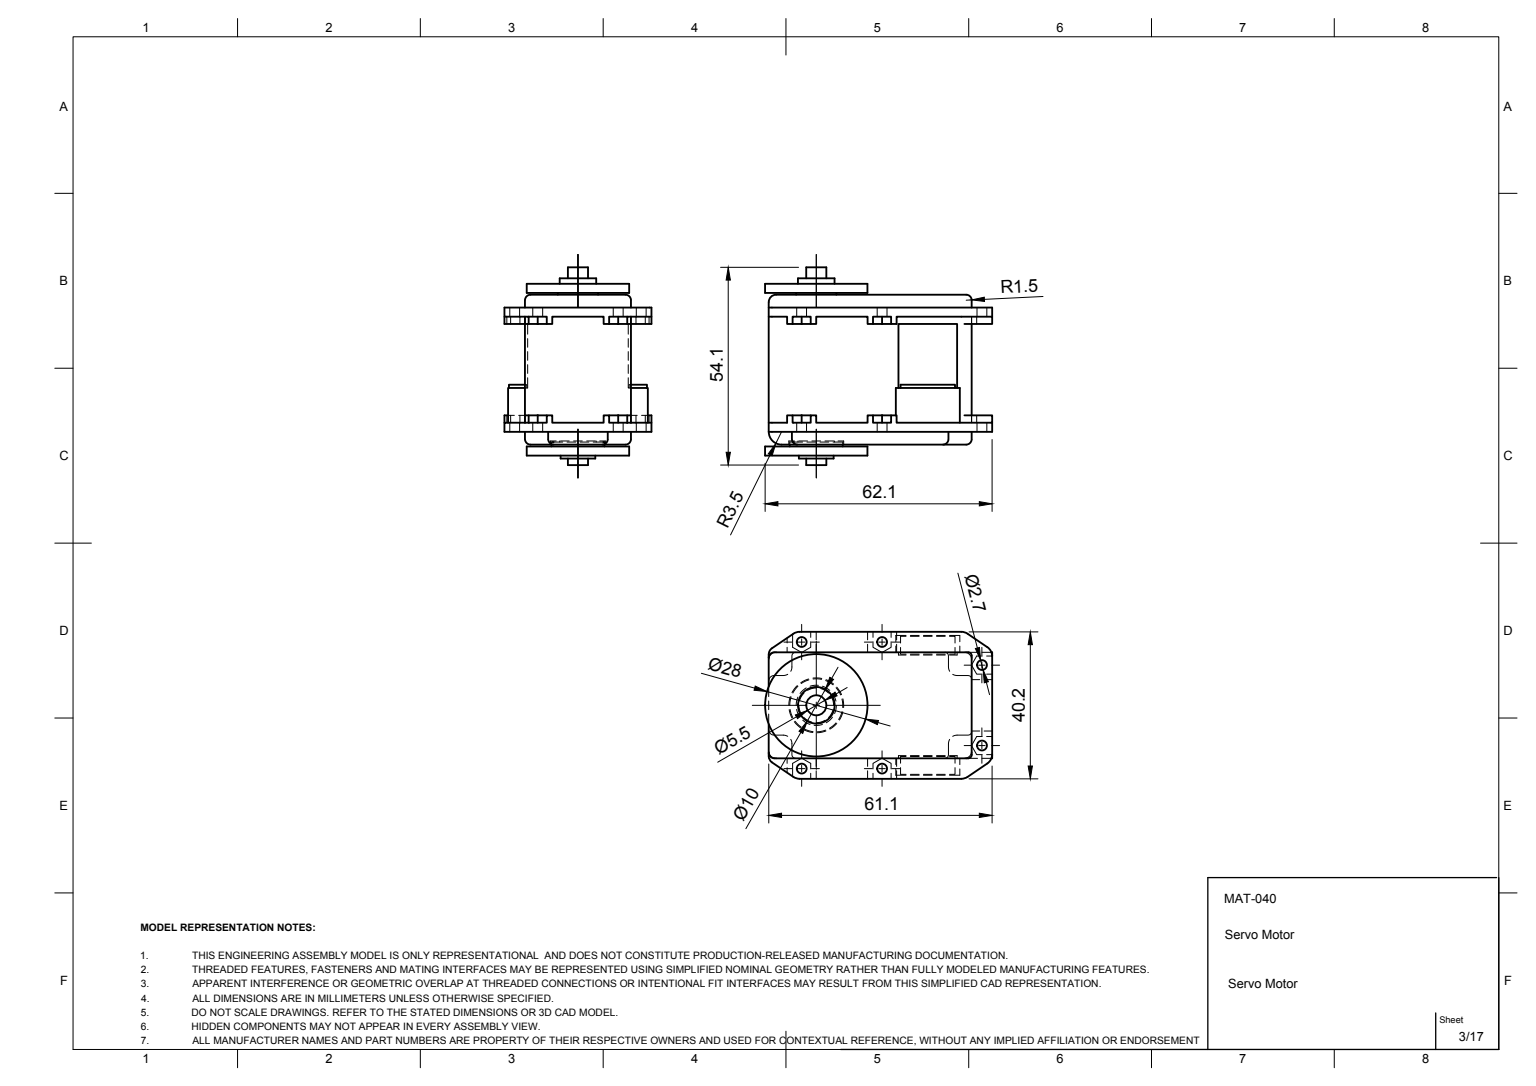
ISO-10303-21;
HEADER;
/* Generated by software containing ST-Developer
 * from STEP Tools, Inc. (www.steptools.com) 
 */

FILE_DESCRIPTION(
/* description */ ('STEP AP214'),
/* implementation_level */ '2;1');

FILE_NAME(
/* name */ 'Servo Motor.step',
/* time_stamp */ '2026-11-14T21:53:28-08:00',
/* author */ (''),
/* organization */ (''),
/* preprocessor_version */ 'ST-DEVELOPER v20.2',
/* originating_system */ 'Autodesk Translation Framework v15.17.0.0',
/* authorisation */ '');

FILE_SCHEMA (('AUTOMOTIVE_DESIGN { 1 0 10303 214 3 1 1 }'));
ENDSEC;

DATA;
#10=MECHANICAL_DESIGN_GEOMETRIC_PRESENTATION_REPRESENTATION('',(#319),#20176);
#223=TOROIDAL_SURFACE('',#11390,2.00000000000006,1.49999999999999);
#224=TOROIDAL_SURFACE('',#11425,1.99999999999991,1.5);
#225=TOROIDAL_SURFACE('',#11523,3.85000000000003,1.50000000000001);
#226=TOROIDAL_SURFACE('',#11533,3.85000000000009,1.50000000000001);
#227=TOROIDAL_SURFACE('',#11543,3.85,1.5);
#228=TOROIDAL_SURFACE('',#11553,3.84999999999996,1.49999999999999);
#232=B_SPLINE_SURFACE_WITH_KNOTS('',3,3,((#16443,#16444,#16445,#16446),
(#16447,#16448,#16449,#16450),(#16451,#16452,#16453,#16454),(#16455,#16456,
#16457,#16458),(#16459,#16460,#16461,#16462),(#16463,#16464,#16465,#16466),
(#16467,#16468,#16469,#16470),(#16471,#16472,#16473,#16474),(#16475,#16476,
#16477,#16478),(#16479,#16480,#16481,#16482),(#16483,#16484,#16485,#16486)),
 .UNSPECIFIED.,.F.,.F.,.F.,(4,1,1,1,1,1,1,1,4),(4,4),(-1.345105E-12,0.125,
0.25,0.375,0.5,0.625,0.75,0.875,0.999999999999432),(-0.007830111379204,
1.00000000177778),.UNSPECIFIED.);
#233=B_SPLINE_SURFACE_WITH_KNOTS('',3,3,((#16489,#16490,#16491,#16492),
(#16493,#16494,#16495,#16496),(#16497,#16498,#16499,#16500),(#16501,#16502,
#16503,#16504),(#16505,#16506,#16507,#16508),(#16509,#16510,#16511,#16512),
(#16513,#16514,#16515,#16516),(#16517,#16518,#16519,#16520),(#16521,#16522,
#16523,#16524),(#16525,#16526,#16527,#16528),(#16529,#16530,#16531,#16532)),
 .UNSPECIFIED.,.F.,.F.,.F.,(4,1,1,1,1,1,1,1,4),(4,4),(-0.000181680414011076,
0.125,0.25,0.375,0.5,0.625,0.75,0.875,1.00018168041298),(-0.007830111378265,
1.00000000177562),.UNSPECIFIED.);
#234=B_SPLINE_SURFACE_WITH_KNOTS('',3,3,((#18463,#18464,#18465,#18466),
(#18467,#18468,#18469,#18470),(#18471,#18472,#18473,#18474),(#18475,#18476,
#18477,#18478),(#18479,#18480,#18481,#18482),(#18483,#18484,#18485,#18486),
(#18487,#18488,#18489,#18490),(#18491,#18492,#18493,#18494),(#18495,#18496,
#18497,#18498),(#18499,#18500,#18501,#18502),(#18503,#18504,#18505,#18506)),
 .UNSPECIFIED.,.F.,.F.,.F.,(4,1,1,1,1,1,1,1,4),(4,4),(-0.000181679232336337,
0.125,0.25,0.375,0.5,0.625,0.75,0.875,1.00018167923146),(-0.007830111378221,
1.00000000177564),.UNSPECIFIED.);
#235=B_SPLINE_SURFACE_WITH_KNOTS('',3,3,((#18507,#18508,#18509,#18510),
(#18511,#18512,#18513,#18514),(#18515,#18516,#18517,#18518),(#18519,#18520,
#18521,#18522),(#18523,#18524,#18525,#18526),(#18527,#18528,#18529,#18530),
(#18531,#18532,#18533,#18534),(#18535,#18536,#18537,#18538),(#18539,#18540,
#18541,#18542),(#18543,#18544,#18545,#18546),(#18547,#18548,#18549,#18550)),
 .UNSPECIFIED.,.F.,.F.,.F.,(4,1,1,1,1,1,1,1,4),(4,4),(-1.346238E-12,0.125,
0.25,0.375,0.5,0.625,0.75,0.875,0.999999999999431),(-0.007830111379204,
1.00000000177778),.UNSPECIFIED.);
#236=B_SPLINE_SURFACE_WITH_KNOTS('',3,3,((#18551,#18552,#18553,#18554),
(#18555,#18556,#18557,#18558),(#18559,#18560,#18561,#18562),(#18563,#18564,
#18565,#18566),(#18567,#18568,#18569,#18570),(#18571,#18572,#18573,#18574),
(#18575,#18576,#18577,#18578),(#18579,#18580,#18581,#18582),(#18583,#18584,
#18585,#18586),(#18587,#18588,#18589,#18590),(#18591,#18592,#18593,#18594)),
 .UNSPECIFIED.,.F.,.F.,.F.,(4,1,1,1,1,1,1,1,4),(4,4),(-1.340881E-12,0.125,
0.25,0.375,0.5,0.625,0.75,0.875,0.999999999999857),(-0.007830111378128,
1.00000000177777),.UNSPECIFIED.);
#237=B_SPLINE_SURFACE_WITH_KNOTS('',3,3,((#18595,#18596,#18597,#18598),
(#18599,#18600,#18601,#18602),(#18603,#18604,#18605,#18606),(#18607,#18608,
#18609,#18610),(#18611,#18612,#18613,#18614),(#18615,#18616,#18617,#18618),
(#18619,#18620,#18621,#18622),(#18623,#18624,#18625,#18626),(#18627,#18628,
#18629,#18630),(#18631,#18632,#18633,#18634),(#18635,#18636,#18637,#18638)),
 .UNSPECIFIED.,.F.,.F.,.F.,(4,1,1,1,1,1,1,1,4),(4,4),(-0.000181679230988105,
0.125,0.25,0.375,0.5,0.625,0.75,0.875,1.00018167923038),(-0.007830111380071,
1.00000000177566),.UNSPECIFIED.);
#238=B_SPLINE_SURFACE_WITH_KNOTS('',3,3,((#18639,#18640,#18641,#18642),
(#18643,#18644,#18645,#18646),(#18647,#18648,#18649,#18650),(#18651,#18652,
#18653,#18654),(#18655,#18656,#18657,#18658),(#18659,#18660,#18661,#18662),
(#18663,#18664,#18665,#18666),(#18667,#18668,#18669,#18670),(#18671,#18672,
#18673,#18674),(#18675,#18676,#18677,#18678),(#18679,#18680,#18681,#18682)),
 .UNSPECIFIED.,.F.,.F.,.F.,(4,1,1,1,1,1,1,1,4),(4,4),(-0.000181679231834029,
0.125,0.25,0.375,0.5,0.625,0.75,0.875,1.0001816792308),(-0.00783011137814,
1.00000000177563),.UNSPECIFIED.);
#239=B_SPLINE_SURFACE_WITH_KNOTS('',3,3,((#18683,#18684,#18685,#18686),
(#18687,#18688,#18689,#18690),(#18691,#18692,#18693,#18694),(#18695,#18696,
#18697,#18698),(#18699,#18700,#18701,#18702),(#18703,#18704,#18705,#18706),
(#18707,#18708,#18709,#18710),(#18711,#18712,#18713,#18714),(#18715,#18716,
#18717,#18718),(#18719,#18720,#18721,#18722),(#18723,#18724,#18725,#18726)),
 .UNSPECIFIED.,.F.,.F.,.F.,(4,1,1,1,1,1,1,1,4),(4,4),(-4.869438E-14,0.125,
0.25,0.375,0.5,0.625,0.75,0.875,0.999999999999432),(-0.007830111379894,
1.00000000177778),.UNSPECIFIED.);
#244=SPHERICAL_SURFACE('',#11302,1.5);
#245=SPHERICAL_SURFACE('',#11304,1.5);
#246=SPHERICAL_SURFACE('',#11635,1.5);
#247=SPHERICAL_SURFACE('',#11636,1.5);
#248=SPHERICAL_SURFACE('',#11637,1.5);
#249=SPHERICAL_SURFACE('',#11638,1.49999999999999);
#250=SPHERICAL_SURFACE('',#11639,1.49999999999999);
#251=SPHERICAL_SURFACE('',#11640,1.50000000000001);
#264=B_SPLINE_CURVE_WITH_KNOTS('',3,(#15932,#15933,#15934,#15935),
 .UNSPECIFIED.,.F.,.F.,(4,4),(0.,1.),.UNSPECIFIED.);
#265=B_SPLINE_CURVE_WITH_KNOTS('',3,(#15937,#15938,#15939,#15940,#15941,
#15942,#15943,#15944,#15945,#15946,#15947,#15948,#15949,#15950,#15951,#15952,
#15953,#15954,#15955,#15956,#15957,#15958,#15959,#15960,#15961,#15962,#15963,
#15964,#15965,#15966,#15967,#15968,#15969,#15970,#15971,#15972,#15973,#15974,
#15975,#15976,#15977,#15978,#15979,#15980,#15981,#15982,#15983,#15984,#15985,
#15986,#15987,#15988,#15989,#15990,#15991,#15992,#15993,#15994,#15995,#15996,
#15997,#15998,#15999,#16000,#16001,#16002,#16003,#16004,#16005,#16006,#16007,
#16008,#16009,#16010,#16011,#16012,#16013,#16014,#16015,#16016,#16017,#16018,
#16019,#16020,#16021,#16022,#16023,#16024,#16025,#16026,#16027,#16028,#16029,
#16030,#16031,#16032,#16033,#16034,#16035,#16036,#16037,#16038,#16039,#16040,
#16041,#16042,#16043,#16044,#16045,#16046,#16047,#16048,#16049,#16050,#16051,
#16052,#16053,#16054,#16055,#16056,#16057,#16058,#16059,#16060,#16061,#16062,
#16063,#16064,#16065,#16066,#16067,#16068,#16069,#16070,#16071,#16072,#16073,
#16074,#16075,#16076,#16077,#16078,#16079,#16080,#16081,#16082,#16083,#16084,
#16085,#16086,#16087,#16088,#16089,#16090,#16091,#16092,#16093,#16094,#16095,
#16096,#16097,#16098,#16099,#16100,#16101,#16102,#16103,#16104,#16105,#16106,
#16107,#16108,#16109,#16110,#16111,#16112,#16113,#16114,#16115,#16116,#16117),
 .UNSPECIFIED.,.F.,.F.,(4,3,3,3,3,3,3,3,3,3,3,3,3,3,3,3,3,3,3,3,3,3,3,3,
3,3,3,3,3,3,3,3,3,3,3,3,3,3,3,3,3,3,3,3,3,3,3,3,3,3,3,3,3,3,3,3,3,3,3,3,
4),(0.,0.0533325059244852,0.0625000000000259,0.0841085084394197,0.105548099870102,
0.125000000000052,0.17630092547594,0.187500000000078,0.218750000000089,
0.234375000000094,0.242187500000095,0.24754815261247,0.250000000000095,
0.287437188888397,0.323763744374451,0.36001030828085,0.393976204362633,
0.427224027426155,0.459537106534552,0.468750000000046,0.484375000000039,
0.492187500000034,0.496093750000031,0.499047272546838,0.500000000000028,
0.531406909119804,0.562578454559912,0.59375000000002,0.605659576286838,
0.617496842340772,0.625000000000018,0.661169076078725,0.687500000000014,
0.71875000000001,0.73437500000001,0.742187500000009,0.750000000000009,0.781516758419965,
0.812499999999997,0.832471681794437,0.852007987221176,0.870840274034354,
0.874999999999985,0.897518269248034,0.906249999999981,0.921874999999979,
0.92968749999998,0.934543491568822,0.93749999999998,0.950765500153561,0.963898282500585,
0.968749999999992,0.97863369201704,0.984374999999997,0.991614704653795,
0.992187500000001,0.994140625,0.995507742631974,0.99609375,0.998075415265071,
1.),.UNSPECIFIED.);
#266=B_SPLINE_CURVE_WITH_KNOTS('',3,(#16122,#16123,#16124,#16125,#16126,
#16127,#16128,#16129,#16130,#16131,#16132,#16133,#16134,#16135,#16136,#16137,
#16138,#16139,#16140,#16141,#16142,#16143,#16144,#16145,#16146,#16147,#16148,
#16149,#16150,#16151,#16152,#16153,#16154,#16155,#16156,#16157,#16158,#16159,
#16160,#16161,#16162,#16163,#16164,#16165,#16166,#16167,#16168,#16169,#16170,
#16171,#16172,#16173),.UNSPECIFIED.,.F.,.F.,(4,3,3,3,3,3,3,3,3,3,3,3,3,
3,3,3,3,4),(0.,0.0745637565188147,0.124999999999995,0.166238958053025,0.208865678848304,
0.249999999999991,0.346113958897021,0.44432471974493,0.499999999999994,
0.562499999999995,0.623864871544663,0.68693243577233,0.744023847861239,
0.749999999999997,0.824321378787994,0.897946690630251,0.96837154638694,
1.),.UNSPECIFIED.);
#267=B_SPLINE_CURVE_WITH_KNOTS('',3,(#16175,#16176,#16177,#16178),
 .UNSPECIFIED.,.F.,.F.,(4,4),(0.,1.),.UNSPECIFIED.);
#268=B_SPLINE_CURVE_WITH_KNOTS('',3,(#16183,#16184,#16185,#16186,#16187,
#16188,#16189,#16190,#16191,#16192,#16193,#16194,#16195,#16196,#16197,#16198,
#16199,#16200,#16201,#16202,#16203,#16204,#16205,#16206,#16207,#16208,#16209,
#16210,#16211,#16212,#16213,#16214,#16215,#16216,#16217,#16218,#16219,#16220,
#16221,#16222,#16223,#16224,#16225,#16226,#16227,#16228,#16229,#16230,#16231,
#16232,#16233,#16234,#16235,#16236),.UNSPECIFIED.,.F.,.F.,(4,2,2,2,1,1,
2,2,2,2,2,2,2,2,2,2,1,1,2,2,2,2,2,2,2,2,2,2,4),(0.,0.0625000000000705,0.0937500000001039,
0.109375000000121,0.117187500000129,0.121093750000133,0.123046875000136,
0.125000000000139,0.187500000000148,0.218750000000152,0.250000000000156,
0.312500000000164,0.343750000000167,0.37500000000017,0.437500000000176,
0.468750000000182,0.484375000000184,0.492187500000182,0.496093750000183,
0.500000000000184,0.625000000000146,0.687500000000124,0.718750000000111,
0.734375000000106,0.7500000000001,0.812500000000071,0.84375000000006,0.875000000000048,
1.),.UNSPECIFIED.);
#269=B_SPLINE_CURVE_WITH_KNOTS('',3,(#16244,#16245,#16246,#16247,#16248,
#16249,#16250,#16251,#16252,#16253,#16254,#16255,#16256,#16257,#16258,#16259,
#16260,#16261,#16262,#16263,#16264,#16265,#16266,#16267,#16268,#16269,#16270,
#16271,#16272,#16273,#16274,#16275,#16276,#16277,#16278,#16279,#16280,#16281,
#16282,#16283,#16284,#16285,#16286,#16287,#16288,#16289,#16290,#16291,#16292,
#16293,#16294,#16295),.UNSPECIFIED.,.F.,.F.,(4,3,3,3,3,3,3,3,3,3,3,3,3,
3,3,3,3,4),(0.,0.0745637565509513,0.125,0.166238958062739,0.208865678867621,
0.25,0.346113958735942,0.444324719419348,0.5,0.5625,0.623864871537258,0.686932435768629,
0.74402384785074,0.75,0.824321356610985,0.897946645963302,0.968371480101265,
0.999999995426981),.UNSPECIFIED.);
#270=B_SPLINE_CURVE_WITH_KNOTS('',3,(#16770,#16771,#16772,#16773),
 .UNSPECIFIED.,.F.,.F.,(4,4),(0.,1.),.UNSPECIFIED.);
#271=B_SPLINE_CURVE_WITH_KNOTS('',3,(#16782,#16783,#16784,#16785),
 .UNSPECIFIED.,.F.,.F.,(4,4),(0.,1.),.UNSPECIFIED.);
#272=B_SPLINE_CURVE_WITH_KNOTS('',3,(#16789,#16790,#16791,#16792),
 .UNSPECIFIED.,.F.,.F.,(4,4),(0.,1.),.UNSPECIFIED.);
#273=B_SPLINE_CURVE_WITH_KNOTS('',3,(#16802,#16803,#16804,#16805),
 .UNSPECIFIED.,.F.,.F.,(4,4),(0.,1.),.UNSPECIFIED.);
#274=B_SPLINE_CURVE_WITH_KNOTS('',3,(#16814,#16815,#16816,#16817),
 .UNSPECIFIED.,.F.,.F.,(4,4),(0.,1.),.UNSPECIFIED.);
#275=B_SPLINE_CURVE_WITH_KNOTS('',3,(#16826,#16827,#16828,#16829),
 .UNSPECIFIED.,.F.,.F.,(4,4),(0.,1.),.UNSPECIFIED.);
#276=B_SPLINE_CURVE_WITH_KNOTS('',3,(#16833,#16834,#16835,#16836),
 .UNSPECIFIED.,.F.,.F.,(4,4),(0.,1.),.UNSPECIFIED.);
#277=B_SPLINE_CURVE_WITH_KNOTS('',3,(#16846,#16847,#16848,#16849),
 .UNSPECIFIED.,.F.,.F.,(4,4),(0.,1.),.UNSPECIFIED.);
#278=B_SPLINE_CURVE_WITH_KNOTS('',3,(#16858,#16859,#16860,#16861),
 .UNSPECIFIED.,.F.,.F.,(4,4),(0.,1.),.UNSPECIFIED.);
#279=B_SPLINE_CURVE_WITH_KNOTS('',3,(#16870,#16871,#16872,#16873),
 .UNSPECIFIED.,.F.,.F.,(4,4),(0.,1.),.UNSPECIFIED.);
#280=B_SPLINE_CURVE_WITH_KNOTS('',3,(#16877,#16878,#16879,#16880),
 .UNSPECIFIED.,.F.,.F.,(4,4),(0.,1.),.UNSPECIFIED.);
#281=B_SPLINE_CURVE_WITH_KNOTS('',3,(#16890,#16891,#16892,#16893),
 .UNSPECIFIED.,.F.,.F.,(4,4),(0.,1.),.UNSPECIFIED.);
#282=B_SPLINE_CURVE_WITH_KNOTS('',3,(#17701,#17702,#17703,#17704,#17705,
#17706,#17707,#17708,#17709,#17710,#17711,#17712,#17713,#17714,#17715,#17716,
#17717,#17718,#17719,#17720,#17721,#17722,#17723,#17724,#17725,#17726,#17727,
#17728,#17729,#17730,#17731,#17732,#17733,#17734,#17735,#17736,#17737,#17738,
#17739,#17740,#17741,#17742,#17743,#17744,#17745,#17746,#17747,#17748,#17749,
#17750,#17751,#17752,#17753,#17754),.UNSPECIFIED.,.F.,.F.,(4,2,2,2,1,1,
2,2,2,2,2,2,2,2,2,2,1,1,2,2,2,2,2,2,2,2,2,2,4),(0.,0.0624999999999807,0.093749999999971,
0.109374999999966,0.117187499999965,0.121093749999965,0.123046874999964,
0.124999999999963,0.187499999999964,0.218749999999966,0.249999999999968,
0.312499999999973,0.343749999999976,0.37499999999998,0.437499999999987,
0.468749999999992,0.484374999999994,0.492187499999996,0.496093749999996,
0.499999999999996,0.625000000000009,0.687500000000016,0.718750000000018,
0.734375000000018,0.750000000000018,0.812500000000013,0.843750000000011,
0.875000000000008,1.),.UNSPECIFIED.);
#283=B_SPLINE_CURVE_WITH_KNOTS('',3,(#17756,#17757,#17758,#17759,#17760,
#17761,#17762,#17763,#17764,#17765,#17766,#17767,#17768,#17769,#17770,#17771,
#17772,#17773,#17774,#17775,#17776,#17777,#17778,#17779,#17780,#17781,#17782,
#17783,#17784,#17785,#17786,#17787,#17788,#17789,#17790,#17791,#17792,#17793,
#17794,#17795,#17796,#17797,#17798,#17799,#17800,#17801,#17802,#17803,#17804,
#17805,#17806,#17807,#17808,#17809,#17810,#17811,#17812,#17813,#17814,#17815,
#17816,#17817,#17818,#17819,#17820,#17821,#17822,#17823,#17824,#17825,#17826,
#17827,#17828,#17829,#17830,#17831,#17832,#17833,#17834,#17835,#17836,#17837,
#17838,#17839,#17840,#17841,#17842,#17843,#17844,#17845,#17846,#17847,#17848,
#17849,#17850,#17851,#17852,#17853,#17854,#17855,#17856,#17857,#17858,#17859,
#17860,#17861,#17862,#17863,#17864,#17865,#17866,#17867,#17868,#17869,#17870,
#17871,#17872,#17873,#17874,#17875,#17876,#17877,#17878,#17879,#17880,#17881,
#17882,#17883,#17884,#17885,#17886,#17887,#17888,#17889,#17890,#17891,#17892,
#17893,#17894,#17895,#17896,#17897,#17898,#17899,#17900,#17901,#17902,#17903,
#17904,#17905,#17906,#17907,#17908,#17909,#17910,#17911,#17912,#17913,#17914,
#17915,#17916,#17917,#17918,#17919,#17920,#17921,#17922,#17923,#17924,#17925,
#17926,#17927,#17928,#17929,#17930,#17931,#17932,#17933,#17934,#17935,#17936),
 .UNSPECIFIED.,.F.,.F.,(4,3,3,3,3,3,3,3,3,3,3,3,3,3,3,3,3,3,3,3,3,3,3,3,
3,3,3,3,3,3,3,3,3,3,3,3,3,3,3,3,3,3,3,3,3,3,3,3,3,3,3,3,3,3,3,3,3,3,3,3,
4),(0.,0.0533325059154056,0.062500000000017,0.0841085084223245,0.105548099835893,
0.125000000000034,0.17630092547998,0.187500000000051,0.21875000000006,0.234375000000064,
0.242187500000064,0.2475481526123,0.250000000000065,0.287437188884715,0.323763744367256,
0.360010308275466,0.393976204354617,0.427224027414522,0.45953710653336,
0.468750000000096,0.484375000000098,0.492187500000099,0.496093750000102,
0.499047272544739,0.500000000000104,0.531406909072734,0.56257845453641,
0.593750000000087,0.605659576246251,0.617496842260655,0.625000000000081,
0.661169076083868,0.687500000000069,0.718750000000065,0.734375000000062,
0.742187500000061,0.750000000000059,0.781516758434333,0.812500000000044,
0.832471682711535,0.852007989016106,0.870840276699918,0.875000000000029,
0.897518269572018,0.906250000000022,0.921875000000018,0.929687500000018,
0.934543491257381,0.937500000000019,0.950765546817596,0.963898373867096,
0.968750000000011,0.978633754201887,0.984375000000007,0.991614644761784,
0.992187500000004,0.994140625000003,0.995507742863477,0.996093750000002,
0.998075415535184,1.),.UNSPECIFIED.);
#284=B_SPLINE_CURVE_WITH_KNOTS('',3,(#17938,#17939,#17940,#17941,#17942,
#17943,#17944,#17945,#17946,#17947,#17948,#17949,#17950,#17951,#17952,#17953,
#17954,#17955,#17956,#17957,#17958,#17959,#17960,#17961,#17962,#17963,#17964,
#17965,#17966,#17967,#17968,#17969,#17970,#17971,#17972,#17973,#17974,#17975,
#17976,#17977,#17978,#17979,#17980,#17981,#17982,#17983,#17984,#17985,#17986,
#17987,#17988,#17989,#17990,#17991,#17992,#17993,#17994,#17995,#17996,#17997,
#17998,#17999,#18000,#18001,#18002,#18003,#18004,#18005,#18006,#18007,#18008,
#18009,#18010,#18011,#18012,#18013,#18014,#18015,#18016,#18017,#18018,#18019,
#18020,#18021,#18022,#18023,#18024,#18025,#18026,#18027,#18028,#18029,#18030,
#18031,#18032,#18033,#18034,#18035,#18036,#18037,#18038,#18039,#18040,#18041,
#18042,#18043,#18044,#18045,#18046,#18047,#18048,#18049,#18050,#18051,#18052,
#18053,#18054,#18055,#18056,#18057,#18058,#18059,#18060,#18061,#18062,#18063,
#18064,#18065,#18066,#18067,#18068,#18069,#18070,#18071,#18072,#18073,#18074,
#18075,#18076,#18077,#18078,#18079,#18080,#18081,#18082,#18083,#18084,#18085,
#18086,#18087,#18088,#18089,#18090,#18091,#18092,#18093,#18094,#18095,#18096,
#18097,#18098,#18099,#18100,#18101,#18102,#18103,#18104,#18105,#18106,#18107,
#18108,#18109,#18110,#18111,#18112,#18113,#18114,#18115,#18116,#18117,#18118),
 .UNSPECIFIED.,.F.,.F.,(4,3,3,3,3,3,3,3,3,3,3,3,3,3,3,3,3,3,3,3,3,3,3,3,
3,3,3,3,3,3,3,3,3,3,3,3,3,3,3,3,3,3,3,3,3,3,3,3,3,3,3,3,3,3,3,3,3,3,3,3,
4),(0.,0.053332505916002,0.0625000000000664,0.0841085085020462,0.105548099995911,
0.125000000000133,0.176300925460898,0.187500000000199,0.218750000000231,
0.234375000000248,0.242187500000256,0.247548152608829,0.250000000000264,
0.287437188887554,0.323763744372456,0.360010308279463,0.393976204361919,
0.427224027424111,0.459537106542875,0.468750000000484,0.484375000000498,
0.492187500000504,0.496093750000504,0.499047272547063,0.500000000000505,
0.531250000000472,0.562500000000438,0.593750000000407,0.605659576239387,
0.617496842248128,0.625000000000376,0.661011309028678,0.697853969089471,
0.718750000000282,0.734375000000266,0.742187500000258,0.750000000000251,
0.781516758445273,0.812500000000191,0.832471681935561,0.85200798749801,
0.870840274446439,0.875000000000132,0.897518269314931,0.906250000000102,
0.921875000000087,0.92968750000008,0.934543491553856,0.937500000000074,
0.950765490114461,0.963898262934216,0.96875000000004,0.978633529008707,
0.984375000000022,0.991614027021566,0.992187500000011,0.994140625000009,
0.995507744224286,0.996093750000006,0.998075415565434,1.),.UNSPECIFIED.);
#285=B_SPLINE_CURVE_WITH_KNOTS('',3,(#18120,#18121,#18122,#18123,#18124,
#18125,#18126,#18127,#18128,#18129,#18130,#18131,#18132,#18133,#18134,#18135,
#18136,#18137,#18138,#18139,#18140,#18141,#18142,#18143,#18144,#18145,#18146,
#18147,#18148,#18149,#18150,#18151,#18152,#18153,#18154,#18155,#18156,#18157,
#18158,#18159,#18160,#18161,#18162,#18163,#18164,#18165,#18166,#18167,#18168,
#18169,#18170,#18171,#18172,#18173),.UNSPECIFIED.,.F.,.F.,(4,2,2,2,1,1,
2,2,2,2,2,2,2,2,2,2,1,1,2,2,2,2,2,2,2,2,2,2,4),(0.,0.0625000000000238,0.0937500000000341,
0.109375000000038,0.11718750000004,0.12109375000004,0.123046875000041,0.125000000000041,
0.187500000000023,0.218750000000015,0.250000000000006,0.312499999999989,
0.343749999999983,0.374999999999977,0.437499999999965,0.468749999999959,
0.484374999999956,0.492187499999955,0.496093749999954,0.499999999999953,
0.624999999999966,0.687499999999976,0.71874999999998,0.734374999999982,
0.749999999999985,0.812499999999992,0.843749999999994,0.874999999999997,
1.),.UNSPECIFIED.);
#286=B_SPLINE_CURVE_WITH_KNOTS('',3,(#18175,#18176,#18177,#18178,#18179,
#18180,#18181,#18182,#18183,#18184,#18185,#18186,#18187,#18188,#18189,#18190,
#18191,#18192,#18193,#18194,#18195,#18196,#18197,#18198,#18199,#18200,#18201,
#18202,#18203,#18204,#18205,#18206,#18207,#18208,#18209,#18210,#18211,#18212,
#18213,#18214,#18215,#18216,#18217,#18218,#18219,#18220,#18221,#18222,#18223,
#18224,#18225,#18226,#18227,#18228),.UNSPECIFIED.,.F.,.F.,(4,2,2,2,1,1,
2,2,2,2,2,2,2,2,2,2,1,1,2,2,2,2,2,2,2,2,2,2,4),(0.,0.0625000000000846,0.093750000000127,
0.109375000000148,0.117187500000158,0.121093750000162,0.123046875000163,
0.125000000000164,0.187500000000187,0.2187500000002,0.250000000000213,0.312500000000245,
0.343750000000259,0.375000000000273,0.437500000000297,0.468750000000308,
0.484375000000314,0.492187500000316,0.496093750000316,0.500000000000315,
0.625000000000258,0.687500000000227,0.718750000000211,0.734375000000202,
0.750000000000193,0.812500000000147,0.843750000000123,0.875000000000099,
1.),.UNSPECIFIED.);
#287=B_SPLINE_CURVE_WITH_KNOTS('',3,(#18230,#18231,#18232,#18233,#18234,
#18235,#18236,#18237,#18238,#18239,#18240,#18241,#18242,#18243,#18244,#18245,
#18246,#18247,#18248,#18249,#18250,#18251,#18252,#18253,#18254,#18255,#18256,
#18257,#18258,#18259,#18260,#18261,#18262,#18263,#18264,#18265,#18266,#18267,
#18268,#18269,#18270,#18271,#18272,#18273,#18274,#18275,#18276,#18277,#18278,
#18279,#18280,#18281,#18282,#18283,#18284,#18285,#18286,#18287,#18288,#18289,
#18290,#18291,#18292,#18293,#18294,#18295,#18296,#18297,#18298,#18299,#18300,
#18301,#18302,#18303,#18304,#18305,#18306,#18307,#18308,#18309,#18310,#18311,
#18312,#18313,#18314,#18315,#18316,#18317,#18318,#18319,#18320,#18321,#18322,
#18323,#18324,#18325,#18326,#18327,#18328,#18329,#18330,#18331,#18332,#18333,
#18334,#18335,#18336,#18337,#18338,#18339,#18340,#18341,#18342,#18343,#18344,
#18345,#18346,#18347,#18348,#18349,#18350,#18351,#18352,#18353,#18354,#18355,
#18356,#18357,#18358,#18359,#18360,#18361,#18362,#18363,#18364,#18365,#18366,
#18367,#18368,#18369,#18370,#18371,#18372,#18373,#18374,#18375,#18376,#18377,
#18378,#18379,#18380,#18381,#18382,#18383,#18384,#18385,#18386,#18387,#18388,
#18389,#18390,#18391,#18392,#18393,#18394,#18395,#18396,#18397,#18398,#18399,
#18400,#18401,#18402,#18403,#18404,#18405,#18406,#18407,#18408,#18409,#18410),
 .UNSPECIFIED.,.F.,.F.,(4,3,3,3,3,3,3,3,3,3,3,3,3,3,3,3,3,3,3,3,3,3,3,3,
3,3,3,3,3,3,3,3,3,3,3,3,3,3,3,3,3,3,3,3,3,3,3,3,3,3,3,3,3,3,3,3,3,3,3,3,
4),(0.,0.05335209394236,0.062500000000007,0.0841472767069337,0.105624836390271,
0.125000000000014,0.176300925463353,0.187500000000021,0.218750000000026,
0.234375000000029,0.24218750000003,0.247548152609244,0.250000000000031,
0.287437188886521,0.323763744370703,0.360010308278026,0.393976204358943,
0.427224027420569,0.459537106532236,0.468749999999997,0.484374999999994,
0.492187499999994,0.496093749999994,0.499047272546512,0.499999999999994,
0.531406909114999,0.562578454557502,0.593750000000005,0.605659576241387,
0.617496842252372,0.625000000000008,0.661011309019872,0.69785396907197,
0.718750000000017,0.734375000000017,0.742187500000017,0.750000000000017,
0.781516758358948,0.812500000000015,0.83247168165504,0.852007986946234,
0.870840273623334,0.875000000000014,0.897518269153575,0.906250000000012,
0.921875000000012,0.929687500000011,0.934543491364392,0.937500000000009,
0.950765509160406,0.963898300247594,0.968750000000007,0.978633643598403,
0.984375000000004,0.991614445716802,0.992187500000004,0.994140625000004,
0.995507743246036,0.996093750000003,0.998075415497727,1.),.UNSPECIFIED.);
#292=(
BOUNDED_SURFACE()
B_SPLINE_SURFACE(2,2,((#15889,#15890,#15891),(#15892,#15893,#15894),(#15895,
#15896,#15897),(#15898,#15899,#15900),(#15901,#15902,#15903)),
 .UNSPECIFIED.,.F.,.F.,.F.)
B_SPLINE_SURFACE_WITH_KNOTS((3,2,3),(3,3),(-1.57079650760589,-0.785398253794349,
1.7193274521714E-11),(-6.45261621924302E-12,1.57079632720499),
 .UNSPECIFIED.)
GEOMETRIC_REPRESENTATION_ITEM()
RATIONAL_B_SPLINE_SURFACE(((1.,0.707106781039276,1.),(0.923879515211315,
0.6532814700692,0.923879515211315),(1.,0.707106781039276,1.),(0.923879515211332,
0.653281470069212,0.923879515211332),(1.,0.707106781039276,1.)))
REPRESENTATION_ITEM('')
SURFACE()
);
#293=(
BOUNDED_SURFACE()
B_SPLINE_SURFACE(2,2,((#15907,#15908,#15909),(#15910,#15911,#15912),(#15913,
#15914,#15915),(#15916,#15917,#15918),(#15919,#15920,#15921)),
 .UNSPECIFIED.,.F.,.F.,.F.)
B_SPLINE_SURFACE_WITH_KNOTS((3,2,3),(3,3),(-1.21879451958182E-11,0.785398208598734,
1.57079641720966),(-1.18060512023842E-11,1.57079632732992),
 .UNSPECIFIED.)
GEOMETRIC_REPRESENTATION_ITEM()
RATIONAL_B_SPLINE_SURFACE(((1.,0.707106780993216,1.),(0.923879523860082,
0.653281476142247,0.923879523860082),(1.,0.707106780993216,1.),(0.923879523860064,
0.653281476142235,0.923879523860064),(1.,0.707106780993216,1.)))
REPRESENTATION_ITEM('')
SURFACE()
);
#295=SHAPE_REPRESENTATION_RELATIONSHIP('SRR','None',#20257,#307);
#307=ADVANCED_BREP_SHAPE_REPRESENTATION('',(#354),#20163);
#319=STYLED_ITEM('',(#20336),#354);
#354=MANIFOLD_SOLID_BREP('Body1',#10945);
#414=FACE_BOUND('',#1600,.T.);
#415=FACE_BOUND('',#1606,.T.);
#416=FACE_BOUND('',#1619,.T.);
#417=FACE_BOUND('',#1620,.T.);
#418=FACE_BOUND('',#1621,.T.);
#419=FACE_BOUND('',#1622,.T.);
#420=FACE_BOUND('',#1623,.T.);
#421=FACE_BOUND('',#1624,.T.);
#422=FACE_BOUND('',#1632,.T.);
#423=FACE_BOUND('',#1633,.T.);
#424=FACE_BOUND('',#1634,.T.);
#425=FACE_BOUND('',#1635,.T.);
#426=FACE_BOUND('',#1636,.T.);
#427=FACE_BOUND('',#1637,.T.);
#428=FACE_BOUND('',#1643,.T.);
#429=FACE_BOUND('',#1685,.T.);
#430=FACE_BOUND('',#1739,.T.);
#431=FACE_BOUND('',#1741,.T.);
#432=FACE_BOUND('',#1743,.T.);
#433=FACE_BOUND('',#1745,.T.);
#434=FACE_BOUND('',#1747,.T.);
#435=FACE_BOUND('',#1749,.T.);
#436=FACE_BOUND('',#1816,.T.);
#437=FACE_BOUND('',#1818,.T.);
#438=FACE_BOUND('',#1820,.T.);
#439=FACE_BOUND('',#1822,.T.);
#440=FACE_BOUND('',#1824,.T.);
#441=FACE_BOUND('',#1826,.T.);
#442=FACE_BOUND('',#1839,.T.);
#443=FACE_BOUND('',#1848,.T.);
#444=FACE_BOUND('',#1875,.T.);
#445=FACE_BOUND('',#1881,.T.);
#446=FACE_BOUND('',#1910,.T.);
#447=FACE_BOUND('',#1913,.T.);
#448=FACE_BOUND('',#1915,.T.);
#449=FACE_BOUND('',#1917,.T.);
#598=PLANE('',#11282);
#599=PLANE('',#11295);
#600=PLANE('',#11296);
#601=PLANE('',#11301);
#602=PLANE('',#11303);
#603=PLANE('',#11305);
#604=PLANE('',#11315);
#605=PLANE('',#11350);
#606=PLANE('',#11363);
#607=PLANE('',#11364);
#608=PLANE('',#11365);
#609=PLANE('',#11366);
#610=PLANE('',#11367);
#611=PLANE('',#11368);
#612=PLANE('',#11371);
#613=PLANE('',#11374);
#614=PLANE('',#11379);
#615=PLANE('',#11384);
#616=PLANE('',#11387);
#617=PLANE('',#11393);
#618=PLANE('',#11396);
#619=PLANE('',#11399);
#620=PLANE('',#11402);
#621=PLANE('',#11405);
#622=PLANE('',#11408);
#623=PLANE('',#11411);
#624=PLANE('',#11414);
#625=PLANE('',#11417);
#626=PLANE('',#11420);
#627=PLANE('',#11423);
#628=PLANE('',#11427);
#629=PLANE('',#11428);
#630=PLANE('',#11433);
#631=PLANE('',#11434);
#632=PLANE('',#11435);
#633=PLANE('',#11436);
#634=PLANE('',#11437);
#635=PLANE('',#11440);
#636=PLANE('',#11445);
#637=PLANE('',#11450);
#638=PLANE('',#11453);
#639=PLANE('',#11458);
#640=PLANE('',#11459);
#641=PLANE('',#11460);
#642=PLANE('',#11461);
#643=PLANE('',#11462);
#644=PLANE('',#11466);
#645=PLANE('',#11467);
#646=PLANE('',#11468);
#647=PLANE('',#11469);
#648=PLANE('',#11470);
#649=PLANE('',#11471);
#650=PLANE('',#11472);
#651=PLANE('',#11473);
#652=PLANE('',#11474);
#653=PLANE('',#11475);
#654=PLANE('',#11476);
#655=PLANE('',#11477);
#656=PLANE('',#11478);
#657=PLANE('',#11479);
#658=PLANE('',#11480);
#659=PLANE('',#11481);
#660=PLANE('',#11482);
#661=PLANE('',#11483);
#662=PLANE('',#11484);
#663=PLANE('',#11485);
#664=PLANE('',#11486);
#665=PLANE('',#11487);
#666=PLANE('',#11488);
#667=PLANE('',#11489);
#668=PLANE('',#11490);
#669=PLANE('',#11491);
#670=PLANE('',#11492);
#671=PLANE('',#11493);
#672=PLANE('',#11494);
#673=PLANE('',#11495);
#674=PLANE('',#11496);
#675=PLANE('',#11497);
#676=PLANE('',#11498);
#677=PLANE('',#11499);
#678=PLANE('',#11500);
#679=PLANE('',#11501);
#680=PLANE('',#11502);
#681=PLANE('',#11503);
#682=PLANE('',#11504);
#683=PLANE('',#11505);
#684=PLANE('',#11506);
#685=PLANE('',#11507);
#686=PLANE('',#11508);
#687=PLANE('',#11509);
#688=PLANE('',#11510);
#689=PLANE('',#11511);
#690=PLANE('',#11512);
#691=PLANE('',#11513);
#692=PLANE('',#11514);
#693=PLANE('',#11515);
#694=PLANE('',#11516);
#695=PLANE('',#11517);
#696=PLANE('',#11518);
#697=PLANE('',#11519);
#698=PLANE('',#11520);
#699=PLANE('',#11556);
#700=PLANE('',#11557);
#701=PLANE('',#11558);
#702=PLANE('',#11559);
#703=PLANE('',#11560);
#704=PLANE('',#11561);
#705=PLANE('',#11562);
#706=PLANE('',#11563);
#707=PLANE('',#11564);
#708=PLANE('',#11565);
#709=PLANE('',#11566);
#710=PLANE('',#11567);
#711=PLANE('',#11568);
#712=PLANE('',#11569);
#713=PLANE('',#11570);
#714=PLANE('',#11571);
#715=PLANE('',#11572);
#716=PLANE('',#11573);
#717=PLANE('',#11574);
#718=PLANE('',#11575);
#719=PLANE('',#11576);
#720=PLANE('',#11577);
#721=PLANE('',#11578);
#722=PLANE('',#11579);
#723=PLANE('',#11580);
#724=PLANE('',#11581);
#725=PLANE('',#11582);
#726=PLANE('',#11586);
#727=PLANE('',#11587);
#728=PLANE('',#11588);
#729=PLANE('',#11589);
#730=PLANE('',#11590);
#731=PLANE('',#11591);
#732=PLANE('',#11592);
#733=PLANE('',#11593);
#734=PLANE('',#11594);
#735=PLANE('',#11595);
#736=PLANE('',#11596);
#737=PLANE('',#11597);
#738=PLANE('',#11598);
#739=PLANE('',#11599);
#740=PLANE('',#11600);
#741=PLANE('',#11601);
#742=PLANE('',#11602);
#743=PLANE('',#11603);
#744=PLANE('',#11604);
#745=PLANE('',#11605);
#746=PLANE('',#11606);
#747=PLANE('',#11607);
#748=PLANE('',#11608);
#749=PLANE('',#11609);
#750=PLANE('',#11610);
#751=PLANE('',#11611);
#752=PLANE('',#11612);
#753=PLANE('',#11613);
#754=PLANE('',#11614);
#755=PLANE('',#11615);
#756=PLANE('',#11616);
#757=PLANE('',#11617);
#758=PLANE('',#11618);
#759=PLANE('',#11619);
#760=PLANE('',#11620);
#761=PLANE('',#11621);
#762=PLANE('',#11622);
#763=PLANE('',#11623);
#764=PLANE('',#11624);
#765=PLANE('',#11625);
#766=PLANE('',#11626);
#767=PLANE('',#11627);
#768=PLANE('',#11628);
#769=PLANE('',#11629);
#770=PLANE('',#11630);
#771=PLANE('',#11631);
#772=PLANE('',#11632);
#773=PLANE('',#11633);
#774=PLANE('',#11634);
#775=PLANE('',#11641);
#776=PLANE('',#11642);
#777=PLANE('',#11643);
#778=PLANE('',#11644);
#779=PLANE('',#11645);
#780=PLANE('',#11646);
#781=PLANE('',#11647);
#782=PLANE('',#11648);
#783=PLANE('',#11649);
#784=PLANE('',#11650);
#785=PLANE('',#11651);
#786=PLANE('',#11652);
#787=PLANE('',#11653);
#788=PLANE('',#11654);
#789=PLANE('',#11655);
#790=PLANE('',#11656);
#791=PLANE('',#11657);
#792=PLANE('',#11658);
#793=PLANE('',#11659);
#794=PLANE('',#11660);
#795=PLANE('',#11661);
#796=PLANE('',#11662);
#797=PLANE('',#11663);
#798=PLANE('',#11664);
#799=PLANE('',#11665);
#800=PLANE('',#11666);
#801=PLANE('',#11667);
#802=PLANE('',#11668);
#803=PLANE('',#11669);
#804=PLANE('',#11670);
#805=PLANE('',#11671);
#806=PLANE('',#11672);
#807=PLANE('',#11673);
#951=FACE_OUTER_BOUND('',#1577,.T.);
#952=FACE_OUTER_BOUND('',#1578,.T.);
#953=FACE_OUTER_BOUND('',#1579,.T.);
#954=FACE_OUTER_BOUND('',#1580,.T.);
#955=FACE_OUTER_BOUND('',#1581,.T.);
#956=FACE_OUTER_BOUND('',#1582,.T.);
#957=FACE_OUTER_BOUND('',#1583,.T.);
#958=FACE_OUTER_BOUND('',#1584,.T.);
#959=FACE_OUTER_BOUND('',#1585,.T.);
#960=FACE_OUTER_BOUND('',#1586,.T.);
#961=FACE_OUTER_BOUND('',#1587,.T.);
#962=FACE_OUTER_BOUND('',#1588,.T.);
#963=FACE_OUTER_BOUND('',#1589,.T.);
#964=FACE_OUTER_BOUND('',#1590,.T.);
#965=FACE_OUTER_BOUND('',#1591,.T.);
#966=FACE_OUTER_BOUND('',#1592,.T.);
#967=FACE_OUTER_BOUND('',#1593,.T.);
#968=FACE_OUTER_BOUND('',#1594,.T.);
#969=FACE_OUTER_BOUND('',#1595,.T.);
#970=FACE_OUTER_BOUND('',#1596,.T.);
#971=FACE_OUTER_BOUND('',#1597,.T.);
#972=FACE_OUTER_BOUND('',#1598,.T.);
#973=FACE_OUTER_BOUND('',#1599,.T.);
#974=FACE_OUTER_BOUND('',#1601,.T.);
#975=FACE_OUTER_BOUND('',#1602,.T.);
#976=FACE_OUTER_BOUND('',#1603,.T.);
#977=FACE_OUTER_BOUND('',#1604,.T.);
#978=FACE_OUTER_BOUND('',#1605,.T.);
#979=FACE_OUTER_BOUND('',#1607,.T.);
#980=FACE_OUTER_BOUND('',#1608,.T.);
#981=FACE_OUTER_BOUND('',#1609,.T.);
#982=FACE_OUTER_BOUND('',#1610,.T.);
#983=FACE_OUTER_BOUND('',#1611,.T.);
#984=FACE_OUTER_BOUND('',#1612,.T.);
#985=FACE_OUTER_BOUND('',#1613,.T.);
#986=FACE_OUTER_BOUND('',#1614,.T.);
#987=FACE_OUTER_BOUND('',#1615,.T.);
#988=FACE_OUTER_BOUND('',#1616,.T.);
#989=FACE_OUTER_BOUND('',#1617,.T.);
#990=FACE_OUTER_BOUND('',#1618,.T.);
#991=FACE_OUTER_BOUND('',#1625,.T.);
#992=FACE_OUTER_BOUND('',#1626,.T.);
#993=FACE_OUTER_BOUND('',#1627,.T.);
#994=FACE_OUTER_BOUND('',#1628,.T.);
#995=FACE_OUTER_BOUND('',#1629,.T.);
#996=FACE_OUTER_BOUND('',#1630,.T.);
#997=FACE_OUTER_BOUND('',#1631,.T.);
#998=FACE_OUTER_BOUND('',#1638,.T.);
#999=FACE_OUTER_BOUND('',#1639,.T.);
#1000=FACE_OUTER_BOUND('',#1640,.T.);
#1001=FACE_OUTER_BOUND('',#1641,.T.);
#1002=FACE_OUTER_BOUND('',#1642,.T.);
#1003=FACE_OUTER_BOUND('',#1644,.T.);
#1004=FACE_OUTER_BOUND('',#1645,.T.);
#1005=FACE_OUTER_BOUND('',#1646,.T.);
#1006=FACE_OUTER_BOUND('',#1647,.T.);
#1007=FACE_OUTER_BOUND('',#1648,.T.);
#1008=FACE_OUTER_BOUND('',#1649,.T.);
#1009=FACE_OUTER_BOUND('',#1650,.T.);
#1010=FACE_OUTER_BOUND('',#1651,.T.);
#1011=FACE_OUTER_BOUND('',#1652,.T.);
#1012=FACE_OUTER_BOUND('',#1653,.T.);
#1013=FACE_OUTER_BOUND('',#1654,.T.);
#1014=FACE_OUTER_BOUND('',#1655,.T.);
#1015=FACE_OUTER_BOUND('',#1656,.T.);
#1016=FACE_OUTER_BOUND('',#1657,.T.);
#1017=FACE_OUTER_BOUND('',#1658,.T.);
#1018=FACE_OUTER_BOUND('',#1659,.T.);
#1019=FACE_OUTER_BOUND('',#1660,.T.);
#1020=FACE_OUTER_BOUND('',#1661,.T.);
#1021=FACE_OUTER_BOUND('',#1662,.T.);
#1022=FACE_OUTER_BOUND('',#1663,.T.);
#1023=FACE_OUTER_BOUND('',#1664,.T.);
#1024=FACE_OUTER_BOUND('',#1665,.T.);
#1025=FACE_OUTER_BOUND('',#1666,.T.);
#1026=FACE_OUTER_BOUND('',#1667,.T.);
#1027=FACE_OUTER_BOUND('',#1668,.T.);
#1028=FACE_OUTER_BOUND('',#1669,.T.);
#1029=FACE_OUTER_BOUND('',#1670,.T.);
#1030=FACE_OUTER_BOUND('',#1671,.T.);
#1031=FACE_OUTER_BOUND('',#1672,.T.);
#1032=FACE_OUTER_BOUND('',#1673,.T.);
#1033=FACE_OUTER_BOUND('',#1674,.T.);
#1034=FACE_OUTER_BOUND('',#1675,.T.);
#1035=FACE_OUTER_BOUND('',#1676,.T.);
#1036=FACE_OUTER_BOUND('',#1677,.T.);
#1037=FACE_OUTER_BOUND('',#1678,.T.);
#1038=FACE_OUTER_BOUND('',#1679,.T.);
#1039=FACE_OUTER_BOUND('',#1680,.T.);
#1040=FACE_OUTER_BOUND('',#1681,.T.);
#1041=FACE_OUTER_BOUND('',#1682,.T.);
#1042=FACE_OUTER_BOUND('',#1683,.T.);
#1043=FACE_OUTER_BOUND('',#1684,.T.);
#1044=FACE_OUTER_BOUND('',#1686,.T.);
#1045=FACE_OUTER_BOUND('',#1687,.T.);
#1046=FACE_OUTER_BOUND('',#1688,.T.);
#1047=FACE_OUTER_BOUND('',#1689,.T.);
#1048=FACE_OUTER_BOUND('',#1690,.T.);
#1049=FACE_OUTER_BOUND('',#1691,.T.);
#1050=FACE_OUTER_BOUND('',#1692,.T.);
#1051=FACE_OUTER_BOUND('',#1693,.T.);
#1052=FACE_OUTER_BOUND('',#1694,.T.);
#1053=FACE_OUTER_BOUND('',#1695,.T.);
#1054=FACE_OUTER_BOUND('',#1696,.T.);
#1055=FACE_OUTER_BOUND('',#1697,.T.);
#1056=FACE_OUTER_BOUND('',#1698,.T.);
#1057=FACE_OUTER_BOUND('',#1699,.T.);
#1058=FACE_OUTER_BOUND('',#1700,.T.);
#1059=FACE_OUTER_BOUND('',#1701,.T.);
#1060=FACE_OUTER_BOUND('',#1702,.T.);
#1061=FACE_OUTER_BOUND('',#1703,.T.);
#1062=FACE_OUTER_BOUND('',#1704,.T.);
#1063=FACE_OUTER_BOUND('',#1705,.T.);
#1064=FACE_OUTER_BOUND('',#1706,.T.);
#1065=FACE_OUTER_BOUND('',#1707,.T.);
#1066=FACE_OUTER_BOUND('',#1708,.T.);
#1067=FACE_OUTER_BOUND('',#1709,.T.);
#1068=FACE_OUTER_BOUND('',#1710,.T.);
#1069=FACE_OUTER_BOUND('',#1711,.T.);
#1070=FACE_OUTER_BOUND('',#1712,.T.);
#1071=FACE_OUTER_BOUND('',#1713,.T.);
#1072=FACE_OUTER_BOUND('',#1714,.T.);
#1073=FACE_OUTER_BOUND('',#1715,.T.);
#1074=FACE_OUTER_BOUND('',#1716,.T.);
#1075=FACE_OUTER_BOUND('',#1717,.T.);
#1076=FACE_OUTER_BOUND('',#1718,.T.);
#1077=FACE_OUTER_BOUND('',#1719,.T.);
#1078=FACE_OUTER_BOUND('',#1720,.T.);
#1079=FACE_OUTER_BOUND('',#1721,.T.);
#1080=FACE_OUTER_BOUND('',#1722,.T.);
#1081=FACE_OUTER_BOUND('',#1723,.T.);
#1082=FACE_OUTER_BOUND('',#1724,.T.);
#1083=FACE_OUTER_BOUND('',#1725,.T.);
#1084=FACE_OUTER_BOUND('',#1726,.T.);
#1085=FACE_OUTER_BOUND('',#1727,.T.);
#1086=FACE_OUTER_BOUND('',#1728,.T.);
#1087=FACE_OUTER_BOUND('',#1729,.T.);
#1088=FACE_OUTER_BOUND('',#1730,.T.);
#1089=FACE_OUTER_BOUND('',#1731,.T.);
#1090=FACE_OUTER_BOUND('',#1732,.T.);
#1091=FACE_OUTER_BOUND('',#1733,.T.);
#1092=FACE_OUTER_BOUND('',#1734,.T.);
#1093=FACE_OUTER_BOUND('',#1735,.T.);
#1094=FACE_OUTER_BOUND('',#1736,.T.);
#1095=FACE_OUTER_BOUND('',#1737,.T.);
#1096=FACE_OUTER_BOUND('',#1738,.T.);
#1097=FACE_OUTER_BOUND('',#1740,.T.);
#1098=FACE_OUTER_BOUND('',#1742,.T.);
#1099=FACE_OUTER_BOUND('',#1744,.T.);
#1100=FACE_OUTER_BOUND('',#1746,.T.);
#1101=FACE_OUTER_BOUND('',#1748,.T.);
#1102=FACE_OUTER_BOUND('',#1750,.T.);
#1103=FACE_OUTER_BOUND('',#1751,.T.);
#1104=FACE_OUTER_BOUND('',#1752,.T.);
#1105=FACE_OUTER_BOUND('',#1753,.T.);
#1106=FACE_OUTER_BOUND('',#1754,.T.);
#1107=FACE_OUTER_BOUND('',#1755,.T.);
#1108=FACE_OUTER_BOUND('',#1756,.T.);
#1109=FACE_OUTER_BOUND('',#1757,.T.);
#1110=FACE_OUTER_BOUND('',#1758,.T.);
#1111=FACE_OUTER_BOUND('',#1759,.T.);
#1112=FACE_OUTER_BOUND('',#1760,.T.);
#1113=FACE_OUTER_BOUND('',#1761,.T.);
#1114=FACE_OUTER_BOUND('',#1762,.T.);
#1115=FACE_OUTER_BOUND('',#1763,.T.);
#1116=FACE_OUTER_BOUND('',#1764,.T.);
#1117=FACE_OUTER_BOUND('',#1765,.T.);
#1118=FACE_OUTER_BOUND('',#1766,.T.);
#1119=FACE_OUTER_BOUND('',#1767,.T.);
#1120=FACE_OUTER_BOUND('',#1768,.T.);
#1121=FACE_OUTER_BOUND('',#1769,.T.);
#1122=FACE_OUTER_BOUND('',#1770,.T.);
#1123=FACE_OUTER_BOUND('',#1771,.T.);
#1124=FACE_OUTER_BOUND('',#1772,.T.);
#1125=FACE_OUTER_BOUND('',#1773,.T.);
#1126=FACE_OUTER_BOUND('',#1774,.T.);
#1127=FACE_OUTER_BOUND('',#1775,.T.);
#1128=FACE_OUTER_BOUND('',#1776,.T.);
#1129=FACE_OUTER_BOUND('',#1777,.T.);
#1130=FACE_OUTER_BOUND('',#1778,.T.);
#1131=FACE_OUTER_BOUND('',#1779,.T.);
#1132=FACE_OUTER_BOUND('',#1780,.T.);
#1133=FACE_OUTER_BOUND('',#1781,.T.);
#1134=FACE_OUTER_BOUND('',#1782,.T.);
#1135=FACE_OUTER_BOUND('',#1783,.T.);
#1136=FACE_OUTER_BOUND('',#1784,.T.);
#1137=FACE_OUTER_BOUND('',#1785,.T.);
#1138=FACE_OUTER_BOUND('',#1786,.T.);
#1139=FACE_OUTER_BOUND('',#1787,.T.);
#1140=FACE_OUTER_BOUND('',#1788,.T.);
#1141=FACE_OUTER_BOUND('',#1789,.T.);
#1142=FACE_OUTER_BOUND('',#1790,.T.);
#1143=FACE_OUTER_BOUND('',#1791,.T.);
#1144=FACE_OUTER_BOUND('',#1792,.T.);
#1145=FACE_OUTER_BOUND('',#1793,.T.);
#1146=FACE_OUTER_BOUND('',#1794,.T.);
#1147=FACE_OUTER_BOUND('',#1795,.T.);
#1148=FACE_OUTER_BOUND('',#1796,.T.);
#1149=FACE_OUTER_BOUND('',#1797,.T.);
#1150=FACE_OUTER_BOUND('',#1798,.T.);
#1151=FACE_OUTER_BOUND('',#1799,.T.);
#1152=FACE_OUTER_BOUND('',#1800,.T.);
#1153=FACE_OUTER_BOUND('',#1801,.T.);
#1154=FACE_OUTER_BOUND('',#1802,.T.);
#1155=FACE_OUTER_BOUND('',#1803,.T.);
#1156=FACE_OUTER_BOUND('',#1804,.T.);
#1157=FACE_OUTER_BOUND('',#1805,.T.);
#1158=FACE_OUTER_BOUND('',#1806,.T.);
#1159=FACE_OUTER_BOUND('',#1807,.T.);
#1160=FACE_OUTER_BOUND('',#1808,.T.);
#1161=FACE_OUTER_BOUND('',#1809,.T.);
#1162=FACE_OUTER_BOUND('',#1810,.T.);
#1163=FACE_OUTER_BOUND('',#1811,.T.);
#1164=FACE_OUTER_BOUND('',#1812,.T.);
#1165=FACE_OUTER_BOUND('',#1813,.T.);
#1166=FACE_OUTER_BOUND('',#1814,.T.);
#1167=FACE_OUTER_BOUND('',#1815,.T.);
#1168=FACE_OUTER_BOUND('',#1817,.T.);
#1169=FACE_OUTER_BOUND('',#1819,.T.);
#1170=FACE_OUTER_BOUND('',#1821,.T.);
#1171=FACE_OUTER_BOUND('',#1823,.T.);
#1172=FACE_OUTER_BOUND('',#1825,.T.);
#1173=FACE_OUTER_BOUND('',#1827,.T.);
#1174=FACE_OUTER_BOUND('',#1828,.T.);
#1175=FACE_OUTER_BOUND('',#1829,.T.);
#1176=FACE_OUTER_BOUND('',#1830,.T.);
#1177=FACE_OUTER_BOUND('',#1831,.T.);
#1178=FACE_OUTER_BOUND('',#1832,.T.);
#1179=FACE_OUTER_BOUND('',#1833,.T.);
#1180=FACE_OUTER_BOUND('',#1834,.T.);
#1181=FACE_OUTER_BOUND('',#1835,.T.);
#1182=FACE_OUTER_BOUND('',#1836,.T.);
#1183=FACE_OUTER_BOUND('',#1837,.T.);
#1184=FACE_OUTER_BOUND('',#1838,.T.);
#1185=FACE_OUTER_BOUND('',#1840,.T.);
#1186=FACE_OUTER_BOUND('',#1841,.T.);
#1187=FACE_OUTER_BOUND('',#1842,.T.);
#1188=FACE_OUTER_BOUND('',#1843,.T.);
#1189=FACE_OUTER_BOUND('',#1844,.T.);
#1190=FACE_OUTER_BOUND('',#1845,.T.);
#1191=FACE_OUTER_BOUND('',#1846,.T.);
#1192=FACE_OUTER_BOUND('',#1847,.T.);
#1193=FACE_OUTER_BOUND('',#1849,.T.);
#1194=FACE_OUTER_BOUND('',#1850,.T.);
#1195=FACE_OUTER_BOUND('',#1851,.T.);
#1196=FACE_OUTER_BOUND('',#1852,.T.);
#1197=FACE_OUTER_BOUND('',#1853,.T.);
#1198=FACE_OUTER_BOUND('',#1854,.T.);
#1199=FACE_OUTER_BOUND('',#1855,.T.);
#1200=FACE_OUTER_BOUND('',#1856,.T.);
#1201=FACE_OUTER_BOUND('',#1857,.T.);
#1202=FACE_OUTER_BOUND('',#1858,.T.);
#1203=FACE_OUTER_BOUND('',#1859,.T.);
#1204=FACE_OUTER_BOUND('',#1860,.T.);
#1205=FACE_OUTER_BOUND('',#1861,.T.);
#1206=FACE_OUTER_BOUND('',#1862,.T.);
#1207=FACE_OUTER_BOUND('',#1863,.T.);
#1208=FACE_OUTER_BOUND('',#1864,.T.);
#1209=FACE_OUTER_BOUND('',#1865,.T.);
#1210=FACE_OUTER_BOUND('',#1866,.T.);
#1211=FACE_OUTER_BOUND('',#1867,.T.);
#1212=FACE_OUTER_BOUND('',#1868,.T.);
#1213=FACE_OUTER_BOUND('',#1869,.T.);
#1214=FACE_OUTER_BOUND('',#1870,.T.);
#1215=FACE_OUTER_BOUND('',#1871,.T.);
#1216=FACE_OUTER_BOUND('',#1872,.T.);
#1217=FACE_OUTER_BOUND('',#1873,.T.);
#1218=FACE_OUTER_BOUND('',#1874,.T.);
#1219=FACE_OUTER_BOUND('',#1876,.T.);
#1220=FACE_OUTER_BOUND('',#1877,.T.);
#1221=FACE_OUTER_BOUND('',#1878,.T.);
#1222=FACE_OUTER_BOUND('',#1879,.T.);
#1223=FACE_OUTER_BOUND('',#1880,.T.);
#1224=FACE_OUTER_BOUND('',#1882,.T.);
#1225=FACE_OUTER_BOUND('',#1883,.T.);
#1226=FACE_OUTER_BOUND('',#1884,.T.);
#1227=FACE_OUTER_BOUND('',#1885,.T.);
#1228=FACE_OUTER_BOUND('',#1886,.T.);
#1229=FACE_OUTER_BOUND('',#1887,.T.);
#1230=FACE_OUTER_BOUND('',#1888,.T.);
#1231=FACE_OUTER_BOUND('',#1889,.T.);
#1232=FACE_OUTER_BOUND('',#1890,.T.);
#1233=FACE_OUTER_BOUND('',#1891,.T.);
#1234=FACE_OUTER_BOUND('',#1892,.T.);
#1235=FACE_OUTER_BOUND('',#1893,.T.);
#1236=FACE_OUTER_BOUND('',#1894,.T.);
#1237=FACE_OUTER_BOUND('',#1895,.T.);
#1238=FACE_OUTER_BOUND('',#1896,.T.);
#1239=FACE_OUTER_BOUND('',#1897,.T.);
#1240=FACE_OUTER_BOUND('',#1898,.T.);
#1241=FACE_OUTER_BOUND('',#1899,.T.);
#1242=FACE_OUTER_BOUND('',#1900,.T.);
#1243=FACE_OUTER_BOUND('',#1901,.T.);
#1244=FACE_OUTER_BOUND('',#1902,.T.);
#1245=FACE_OUTER_BOUND('',#1903,.T.);
#1246=FACE_OUTER_BOUND('',#1904,.T.);
#1247=FACE_OUTER_BOUND('',#1905,.T.);
#1248=FACE_OUTER_BOUND('',#1906,.T.);
#1249=FACE_OUTER_BOUND('',#1907,.T.);
#1250=FACE_OUTER_BOUND('',#1908,.T.);
#1251=FACE_OUTER_BOUND('',#1909,.T.);
#1252=FACE_OUTER_BOUND('',#1911,.T.);
#1253=FACE_OUTER_BOUND('',#1912,.T.);
#1254=FACE_OUTER_BOUND('',#1914,.T.);
#1255=FACE_OUTER_BOUND('',#1916,.T.);
#1256=FACE_OUTER_BOUND('',#1918,.T.);
#1577=EDGE_LOOP('',(#7445,#7446,#7447,#7448));
#1578=EDGE_LOOP('',(#7449,#7450,#7451,#7452));
#1579=EDGE_LOOP('',(#7453,#7454,#7455,#7456));
#1580=EDGE_LOOP('',(#7457,#7458,#7459,#7460));
#1581=EDGE_LOOP('',(#7461,#7462,#7463,#7464));
#1582=EDGE_LOOP('',(#7465,#7466,#7467,#7468));
#1583=EDGE_LOOP('',(#7469,#7470,#7471,#7472));
#1584=EDGE_LOOP('',(#7473,#7474,#7475,#7476));
#1585=EDGE_LOOP('',(#7477,#7478,#7479,#7480));
#1586=EDGE_LOOP('',(#7481,#7482,#7483,#7484));
#1587=EDGE_LOOP('',(#7485,#7486,#7487,#7488));
#1588=EDGE_LOOP('',(#7489,#7490,#7491,#7492));
#1589=EDGE_LOOP('',(#7493,#7494,#7495,#7496));
#1590=EDGE_LOOP('',(#7497,#7498,#7499,#7500));
#1591=EDGE_LOOP('',(#7501,#7502,#7503,#7504));
#1592=EDGE_LOOP('',(#7505,#7506,#7507,#7508));
#1593=EDGE_LOOP('',(#7509,#7510,#7511,#7512));
#1594=EDGE_LOOP('',(#7513,#7514,#7515,#7516));
#1595=EDGE_LOOP('',(#7517,#7518,#7519,#7520));
#1596=EDGE_LOOP('',(#7521,#7522,#7523,#7524));
#1597=EDGE_LOOP('',(#7525,#7526,#7527,#7528));
#1598=EDGE_LOOP('',(#7529,#7530,#7531,#7532));
#1599=EDGE_LOOP('',(#7533,#7534,#7535,#7536));
#1600=EDGE_LOOP('',(#7537));
#1601=EDGE_LOOP('',(#7538,#7539,#7540,#7541));
#1602=EDGE_LOOP('',(#7542,#7543,#7544,#7545));
#1603=EDGE_LOOP('',(#7546,#7547,#7548,#7549));
#1604=EDGE_LOOP('',(#7550,#7551,#7552,#7553));
#1605=EDGE_LOOP('',(#7554));
#1606=EDGE_LOOP('',(#7555));
#1607=EDGE_LOOP('',(#7556,#7557,#7558,#7559,#7560,#7561,#7562,#7563,#7564,
#7565,#7566,#7567,#7568,#7569,#7570,#7571,#7572,#7573));
#1608=EDGE_LOOP('',(#7574,#7575,#7576,#7577));
#1609=EDGE_LOOP('',(#7578,#7579,#7580,#7581));
#1610=EDGE_LOOP('',(#7582,#7583,#7584,#7585,#7586,#7587));
#1611=EDGE_LOOP('',(#7588,#7589,#7590));
#1612=EDGE_LOOP('',(#7591,#7592,#7593,#7594,#7595,#7596));
#1613=EDGE_LOOP('',(#7597,#7598,#7599));
#1614=EDGE_LOOP('',(#7600,#7601,#7602,#7603,#7604,#7605));
#1615=EDGE_LOOP('',(#7606,#7607,#7608,#7609));
#1616=EDGE_LOOP('',(#7610,#7611,#7612,#7613));
#1617=EDGE_LOOP('',(#7614,#7615,#7616,#7617));
#1618=EDGE_LOOP('',(#7618,#7619,#7620,#7621,#7622,#7623,#7624,#7625,#7626,
#7627,#7628,#7629,#7630,#7631,#7632,#7633,#7634,#7635,#7636,#7637,#7638,
#7639,#7640,#7641,#7642,#7643,#7644,#7645,#7646,#7647,#7648,#7649,#7650,
#7651,#7652,#7653,#7654,#7655,#7656,#7657));
#1619=EDGE_LOOP('',(#7658));
#1620=EDGE_LOOP('',(#7659));
#1621=EDGE_LOOP('',(#7660));
#1622=EDGE_LOOP('',(#7661));
#1623=EDGE_LOOP('',(#7662));
#1624=EDGE_LOOP('',(#7663));
#1625=EDGE_LOOP('',(#7664,#7665,#7666,#7667));
#1626=EDGE_LOOP('',(#7668,#7669,#7670,#7671));
#1627=EDGE_LOOP('',(#7672,#7673,#7674,#7675));
#1628=EDGE_LOOP('',(#7676,#7677,#7678,#7679));
#1629=EDGE_LOOP('',(#7680,#7681,#7682,#7683));
#1630=EDGE_LOOP('',(#7684,#7685,#7686,#7687));
#1631=EDGE_LOOP('',(#7688,#7689,#7690,#7691,#7692,#7693,#7694,#7695,#7696,
#7697,#7698,#7699,#7700,#7701,#7702,#7703,#7704,#7705,#7706,#7707,#7708,
#7709,#7710,#7711));
#1632=EDGE_LOOP('',(#7712));
#1633=EDGE_LOOP('',(#7713));
#1634=EDGE_LOOP('',(#7714));
#1635=EDGE_LOOP('',(#7715));
#1636=EDGE_LOOP('',(#7716));
#1637=EDGE_LOOP('',(#7717));
#1638=EDGE_LOOP('',(#7718,#7719,#7720,#7721));
#1639=EDGE_LOOP('',(#7722,#7723,#7724,#7725));
#1640=EDGE_LOOP('',(#7726,#7727,#7728,#7729));
#1641=EDGE_LOOP('',(#7730,#7731,#7732,#7733));
#1642=EDGE_LOOP('',(#7734));
#1643=EDGE_LOOP('',(#7735));
#1644=EDGE_LOOP('',(#7736,#7737,#7738,#7739,#7740,#7741,#7742,#7743));
#1645=EDGE_LOOP('',(#7744,#7745,#7746,#7747,#7748,#7749));
#1646=EDGE_LOOP('',(#7750,#7751,#7752,#7753,#7754,#7755,#7756,#7757,#7758,
#7759,#7760,#7761,#7762,#7763,#7764,#7765,#7766,#7767,#7768,#7769,#7770,
#7771,#7772,#7773,#7774,#7775,#7776,#7777,#7778,#7779,#7780,#7781,#7782,
#7783,#7784,#7785,#7786,#7787,#7788,#7789));
#1647=EDGE_LOOP('',(#7790,#7791,#7792,#7793,#7794,#7795));
#1648=EDGE_LOOP('',(#7796,#7797,#7798,#7799,#7800,#7801,#7802,#7803));
#1649=EDGE_LOOP('',(#7804,#7805,#7806,#7807));
#1650=EDGE_LOOP('',(#7808,#7809,#7810,#7811,#7812,#7813,#7814,#7815,#7816,
#7817,#7818,#7819,#7820,#7821,#7822,#7823));
#1651=EDGE_LOOP('',(#7824,#7825,#7826,#7827));
#1652=EDGE_LOOP('',(#7828,#7829,#7830,#7831));
#1653=EDGE_LOOP('',(#7832,#7833,#7834,#7835,#7836,#7837));
#1654=EDGE_LOOP('',(#7838,#7839,#7840,#7841,#7842,#7843,#7844,#7845,#7846,
#7847,#7848,#7849));
#1655=EDGE_LOOP('',(#7850,#7851,#7852,#7853,#7854,#7855));
#1656=EDGE_LOOP('',(#7856,#7857,#7858,#7859));
#1657=EDGE_LOOP('',(#7860,#7861,#7862,#7863));
#1658=EDGE_LOOP('',(#7864,#7865,#7866,#7867,#7868,#7869,#7870,#7871,#7872,
#7873,#7874,#7875,#7876,#7877,#7878,#7879));
#1659=EDGE_LOOP('',(#7880,#7881,#7882,#7883));
#1660=EDGE_LOOP('',(#7884,#7885,#7886,#7887));
#1661=EDGE_LOOP('',(#7888,#7889,#7890,#7891));
#1662=EDGE_LOOP('',(#7892,#7893,#7894,#7895));
#1663=EDGE_LOOP('',(#7896,#7897,#7898,#7899,#7900));
#1664=EDGE_LOOP('',(#7901,#7902,#7903,#7904));
#1665=EDGE_LOOP('',(#7905,#7906,#7907,#7908,#7909,#7910));
#1666=EDGE_LOOP('',(#7911,#7912,#7913,#7914));
#1667=EDGE_LOOP('',(#7915,#7916,#7917,#7918,#7919));
#1668=EDGE_LOOP('',(#7920,#7921,#7922,#7923));
#1669=EDGE_LOOP('',(#7924,#7925,#7926,#7927,#7928));
#1670=EDGE_LOOP('',(#7929,#7930,#7931,#7932));
#1671=EDGE_LOOP('',(#7933,#7934,#7935,#7936,#7937,#7938));
#1672=EDGE_LOOP('',(#7939,#7940,#7941,#7942));
#1673=EDGE_LOOP('',(#7943,#7944,#7945,#7946,#7947));
#1674=EDGE_LOOP('',(#7948,#7949,#7950,#7951));
#1675=EDGE_LOOP('',(#7952,#7953,#7954,#7955,#7956));
#1676=EDGE_LOOP('',(#7957,#7958,#7959,#7960));
#1677=EDGE_LOOP('',(#7961,#7962,#7963,#7964,#7965,#7966));
#1678=EDGE_LOOP('',(#7967,#7968,#7969,#7970));
#1679=EDGE_LOOP('',(#7971,#7972,#7973,#7974,#7975));
#1680=EDGE_LOOP('',(#7976,#7977,#7978,#7979));
#1681=EDGE_LOOP('',(#7980,#7981,#7982,#7983));
#1682=EDGE_LOOP('',(#7984,#7985,#7986,#7987));
#1683=EDGE_LOOP('',(#7988,#7989,#7990,#7991,#7992,#7993,#7994,#7995));
#1684=EDGE_LOOP('',(#7996,#7997,#7998,#7999,#8000,#8001,#8002,#8003,#8004,
#8005,#8006,#8007,#8008,#8009,#8010,#8011));
#1685=EDGE_LOOP('',(#8012));
#1686=EDGE_LOOP('',(#8013,#8014,#8015,#8016,#8017,#8018));
#1687=EDGE_LOOP('',(#8019,#8020,#8021,#8022,#8023,#8024));
#1688=EDGE_LOOP('',(#8025,#8026,#8027,#8028,#8029,#8030,#8031,#8032,#8033,
#8034,#8035,#8036,#8037,#8038,#8039,#8040,#8041,#8042,#8043,#8044,#8045,
#8046,#8047,#8048,#8049,#8050,#8051,#8052,#8053,#8054,#8055,#8056,#8057,
#8058,#8059,#8060,#8061,#8062,#8063,#8064));
#1689=EDGE_LOOP('',(#8065,#8066,#8067,#8068,#8069,#8070,#8071,#8072));
#1690=EDGE_LOOP('',(#8073,#8074,#8075,#8076,#8077,#8078,#8079,#8080,#8081,
#8082,#8083,#8084,#8085,#8086,#8087,#8088));
#1691=EDGE_LOOP('',(#8089,#8090,#8091,#8092));
#1692=EDGE_LOOP('',(#8093,#8094,#8095,#8096));
#1693=EDGE_LOOP('',(#8097,#8098,#8099,#8100,#8101,#8102));
#1694=EDGE_LOOP('',(#8103,#8104,#8105,#8106,#8107,#8108,#8109,#8110,#8111,
#8112,#8113,#8114));
#1695=EDGE_LOOP('',(#8115,#8116,#8117,#8118,#8119,#8120));
#1696=EDGE_LOOP('',(#8121,#8122,#8123,#8124));
#1697=EDGE_LOOP('',(#8125,#8126,#8127,#8128));
#1698=EDGE_LOOP('',(#8129,#8130,#8131,#8132,#8133,#8134,#8135,#8136,#8137,
#8138,#8139,#8140,#8141,#8142,#8143,#8144));
#1699=EDGE_LOOP('',(#8145,#8146,#8147,#8148));
#1700=EDGE_LOOP('',(#8149,#8150,#8151,#8152));
#1701=EDGE_LOOP('',(#8153,#8154,#8155,#8156));
#1702=EDGE_LOOP('',(#8157,#8158,#8159,#8160,#8161));
#1703=EDGE_LOOP('',(#8162,#8163,#8164,#8165));
#1704=EDGE_LOOP('',(#8166,#8167,#8168,#8169));
#1705=EDGE_LOOP('',(#8170,#8171,#8172,#8173,#8174,#8175));
#1706=EDGE_LOOP('',(#8176,#8177,#8178,#8179));
#1707=EDGE_LOOP('',(#8180,#8181,#8182,#8183,#8184,#8185));
#1708=EDGE_LOOP('',(#8186,#8187,#8188,#8189));
#1709=EDGE_LOOP('',(#8190,#8191,#8192));
#1710=EDGE_LOOP('',(#8193,#8194,#8195,#8196,#8197,#8198,#8199,#8200));
#1711=EDGE_LOOP('',(#8201,#8202,#8203,#8204));
#1712=EDGE_LOOP('',(#8205,#8206,#8207,#8208));
#1713=EDGE_LOOP('',(#8209,#8210,#8211,#8212));
#1714=EDGE_LOOP('',(#8213,#8214,#8215,#8216));
#1715=EDGE_LOOP('',(#8217,#8218,#8219,#8220));
#1716=EDGE_LOOP('',(#8221,#8222,#8223,#8224,#8225,#8226,#8227));
#1717=EDGE_LOOP('',(#8228,#8229,#8230));
#1718=EDGE_LOOP('',(#8231,#8232,#8233,#8234,#8235));
#1719=EDGE_LOOP('',(#8236,#8237,#8238,#8239));
#1720=EDGE_LOOP('',(#8240,#8241,#8242,#8243));
#1721=EDGE_LOOP('',(#8244,#8245,#8246,#8247));
#1722=EDGE_LOOP('',(#8248,#8249,#8250,#8251,#8252));
#1723=EDGE_LOOP('',(#8253,#8254,#8255));
#1724=EDGE_LOOP('',(#8256,#8257,#8258,#8259,#8260));
#1725=EDGE_LOOP('',(#8261,#8262,#8263,#8264));
#1726=EDGE_LOOP('',(#8265,#8266,#8267));
#1727=EDGE_LOOP('',(#8268,#8269,#8270,#8271,#8272));
#1728=EDGE_LOOP('',(#8273,#8274,#8275,#8276));
#1729=EDGE_LOOP('',(#8277,#8278,#8279,#8280));
#1730=EDGE_LOOP('',(#8281,#8282,#8283,#8284));
#1731=EDGE_LOOP('',(#8285,#8286,#8287,#8288,#8289));
#1732=EDGE_LOOP('',(#8290,#8291,#8292));
#1733=EDGE_LOOP('',(#8293,#8294,#8295,#8296,#8297));
#1734=EDGE_LOOP('',(#8298,#8299,#8300,#8301));
#1735=EDGE_LOOP('',(#8302,#8303,#8304,#8305,#8306,#8307));
#1736=EDGE_LOOP('',(#8308,#8309,#8310));
#1737=EDGE_LOOP('',(#8311,#8312,#8313,#8314));
#1738=EDGE_LOOP('',(#8315,#8316,#8317,#8318,#8319,#8320));
#1739=EDGE_LOOP('',(#8321));
#1740=EDGE_LOOP('',(#8322,#8323,#8324,#8325,#8326));
#1741=EDGE_LOOP('',(#8327));
#1742=EDGE_LOOP('',(#8328,#8329,#8330,#8331,#8332,#8333,#8334));
#1743=EDGE_LOOP('',(#8335));
#1744=EDGE_LOOP('',(#8336,#8337,#8338,#8339,#8340,#8341));
#1745=EDGE_LOOP('',(#8342));
#1746=EDGE_LOOP('',(#8343,#8344,#8345,#8346,#8347));
#1747=EDGE_LOOP('',(#8348));
#1748=EDGE_LOOP('',(#8349,#8350,#8351,#8352,#8353,#8354,#8355));
#1749=EDGE_LOOP('',(#8356));
#1750=EDGE_LOOP('',(#8357,#8358,#8359,#8360));
#1751=EDGE_LOOP('',(#8361,#8362,#8363,#8364));
#1752=EDGE_LOOP('',(#8365,#8366,#8367,#8368));
#1753=EDGE_LOOP('',(#8369,#8370,#8371,#8372));
#1754=EDGE_LOOP('',(#8373,#8374,#8375,#8376));
#1755=EDGE_LOOP('',(#8377,#8378,#8379,#8380));
#1756=EDGE_LOOP('',(#8381,#8382,#8383,#8384));
#1757=EDGE_LOOP('',(#8385,#8386,#8387,#8388,#8389,#8390,#8391,#8392));
#1758=EDGE_LOOP('',(#8393,#8394,#8395));
#1759=EDGE_LOOP('',(#8396,#8397,#8398,#8399));
#1760=EDGE_LOOP('',(#8400,#8401,#8402,#8403));
#1761=EDGE_LOOP('',(#8404,#8405,#8406,#8407));
#1762=EDGE_LOOP('',(#8408,#8409,#8410,#8411));
#1763=EDGE_LOOP('',(#8412,#8413,#8414,#8415));
#1764=EDGE_LOOP('',(#8416,#8417,#8418,#8419));
#1765=EDGE_LOOP('',(#8420,#8421,#8422,#8423));
#1766=EDGE_LOOP('',(#8424,#8425,#8426,#8427));
#1767=EDGE_LOOP('',(#8428,#8429,#8430,#8431));
#1768=EDGE_LOOP('',(#8432,#8433,#8434,#8435));
#1769=EDGE_LOOP('',(#8436,#8437,#8438,#8439));
#1770=EDGE_LOOP('',(#8440,#8441,#8442,#8443));
#1771=EDGE_LOOP('',(#8444,#8445,#8446,#8447));
#1772=EDGE_LOOP('',(#8448,#8449,#8450,#8451));
#1773=EDGE_LOOP('',(#8452,#8453,#8454,#8455));
#1774=EDGE_LOOP('',(#8456,#8457,#8458,#8459));
#1775=EDGE_LOOP('',(#8460,#8461,#8462,#8463));
#1776=EDGE_LOOP('',(#8464,#8465,#8466,#8467));
#1777=EDGE_LOOP('',(#8468,#8469,#8470,#8471));
#1778=EDGE_LOOP('',(#8472,#8473,#8474,#8475));
#1779=EDGE_LOOP('',(#8476,#8477,#8478,#8479));
#1780=EDGE_LOOP('',(#8480,#8481,#8482,#8483));
#1781=EDGE_LOOP('',(#8484,#8485,#8486,#8487));
#1782=EDGE_LOOP('',(#8488,#8489,#8490,#8491));
#1783=EDGE_LOOP('',(#8492,#8493,#8494,#8495));
#1784=EDGE_LOOP('',(#8496,#8497,#8498,#8499,#8500));
#1785=EDGE_LOOP('',(#8501,#8502,#8503,#8504));
#1786=EDGE_LOOP('',(#8505,#8506,#8507,#8508));
#1787=EDGE_LOOP('',(#8509,#8510,#8511,#8512,#8513,#8514));
#1788=EDGE_LOOP('',(#8515,#8516,#8517,#8518));
#1789=EDGE_LOOP('',(#8519,#8520,#8521,#8522,#8523));
#1790=EDGE_LOOP('',(#8524,#8525,#8526));
#1791=EDGE_LOOP('',(#8527,#8528,#8529,#8530,#8531));
#1792=EDGE_LOOP('',(#8532,#8533,#8534,#8535));
#1793=EDGE_LOOP('',(#8536,#8537,#8538,#8539));
#1794=EDGE_LOOP('',(#8540,#8541,#8542,#8543));
#1795=EDGE_LOOP('',(#8544,#8545,#8546,#8547,#8548));
#1796=EDGE_LOOP('',(#8549,#8550,#8551));
#1797=EDGE_LOOP('',(#8552,#8553,#8554,#8555,#8556));
#1798=EDGE_LOOP('',(#8557,#8558,#8559));
#1799=EDGE_LOOP('',(#8560,#8561,#8562,#8563,#8564));
#1800=EDGE_LOOP('',(#8565,#8566,#8567,#8568,#8569));
#1801=EDGE_LOOP('',(#8570,#8571,#8572));
#1802=EDGE_LOOP('',(#8573,#8574,#8575,#8576,#8577,#8578,#8579));
#1803=EDGE_LOOP('',(#8580,#8581,#8582,#8583));
#1804=EDGE_LOOP('',(#8584,#8585,#8586,#8587));
#1805=EDGE_LOOP('',(#8588,#8589,#8590,#8591));
#1806=EDGE_LOOP('',(#8592,#8593,#8594,#8595));
#1807=EDGE_LOOP('',(#8596,#8597,#8598,#8599));
#1808=EDGE_LOOP('',(#8600,#8601,#8602,#8603));
#1809=EDGE_LOOP('',(#8604,#8605,#8606,#8607,#8608,#8609));
#1810=EDGE_LOOP('',(#8610,#8611,#8612,#8613));
#1811=EDGE_LOOP('',(#8614,#8615,#8616,#8617,#8618,#8619));
#1812=EDGE_LOOP('',(#8620,#8621,#8622,#8623));
#1813=EDGE_LOOP('',(#8624,#8625,#8626));
#1814=EDGE_LOOP('',(#8627,#8628,#8629,#8630));
#1815=EDGE_LOOP('',(#8631,#8632,#8633,#8634,#8635,#8636));
#1816=EDGE_LOOP('',(#8637));
#1817=EDGE_LOOP('',(#8638,#8639,#8640,#8641,#8642));
#1818=EDGE_LOOP('',(#8643));
#1819=EDGE_LOOP('',(#8644,#8645,#8646,#8647,#8648,#8649,#8650));
#1820=EDGE_LOOP('',(#8651));
#1821=EDGE_LOOP('',(#8652,#8653,#8654,#8655,#8656,#8657));
#1822=EDGE_LOOP('',(#8658));
#1823=EDGE_LOOP('',(#8659,#8660,#8661,#8662,#8663));
#1824=EDGE_LOOP('',(#8664));
#1825=EDGE_LOOP('',(#8665,#8666,#8667,#8668,#8669,#8670,#8671));
#1826=EDGE_LOOP('',(#8672));
#1827=EDGE_LOOP('',(#8673,#8674,#8675,#8676));
#1828=EDGE_LOOP('',(#8677,#8678,#8679,#8680));
#1829=EDGE_LOOP('',(#8681,#8682,#8683,#8684));
#1830=EDGE_LOOP('',(#8685,#8686,#8687,#8688));
#1831=EDGE_LOOP('',(#8689,#8690,#8691,#8692));
#1832=EDGE_LOOP('',(#8693,#8694,#8695,#8696));
#1833=EDGE_LOOP('',(#8697,#8698,#8699,#8700));
#1834=EDGE_LOOP('',(#8701,#8702,#8703,#8704));
#1835=EDGE_LOOP('',(#8705,#8706,#8707,#8708));
#1836=EDGE_LOOP('',(#8709,#8710,#8711,#8712));
#1837=EDGE_LOOP('',(#8713,#8714,#8715,#8716));
#1838=EDGE_LOOP('',(#8717));
#1839=EDGE_LOOP('',(#8718));
#1840=EDGE_LOOP('',(#8719,#8720,#8721,#8722,#8723));
#1841=EDGE_LOOP('',(#8724,#8725,#8726,#8727));
#1842=EDGE_LOOP('',(#8728,#8729,#8730,#8731,#8732));
#1843=EDGE_LOOP('',(#8733,#8734,#8735,#8736,#8737,#8738,#8739,#8740,#8741,
#8742,#8743,#8744,#8745,#8746,#8747,#8748,#8749,#8750,#8751,#8752));
#1844=EDGE_LOOP('',(#8753,#8754,#8755,#8756,#8757));
#1845=EDGE_LOOP('',(#8758,#8759,#8760,#8761));
#1846=EDGE_LOOP('',(#8762,#8763,#8764,#8765,#8766,#8767));
#1847=EDGE_LOOP('',(#8768,#8769,#8770,#8771,#8772,#8773,#8774,#8775));
#1848=EDGE_LOOP('',(#8776,#8777,#8778,#8779));
#1849=EDGE_LOOP('',(#8780,#8781,#8782,#8783));
#1850=EDGE_LOOP('',(#8784,#8785,#8786,#8787,#8788));
#1851=EDGE_LOOP('',(#8789,#8790,#8791,#8792,#8793));
#1852=EDGE_LOOP('',(#8794,#8795,#8796,#8797,#8798));
#1853=EDGE_LOOP('',(#8799,#8800,#8801,#8802,#8803));
#1854=EDGE_LOOP('',(#8804,#8805,#8806,#8807,#8808));
#1855=EDGE_LOOP('',(#8809,#8810,#8811,#8812,#8813));
#1856=EDGE_LOOP('',(#8814,#8815,#8816,#8817,#8818));
#1857=EDGE_LOOP('',(#8819,#8820,#8821,#8822));
#1858=EDGE_LOOP('',(#8823,#8824,#8825,#8826,#8827));
#1859=EDGE_LOOP('',(#8828,#8829,#8830,#8831,#8832));
#1860=EDGE_LOOP('',(#8833,#8834,#8835,#8836,#8837));
#1861=EDGE_LOOP('',(#8838,#8839,#8840,#8841,#8842));
#1862=EDGE_LOOP('',(#8843,#8844,#8845,#8846,#8847));
#1863=EDGE_LOOP('',(#8848,#8849,#8850,#8851,#8852));
#1864=EDGE_LOOP('',(#8853,#8854,#8855,#8856,#8857));
#1865=EDGE_LOOP('',(#8858,#8859,#8860,#8861,#8862,#8863));
#1866=EDGE_LOOP('',(#8864,#8865,#8866,#8867,#8868));
#1867=EDGE_LOOP('',(#8869,#8870,#8871,#8872,#8873));
#1868=EDGE_LOOP('',(#8874,#8875,#8876));
#1869=EDGE_LOOP('',(#8877,#8878,#8879));
#1870=EDGE_LOOP('',(#8880,#8881,#8882));
#1871=EDGE_LOOP('',(#8883,#8884,#8885));
#1872=EDGE_LOOP('',(#8886,#8887,#8888));
#1873=EDGE_LOOP('',(#8889,#8890,#8891));
#1874=EDGE_LOOP('',(#8892));
#1875=EDGE_LOOP('',(#8893));
#1876=EDGE_LOOP('',(#8894,#8895,#8896,#8897,#8898));
#1877=EDGE_LOOP('',(#8899,#8900,#8901,#8902,#8903));
#1878=EDGE_LOOP('',(#8904,#8905,#8906,#8907,#8908));
#1879=EDGE_LOOP('',(#8909,#8910,#8911,#8912,#8913));
#1880=EDGE_LOOP('',(#8914,#8915,#8916,#8917,#8918,#8919,#8920,#8921));
#1881=EDGE_LOOP('',(#8922,#8923,#8924,#8925));
#1882=EDGE_LOOP('',(#8926,#8927,#8928,#8929));
#1883=EDGE_LOOP('',(#8930,#8931,#8932,#8933));
#1884=EDGE_LOOP('',(#8934,#8935,#8936,#8937,#8938));
#1885=EDGE_LOOP('',(#8939,#8940,#8941,#8942,#8943));
#1886=EDGE_LOOP('',(#8944,#8945,#8946,#8947,#8948));
#1887=EDGE_LOOP('',(#8949,#8950,#8951,#8952,#8953));
#1888=EDGE_LOOP('',(#8954,#8955,#8956,#8957,#8958));
#1889=EDGE_LOOP('',(#8959,#8960,#8961));
#1890=EDGE_LOOP('',(#8962,#8963,#8964));
#1891=EDGE_LOOP('',(#8965,#8966,#8967));
#1892=EDGE_LOOP('',(#8968,#8969,#8970));
#1893=EDGE_LOOP('',(#8971,#8972,#8973,#8974));
#1894=EDGE_LOOP('',(#8975,#8976,#8977,#8978));
#1895=EDGE_LOOP('',(#8979,#8980,#8981,#8982));
#1896=EDGE_LOOP('',(#8983,#8984,#8985,#8986));
#1897=EDGE_LOOP('',(#8987,#8988,#8989,#8990));
#1898=EDGE_LOOP('',(#8991,#8992,#8993,#8994));
#1899=EDGE_LOOP('',(#8995,#8996,#8997,#8998));
#1900=EDGE_LOOP('',(#8999,#9000,#9001,#9002));
#1901=EDGE_LOOP('',(#9003,#9004,#9005,#9006));
#1902=EDGE_LOOP('',(#9007,#9008,#9009,#9010));
#1903=EDGE_LOOP('',(#9011,#9012,#9013,#9014));
#1904=EDGE_LOOP('',(#9015,#9016,#9017,#9018));
#1905=EDGE_LOOP('',(#9019,#9020,#9021,#9022));
#1906=EDGE_LOOP('',(#9023,#9024,#9025,#9026));
#1907=EDGE_LOOP('',(#9027));
#1908=EDGE_LOOP('',(#9028,#9029,#9030,#9031));
#1909=EDGE_LOOP('',(#9032));
#1910=EDGE_LOOP('',(#9033));
#1911=EDGE_LOOP('',(#9034,#9035,#9036,#9037));
#1912=EDGE_LOOP('',(#9038));
#1913=EDGE_LOOP('',(#9039));
#1914=EDGE_LOOP('',(#9040));
#1915=EDGE_LOOP('',(#9041));
#1916=EDGE_LOOP('',(#9042));
#1917=EDGE_LOOP('',(#9043));
#1918=EDGE_LOOP('',(#9044));
#2353=LINE('',#15693,#3341);
#2354=LINE('',#15699,#3342);
#2355=LINE('',#15705,#3343);
#2356=LINE('',#15711,#3344);
#2357=LINE('',#15717,#3345);
#2358=LINE('',#15723,#3346);
#2359=LINE('',#15729,#3347);
#2360=LINE('',#15735,#3348);
#2361=LINE('',#15741,#3349);
#2362=LINE('',#15747,#3350);
#2363=LINE('',#15753,#3351);
#2364=LINE('',#15759,#3352);
#2365=LINE('',#15765,#3353);
#2366=LINE('',#15771,#3354);
#2367=LINE('',#15777,#3355);
#2368=LINE('',#15783,#3356);
#2369=LINE('',#15789,#3357);
#2370=LINE('',#15795,#3358);
#2371=LINE('',#15801,#3359);
#2372=LINE('',#15807,#3360);
#2373=LINE('',#15813,#3361);
#2374=LINE('',#15819,#3362);
#2375=LINE('',#15824,#3363);
#2376=LINE('',#15826,#3364);
#2377=LINE('',#15828,#3365);
#2378=LINE('',#15829,#3366);
#2379=LINE('',#15834,#3367);
#2380=LINE('',#15839,#3368);
#2381=LINE('',#15845,#3369);
#2382=LINE('',#15852,#3370);
#2383=LINE('',#15857,#3371);
#2384=LINE('',#15859,#3372);
#2385=LINE('',#15861,#3373);
#2386=LINE('',#15863,#3374);
#2387=LINE('',#15865,#3375);
#2388=LINE('',#15867,#3376);
#2389=LINE('',#15869,#3377);
#2390=LINE('',#15871,#3378);
#2391=LINE('',#15873,#3379);
#2392=LINE('',#15875,#3380);
#2393=LINE('',#15877,#3381);
#2394=LINE('',#15879,#3382);
#2395=LINE('',#15881,#3383);
#2396=LINE('',#15883,#3384);
#2397=LINE('',#15885,#3385);
#2398=LINE('',#15887,#3386);
#2399=LINE('',#15888,#3387);
#2400=LINE('',#15928,#3388);
#2401=LINE('',#15930,#3389);
#2402=LINE('',#15931,#3390);
#2403=LINE('',#16121,#3391);
#2404=LINE('',#16180,#3392);
#2405=LINE('',#16181,#3393);
#2406=LINE('',#16239,#3394);
#2407=LINE('',#16241,#3395);
#2408=LINE('',#16243,#3396);
#2409=LINE('',#16299,#3397);
#2410=LINE('',#16305,#3398);
#2411=LINE('',#16311,#3399);
#2412=LINE('',#16317,#3400);
#2413=LINE('',#16321,#3401);
#2414=LINE('',#16325,#3402);
#2415=LINE('',#16329,#3403);
#2416=LINE('',#16333,#3404);
#2417=LINE('',#16336,#3405);
#2418=LINE('',#16340,#3406);
#2419=LINE('',#16344,#3407);
#2420=LINE('',#16348,#3408);
#2421=LINE('',#16352,#3409);
#2422=LINE('',#16356,#3410);
#2423=LINE('',#16360,#3411);
#2424=LINE('',#16364,#3412);
#2425=LINE('',#16368,#3413);
#2426=LINE('',#16372,#3414);
#2427=LINE('',#16376,#3415);
#2428=LINE('',#16380,#3416);
#2429=LINE('',#16385,#3417);
#2430=LINE('',#16392,#3418);
#2431=LINE('',#16396,#3419);
#2432=LINE('',#16401,#3420);
#2433=LINE('',#16407,#3421);
#2434=LINE('',#16418,#3422);
#2435=LINE('',#16421,#3423);
#2436=LINE('',#16425,#3424);
#2437=LINE('',#16429,#3425);
#2438=LINE('',#16433,#3426);
#2439=LINE('',#16437,#3427);
#2440=LINE('',#16440,#3428);
#2441=LINE('',#16537,#3429);
#2442=LINE('',#16539,#3430);
#2443=LINE('',#16540,#3431);
#2444=LINE('',#16542,#3432);
#2445=LINE('',#16544,#3433);
#2446=LINE('',#16545,#3434);
#2447=LINE('',#16548,#3435);
#2448=LINE('',#16549,#3436);
#2449=LINE('',#16553,#3437);
#2450=LINE('',#16555,#3438);
#2451=LINE('',#16557,#3439);
#2452=LINE('',#16559,#3440);
#2453=LINE('',#16561,#3441);
#2454=LINE('',#16563,#3442);
#2455=LINE('',#16565,#3443);
#2456=LINE('',#16567,#3444);
#2457=LINE('',#16569,#3445);
#2458=LINE('',#16571,#3446);
#2459=LINE('',#16573,#3447);
#2460=LINE('',#16575,#3448);
#2461=LINE('',#16577,#3449);
#2462=LINE('',#16579,#3450);
#2463=LINE('',#16580,#3451);
#2464=LINE('',#16582,#3452);
#2465=LINE('',#16584,#3453);
#2466=LINE('',#16586,#3454);
#2467=LINE('',#16588,#3455);
#2468=LINE('',#16590,#3456);
#2469=LINE('',#16592,#3457);
#2470=LINE('',#16594,#3458);
#2471=LINE('',#16596,#3459);
#2472=LINE('',#16598,#3460);
#2473=LINE('',#16600,#3461);
#2474=LINE('',#16602,#3462);
#2475=LINE('',#16604,#3463);
#2476=LINE('',#16606,#3464);
#2477=LINE('',#16608,#3465);
#2478=LINE('',#16610,#3466);
#2479=LINE('',#16612,#3467);
#2480=LINE('',#16614,#3468);
#2481=LINE('',#16616,#3469);
#2482=LINE('',#16618,#3470);
#2483=LINE('',#16620,#3471);
#2484=LINE('',#16622,#3472);
#2485=LINE('',#16624,#3473);
#2486=LINE('',#16625,#3474);
#2487=LINE('',#16628,#3475);
#2488=LINE('',#16629,#3476);
#2489=LINE('',#16633,#3477);
#2490=LINE('',#16635,#3478);
#2491=LINE('',#16637,#3479);
#2492=LINE('',#16638,#3480);
#2493=LINE('',#16639,#3481);
#2494=LINE('',#16642,#3482);
#2495=LINE('',#16645,#3483);
#2496=LINE('',#16648,#3484);
#2497=LINE('',#16650,#3485);
#2498=LINE('',#16652,#3486);
#2499=LINE('',#16654,#3487);
#2500=LINE('',#16656,#3488);
#2501=LINE('',#16658,#3489);
#2502=LINE('',#16660,#3490);
#2503=LINE('',#16662,#3491);
#2504=LINE('',#16664,#3492);
#2505=LINE('',#16666,#3493);
#2506=LINE('',#16668,#3494);
#2507=LINE('',#16670,#3495);
#2508=LINE('',#16672,#3496);
#2509=LINE('',#16673,#3497);
#2510=LINE('',#16677,#3498);
#2511=LINE('',#16680,#3499);
#2512=LINE('',#16681,#3500);
#2513=LINE('',#16688,#3501);
#2514=LINE('',#16692,#3502);
#2515=LINE('',#16694,#3503);
#2516=LINE('',#16696,#3504);
#2517=LINE('',#16698,#3505);
#2518=LINE('',#16700,#3506);
#2519=LINE('',#16702,#3507);
#2520=LINE('',#16704,#3508);
#2521=LINE('',#16706,#3509);
#2522=LINE('',#16708,#3510);
#2523=LINE('',#16709,#3511);
#2524=LINE('',#16715,#3512);
#2525=LINE('',#16719,#3513);
#2526=LINE('',#16720,#3514);
#2527=LINE('',#16724,#3515);
#2528=LINE('',#16727,#3516);
#2529=LINE('',#16729,#3517);
#2530=LINE('',#16731,#3518);
#2531=LINE('',#16733,#3519);
#2532=LINE('',#16735,#3520);
#2533=LINE('',#16737,#3521);
#2534=LINE('',#16739,#3522);
#2535=LINE('',#16741,#3523);
#2536=LINE('',#16743,#3524);
#2537=LINE('',#16745,#3525);
#2538=LINE('',#16747,#3526);
#2539=LINE('',#16749,#3527);
#2540=LINE('',#16751,#3528);
#2541=LINE('',#16752,#3529);
#2542=LINE('',#16761,#3530);
#2543=LINE('',#16762,#3531);
#2544=LINE('',#16765,#3532);
#2545=LINE('',#16774,#3533);
#2546=LINE('',#16775,#3534);
#2547=LINE('',#16779,#3535);
#2548=LINE('',#16787,#3536);
#2549=LINE('',#16793,#3537);
#2550=LINE('',#16797,#3538);
#2551=LINE('',#16800,#3539);
#2552=LINE('',#16806,#3540);
#2553=LINE('',#16809,#3541);
#2554=LINE('',#16818,#3542);
#2555=LINE('',#16819,#3543);
#2556=LINE('',#16823,#3544);
#2557=LINE('',#16831,#3545);
#2558=LINE('',#16837,#3546);
#2559=LINE('',#16841,#3547);
#2560=LINE('',#16844,#3548);
#2561=LINE('',#16850,#3549);
#2562=LINE('',#16853,#3550);
#2563=LINE('',#16862,#3551);
#2564=LINE('',#16863,#3552);
#2565=LINE('',#16867,#3553);
#2566=LINE('',#16875,#3554);
#2567=LINE('',#16881,#3555);
#2568=LINE('',#16885,#3556);
#2569=LINE('',#16888,#3557);
#2570=LINE('',#16894,#3558);
#2571=LINE('',#16897,#3559);
#2572=LINE('',#16901,#3560);
#2573=LINE('',#16907,#3561);
#2574=LINE('',#16909,#3562);
#2575=LINE('',#16911,#3563);
#2576=LINE('',#16913,#3564);
#2577=LINE('',#16914,#3565);
#2578=LINE('',#16920,#3566);
#2579=LINE('',#16922,#3567);
#2580=LINE('',#16924,#3568);
#2581=LINE('',#16928,#3569);
#2582=LINE('',#16930,#3570);
#2583=LINE('',#16932,#3571);
#2584=LINE('',#16936,#3572);
#2585=LINE('',#16938,#3573);
#2586=LINE('',#16940,#3574);
#2587=LINE('',#16943,#3575);
#2588=LINE('',#16944,#3576);
#2589=LINE('',#16947,#3577);
#2590=LINE('',#16948,#3578);
#2591=LINE('',#16951,#3579);
#2592=LINE('',#16953,#3580);
#2593=LINE('',#16954,#3581);
#2594=LINE('',#16958,#3582);
#2595=LINE('',#16960,#3583);
#2596=LINE('',#16962,#3584);
#2597=LINE('',#16964,#3585);
#2598=LINE('',#16966,#3586);
#2599=LINE('',#16968,#3587);
#2600=LINE('',#16970,#3588);
#2601=LINE('',#16972,#3589);
#2602=LINE('',#16973,#3590);
#2603=LINE('',#16975,#3591);
#2604=LINE('',#16977,#3592);
#2605=LINE('',#16979,#3593);
#2606=LINE('',#16981,#3594);
#2607=LINE('',#16983,#3595);
#2608=LINE('',#16985,#3596);
#2609=LINE('',#16987,#3597);
#2610=LINE('',#16989,#3598);
#2611=LINE('',#16991,#3599);
#2612=LINE('',#16993,#3600);
#2613=LINE('',#16995,#3601);
#2614=LINE('',#16997,#3602);
#2615=LINE('',#16999,#3603);
#2616=LINE('',#17001,#3604);
#2617=LINE('',#17003,#3605);
#2618=LINE('',#17005,#3606);
#2619=LINE('',#17007,#3607);
#2620=LINE('',#17008,#3608);
#2621=LINE('',#17010,#3609);
#2622=LINE('',#17012,#3610);
#2623=LINE('',#17014,#3611);
#2624=LINE('',#17016,#3612);
#2625=LINE('',#17018,#3613);
#2626=LINE('',#17020,#3614);
#2627=LINE('',#17022,#3615);
#2628=LINE('',#17024,#3616);
#2629=LINE('',#17026,#3617);
#2630=LINE('',#17027,#3618);
#2631=LINE('',#17030,#3619);
#2632=LINE('',#17032,#3620);
#2633=LINE('',#17034,#3621);
#2634=LINE('',#17036,#3622);
#2635=LINE('',#17037,#3623);
#2636=LINE('',#17041,#3624);
#2637=LINE('',#17043,#3625);
#2638=LINE('',#17044,#3626);
#2639=LINE('',#17046,#3627);
#2640=LINE('',#17048,#3628);
#2641=LINE('',#17050,#3629);
#2642=LINE('',#17052,#3630);
#2643=LINE('',#17054,#3631);
#2644=LINE('',#17056,#3632);
#2645=LINE('',#17058,#3633);
#2646=LINE('',#17060,#3634);
#2647=LINE('',#17062,#3635);
#2648=LINE('',#17064,#3636);
#2649=LINE('',#17066,#3637);
#2650=LINE('',#17067,#3638);
#2651=LINE('',#17070,#3639);
#2652=LINE('',#17074,#3640);
#2653=LINE('',#17075,#3641);
#2654=LINE('',#17078,#3642);
#2655=LINE('',#17086,#3643);
#2656=LINE('',#17087,#3644);
#2657=LINE('',#17089,#3645);
#2658=LINE('',#17091,#3646);
#2659=LINE('',#17093,#3647);
#2660=LINE('',#17095,#3648);
#2661=LINE('',#17097,#3649);
#2662=LINE('',#17099,#3650);
#2663=LINE('',#17101,#3651);
#2664=LINE('',#17102,#3652);
#2665=LINE('',#17105,#3653);
#2666=LINE('',#17112,#3654);
#2667=LINE('',#17113,#3655);
#2668=LINE('',#17116,#3656);
#2669=LINE('',#17121,#3657);
#2670=LINE('',#17122,#3658);
#2671=LINE('',#17124,#3659);
#2672=LINE('',#17126,#3660);
#2673=LINE('',#17128,#3661);
#2674=LINE('',#17130,#3662);
#2675=LINE('',#17132,#3663);
#2676=LINE('',#17134,#3664);
#2677=LINE('',#17136,#3665);
#2678=LINE('',#17138,#3666);
#2679=LINE('',#17140,#3667);
#2680=LINE('',#17142,#3668);
#2681=LINE('',#17144,#3669);
#2682=LINE('',#17145,#3670);
#2683=LINE('',#17152,#3671);
#2684=LINE('',#17154,#3672);
#2685=LINE('',#17155,#3673);
#2686=LINE('',#17157,#3674);
#2687=LINE('',#17158,#3675);
#2688=LINE('',#17162,#3676);
#2689=LINE('',#17163,#3677);
#2690=LINE('',#17164,#3678);
#2691=LINE('',#17168,#3679);
#2692=LINE('',#17169,#3680);
#2693=LINE('',#17172,#3681);
#2694=LINE('',#17175,#3682);
#2695=LINE('',#17179,#3683);
#2696=LINE('',#17181,#3684);
#2697=LINE('',#17183,#3685);
#2698=LINE('',#17184,#3686);
#2699=LINE('',#17186,#3687);
#2700=LINE('',#17187,#3688);
#2701=LINE('',#17191,#3689);
#2702=LINE('',#17193,#3690);
#2703=LINE('',#17194,#3691);
#2704=LINE('',#17197,#3692);
#2705=LINE('',#17198,#3693);
#2706=LINE('',#17201,#3694);
#2707=LINE('',#17203,#3695);
#2708=LINE('',#17204,#3696);
#2709=LINE('',#17207,#3697);
#2710=LINE('',#17208,#3698);
#2711=LINE('',#17211,#3699);
#2712=LINE('',#17212,#3700);
#2713=LINE('',#17216,#3701);
#2714=LINE('',#17217,#3702);
#2715=LINE('',#17218,#3703);
#2716=LINE('',#17221,#3704);
#2717=LINE('',#17222,#3705);
#2718=LINE('',#17224,#3706);
#2719=LINE('',#17225,#3707);
#2720=LINE('',#17228,#3708);
#2721=LINE('',#17229,#3709);
#2722=LINE('',#17231,#3710);
#2723=LINE('',#17233,#3711);
#2724=LINE('',#17234,#3712);
#2725=LINE('',#17236,#3713);
#2726=LINE('',#17238,#3714);
#2727=LINE('',#17240,#3715);
#2728=LINE('',#17243,#3716);
#2729=LINE('',#17244,#3717);
#2730=LINE('',#17247,#3718);
#2731=LINE('',#17248,#3719);
#2732=LINE('',#17250,#3720);
#2733=LINE('',#17252,#3721);
#2734=LINE('',#17253,#3722);
#2735=LINE('',#17257,#3723);
#2736=LINE('',#17258,#3724);
#2737=LINE('',#17260,#3725);
#2738=LINE('',#17262,#3726);
#2739=LINE('',#17263,#3727);
#2740=LINE('',#17265,#3728);
#2741=LINE('',#17267,#3729);
#2742=LINE('',#17269,#3730);
#2743=LINE('',#17272,#3731);
#2744=LINE('',#17273,#3732);
#2745=LINE('',#17276,#3733);
#2746=LINE('',#17277,#3734);
#2747=LINE('',#17279,#3735);
#2748=LINE('',#17281,#3736);
#2749=LINE('',#17282,#3737);
#2750=LINE('',#17284,#3738);
#2751=LINE('',#17289,#3739);
#2752=LINE('',#17290,#3740);
#2753=LINE('',#17293,#3741);
#2754=LINE('',#17295,#3742);
#2755=LINE('',#17297,#3743);
#2756=LINE('',#17298,#3744);
#2757=LINE('',#17301,#3745);
#2758=LINE('',#17303,#3746);
#2759=LINE('',#17305,#3747);
#2760=LINE('',#17306,#3748);
#2761=LINE('',#17309,#3749);
#2762=LINE('',#17311,#3750);
#2763=LINE('',#17313,#3751);
#2764=LINE('',#17314,#3752);
#2765=LINE('',#17317,#3753);
#2766=LINE('',#17319,#3754);
#2767=LINE('',#17321,#3755);
#2768=LINE('',#17322,#3756);
#2769=LINE('',#17325,#3757);
#2770=LINE('',#17327,#3758);
#2771=LINE('',#17329,#3759);
#2772=LINE('',#17330,#3760);
#2773=LINE('',#17333,#3761);
#2774=LINE('',#17335,#3762);
#2775=LINE('',#17336,#3763);
#2776=LINE('',#17339,#3764);
#2777=LINE('',#17340,#3765);
#2778=LINE('',#17342,#3766);
#2779=LINE('',#17343,#3767);
#2780=LINE('',#17345,#3768);
#2781=LINE('',#17347,#3769);
#2782=LINE('',#17350,#3770);
#2783=LINE('',#17351,#3771);
#2784=LINE('',#17354,#3772);
#2785=LINE('',#17355,#3773);
#2786=LINE('',#17358,#3774);
#2787=LINE('',#17360,#3775);
#2788=LINE('',#17361,#3776);
#2789=LINE('',#17364,#3777);
#2790=LINE('',#17365,#3778);
#2791=LINE('',#17367,#3779);
#2792=LINE('',#17370,#3780);
#2793=LINE('',#17371,#3781);
#2794=LINE('',#17374,#3782);
#2795=LINE('',#17376,#3783);
#2796=LINE('',#17377,#3784);
#2797=LINE('',#17380,#3785);
#2798=LINE('',#17381,#3786);
#2799=LINE('',#17384,#3787);
#2800=LINE('',#17385,#3788);
#2801=LINE('',#17388,#3789);
#2802=LINE('',#17389,#3790);
#2803=LINE('',#17391,#3791);
#2804=LINE('',#17393,#3792);
#2805=LINE('',#17395,#3793);
#2806=LINE('',#17397,#3794);
#2807=LINE('',#17434,#3795);
#2808=LINE('',#17437,#3796);
#2809=LINE('',#17438,#3797);
#2810=LINE('',#17440,#3798);
#2811=LINE('',#17442,#3799);
#2812=LINE('',#17444,#3800);
#2813=LINE('',#17446,#3801);
#2814=LINE('',#17449,#3802);
#2815=LINE('',#17450,#3803);
#2816=LINE('',#17453,#3804);
#2817=LINE('',#17454,#3805);
#2818=LINE('',#17456,#3806);
#2819=LINE('',#17458,#3807);
#2820=LINE('',#17459,#3808);
#2821=LINE('',#17461,#3809);
#2822=LINE('',#17463,#3810);
#2823=LINE('',#17465,#3811);
#2824=LINE('',#17468,#3812);
#2825=LINE('',#17469,#3813);
#2826=LINE('',#17472,#3814);
#2827=LINE('',#17473,#3815);
#2828=LINE('',#17476,#3816);
#2829=LINE('',#17477,#3817);
#2830=LINE('',#17480,#3818);
#2831=LINE('',#17481,#3819);
#2832=LINE('',#17483,#3820);
#2833=LINE('',#17485,#3821);
#2834=LINE('',#17488,#3822);
#2835=LINE('',#17489,#3823);
#2836=LINE('',#17491,#3824);
#2837=LINE('',#17493,#3825);
#2838=LINE('',#17494,#3826);
#2839=LINE('',#17497,#3827);
#2840=LINE('',#17498,#3828);
#2841=LINE('',#17501,#3829);
#2842=LINE('',#17503,#3830);
#2843=LINE('',#17504,#3831);
#2844=LINE('',#17507,#3832);
#2845=LINE('',#17508,#3833);
#2846=LINE('',#17511,#3834);
#2847=LINE('',#17512,#3835);
#2848=LINE('',#17515,#3836);
#2849=LINE('',#17516,#3837);
#2850=LINE('',#17519,#3838);
#2851=LINE('',#17520,#3839);
#2852=LINE('',#17525,#3840);
#2853=LINE('',#17527,#3841);
#2854=LINE('',#17528,#3842);
#2855=LINE('',#17532,#3843);
#2856=LINE('',#17535,#3844);
#2857=LINE('',#17537,#3845);
#2858=LINE('',#17539,#3846);
#2859=LINE('',#17540,#3847);
#2860=LINE('',#17542,#3848);
#2861=LINE('',#17543,#3849);
#2862=LINE('',#17547,#3850);
#2863=LINE('',#17548,#3851);
#2864=LINE('',#17551,#3852);
#2865=LINE('',#17553,#3853);
#2866=LINE('',#17555,#3854);
#2867=LINE('',#17556,#3855);
#2868=LINE('',#17560,#3856);
#2869=LINE('',#17561,#3857);
#2870=LINE('',#17563,#3858);
#2871=LINE('',#17564,#3859);
#2872=LINE('',#17567,#3860);
#2873=LINE('',#17569,#3861);
#2874=LINE('',#17570,#3862);
#2875=LINE('',#17573,#3863);
#2876=LINE('',#17575,#3864);
#2877=LINE('',#17577,#3865);
#2878=LINE('',#17578,#3866);
#2879=LINE('',#17582,#3867);
#2880=LINE('',#17583,#3868);
#2881=LINE('',#17585,#3869);
#2882=LINE('',#17586,#3870);
#2883=LINE('',#17589,#3871);
#2884=LINE('',#17591,#3872);
#2885=LINE('',#17592,#3873);
#2886=LINE('',#17594,#3874);
#2887=LINE('',#17596,#3875);
#2888=LINE('',#17598,#3876);
#2889=LINE('',#17601,#3877);
#2890=LINE('',#17602,#3878);
#2891=LINE('',#17605,#3879);
#2892=LINE('',#17607,#3880);
#2893=LINE('',#17608,#3881);
#2894=LINE('',#17611,#3882);
#2895=LINE('',#17612,#3883);
#2896=LINE('',#17615,#3884);
#2897=LINE('',#17616,#3885);
#2898=LINE('',#17619,#3886);
#2899=LINE('',#17620,#3887);
#2900=LINE('',#17622,#3888);
#2901=LINE('',#17624,#3889);
#2902=LINE('',#17626,#3890);
#2903=LINE('',#17629,#3891);
#2904=LINE('',#17631,#3892);
#2905=LINE('',#17634,#3893);
#2906=LINE('',#17635,#3894);
#2907=LINE('',#17638,#3895);
#2908=LINE('',#17640,#3896);
#2909=LINE('',#17641,#3897);
#2910=LINE('',#17643,#3898);
#2911=LINE('',#17644,#3899);
#2912=LINE('',#17646,#3900);
#2913=LINE('',#17647,#3901);
#2914=LINE('',#17648,#3902);
#2915=LINE('',#17651,#3903);
#2916=LINE('',#17652,#3904);
#2917=LINE('',#17653,#3905);
#2918=LINE('',#17656,#3906);
#2919=LINE('',#17658,#3907);
#2920=LINE('',#17661,#3908);
#2921=LINE('',#17663,#3909);
#2922=LINE('',#17665,#3910);
#2923=LINE('',#17666,#3911);
#2924=LINE('',#17669,#3912);
#2925=LINE('',#17672,#3913);
#2926=LINE('',#17676,#3914);
#2927=LINE('',#17679,#3915);
#2928=LINE('',#17682,#3916);
#2929=LINE('',#17683,#3917);
#2930=LINE('',#17685,#3918);
#2931=LINE('',#17686,#3919);
#2932=LINE('',#17688,#3920);
#2933=LINE('',#17691,#3921);
#2934=LINE('',#17694,#3922);
#2935=LINE('',#17695,#3923);
#2936=LINE('',#17697,#3924);
#2937=LINE('',#18413,#3925);
#2938=LINE('',#18416,#3926);
#2939=LINE('',#18419,#3927);
#2940=LINE('',#18422,#3928);
#2941=LINE('',#18424,#3929);
#2942=LINE('',#18426,#3930);
#2943=LINE('',#18427,#3931);
#2944=LINE('',#18430,#3932);
#2945=LINE('',#18433,#3933);
#2946=LINE('',#18434,#3934);
#2947=LINE('',#18436,#3935);
#2948=LINE('',#18437,#3936);
#2949=LINE('',#18439,#3937);
#2950=LINE('',#18440,#3938);
#2951=LINE('',#18450,#3939);
#2952=LINE('',#18451,#3940);
#2953=LINE('',#18452,#3941);
#2954=LINE('',#18455,#3942);
#2955=LINE('',#18456,#3943);
#2956=LINE('',#18459,#3944);
#2957=LINE('',#18460,#3945);
#2958=LINE('',#18462,#3946);
#2959=LINE('',#18730,#3947);
#2960=LINE('',#18731,#3948);
#2961=LINE('',#18732,#3949);
#2962=LINE('',#18735,#3950);
#2963=LINE('',#18736,#3951);
#2964=LINE('',#18739,#3952);
#2965=LINE('',#18740,#3953);
#2966=LINE('',#18742,#3954);
#3341=VECTOR('',#12515,5.5);
#3342=VECTOR('',#12522,14.);
#3343=VECTOR('',#12529,1.35);
#3344=VECTOR('',#12536,1.35);
#3345=VECTOR('',#12543,1.35);
#3346=VECTOR('',#12550,1.35);
#3347=VECTOR('',#12557,1.35);
#3348=VECTOR('',#12564,1.35);
#3349=VECTOR('',#12571,1.35);
#3350=VECTOR('',#12578,1.35);
#3351=VECTOR('',#12585,1.35);
#3352=VECTOR('',#12592,1.35);
#3353=VECTOR('',#12599,1.35);
#3354=VECTOR('',#12606,1.35);
#3355=VECTOR('',#12613,5.);
#3356=VECTOR('',#12620,7.5);
#3357=VECTOR('',#12627,2.75);
#3358=VECTOR('',#12634,5.);
#3359=VECTOR('',#12641,7.25);
#3360=VECTOR('',#12648,14.);
#3361=VECTOR('',#12655,4.75);
#3362=VECTOR('',#12662,2.75);
#3363=VECTOR('',#12667,1000.);
#3364=VECTOR('',#12668,1000.);
#3365=VECTOR('',#12669,1000.);
#3366=VECTOR('',#12670,1000.);
#3367=VECTOR('',#12675,1000.);
#3368=VECTOR('',#12680,1000.);
#3369=VECTOR('',#12687,1000.);
#3370=VECTOR('',#12696,1000.);
#3371=VECTOR('',#12703,1000.);
#3372=VECTOR('',#12704,1000.);
#3373=VECTOR('',#12705,1000.);
#3374=VECTOR('',#12706,1000.);
#3375=VECTOR('',#12707,1000.);
#3376=VECTOR('',#12708,1000.);
#3377=VECTOR('',#12709,1000.);
#3378=VECTOR('',#12710,1000.);
#3379=VECTOR('',#12711,1000.);
#3380=VECTOR('',#12712,1000.);
#3381=VECTOR('',#12713,1000.);
#3382=VECTOR('',#12714,1000.);
#3383=VECTOR('',#12715,1000.);
#3384=VECTOR('',#12716,1000.);
#3385=VECTOR('',#12717,1000.);
#3386=VECTOR('',#12718,1000.);
#3387=VECTOR('',#12719,1000.);
#3388=VECTOR('',#12730,1000.);
#3389=VECTOR('',#12731,1000.);
#3390=VECTOR('',#12732,1000.);
#3391=VECTOR('',#12737,1000.);
#3392=VECTOR('',#12738,1000.);
#3393=VECTOR('',#12739,1000.);
#3394=VECTOR('',#12744,1000.);
#3395=VECTOR('',#12745,1000.);
#3396=VECTOR('',#12746,1000.);
#3397=VECTOR('',#12749,1000.);
#3398=VECTOR('',#12756,1000.);
#3399=VECTOR('',#12763,1000.);
#3400=VECTOR('',#12770,1000.);
#3401=VECTOR('',#12773,1000.);
#3402=VECTOR('',#12776,1000.);
#3403=VECTOR('',#12779,1000.);
#3404=VECTOR('',#12782,1000.);
#3405=VECTOR('',#12785,1000.);
#3406=VECTOR('',#12788,1000.);
#3407=VECTOR('',#12791,1000.);
#3408=VECTOR('',#12794,1000.);
#3409=VECTOR('',#12797,1000.);
#3410=VECTOR('',#12800,1000.);
#3411=VECTOR('',#12803,1000.);
#3412=VECTOR('',#12806,1000.);
#3413=VECTOR('',#12809,1000.);
#3414=VECTOR('',#12812,1000.);
#3415=VECTOR('',#12815,1000.);
#3416=VECTOR('',#12818,1000.);
#3417=VECTOR('',#12823,1000.);
#3418=VECTOR('',#12832,1000.);
#3419=VECTOR('',#12837,1000.);
#3420=VECTOR('',#12842,1000.);
#3421=VECTOR('',#12849,1000.);
#3422=VECTOR('',#12864,1000.);
#3423=VECTOR('',#12867,1000.);
#3424=VECTOR('',#12872,1000.);
#3425=VECTOR('',#12875,1000.);
#3426=VECTOR('',#12878,1000.);
#3427=VECTOR('',#12881,1000.);
#3428=VECTOR('',#12884,1000.);
#3429=VECTOR('',#12897,1000.);
#3430=VECTOR('',#12898,1000.);
#3431=VECTOR('',#12899,1000.);
#3432=VECTOR('',#12900,1000.);
#3433=VECTOR('',#12901,1000.);
#3434=VECTOR('',#12902,1000.);
#3435=VECTOR('',#12905,1000.);
#3436=VECTOR('',#12906,1000.);
#3437=VECTOR('',#12909,1000.);
#3438=VECTOR('',#12910,1000.);
#3439=VECTOR('',#12911,1000.);
#3440=VECTOR('',#12912,1000.);
#3441=VECTOR('',#12913,1000.);
#3442=VECTOR('',#12914,1000.);
#3443=VECTOR('',#12915,1000.);
#3444=VECTOR('',#12916,1000.);
#3445=VECTOR('',#12917,1000.);
#3446=VECTOR('',#12918,1000.);
#3447=VECTOR('',#12919,1000.);
#3448=VECTOR('',#12920,1000.);
#3449=VECTOR('',#12921,1000.);
#3450=VECTOR('',#12922,1000.);
#3451=VECTOR('',#12923,1000.);
#3452=VECTOR('',#12924,1000.);
#3453=VECTOR('',#12925,1000.);
#3454=VECTOR('',#12926,1000.);
#3455=VECTOR('',#12927,1000.);
#3456=VECTOR('',#12928,1000.);
#3457=VECTOR('',#12929,1000.);
#3458=VECTOR('',#12930,1000.);
#3459=VECTOR('',#12931,1000.);
#3460=VECTOR('',#12932,1000.);
#3461=VECTOR('',#12933,1000.);
#3462=VECTOR('',#12934,1000.);
#3463=VECTOR('',#12935,1000.);
#3464=VECTOR('',#12936,1000.);
#3465=VECTOR('',#12937,1000.);
#3466=VECTOR('',#12938,1000.);
#3467=VECTOR('',#12939,1000.);
#3468=VECTOR('',#12940,1000.);
#3469=VECTOR('',#12941,1000.);
#3470=VECTOR('',#12942,1000.);
#3471=VECTOR('',#12943,1000.);
#3472=VECTOR('',#12944,1000.);
#3473=VECTOR('',#12945,1000.);
#3474=VECTOR('',#12946,1000.);
#3475=VECTOR('',#12949,1000.);
#3476=VECTOR('',#12950,1000.);
#3477=VECTOR('',#12953,1000.);
#3478=VECTOR('',#12954,1000.);
#3479=VECTOR('',#12955,1000.);
#3480=VECTOR('',#12956,1000.);
#3481=VECTOR('',#12957,1000.);
#3482=VECTOR('',#12960,1000.);
#3483=VECTOR('',#12963,1000.);
#3484=VECTOR('',#12966,1000.);
#3485=VECTOR('',#12967,1000.);
#3486=VECTOR('',#12968,1000.);
#3487=VECTOR('',#12969,1000.);
#3488=VECTOR('',#12970,1000.);
#3489=VECTOR('',#12971,1000.);
#3490=VECTOR('',#12972,1000.);
#3491=VECTOR('',#12973,1000.);
#3492=VECTOR('',#12974,1000.);
#3493=VECTOR('',#12975,1000.);
#3494=VECTOR('',#12976,1000.);
#3495=VECTOR('',#12977,1000.);
#3496=VECTOR('',#12978,1000.);
#3497=VECTOR('',#12979,1000.);
#3498=VECTOR('',#12984,1000.);
#3499=VECTOR('',#12987,1000.);
#3500=VECTOR('',#12988,1000.);
#3501=VECTOR('',#12995,1000.);
#3502=VECTOR('',#13000,1000.);
#3503=VECTOR('',#13001,1000.);
#3504=VECTOR('',#13002,1000.);
#3505=VECTOR('',#13003,1000.);
#3506=VECTOR('',#13004,1000.);
#3507=VECTOR('',#13005,1000.);
#3508=VECTOR('',#13006,1000.);
#3509=VECTOR('',#13007,1000.);
#3510=VECTOR('',#13008,1000.);
#3511=VECTOR('',#13009,1000.);
#3512=VECTOR('',#13016,1000.);
#3513=VECTOR('',#13021,1000.);
#3514=VECTOR('',#13022,1000.);
#3515=VECTOR('',#13027,1000.);
#3516=VECTOR('',#13030,1000.);
#3517=VECTOR('',#13031,1000.);
#3518=VECTOR('',#13032,1000.);
#3519=VECTOR('',#13033,1000.);
#3520=VECTOR('',#13034,1000.);
#3521=VECTOR('',#13035,1000.);
#3522=VECTOR('',#13036,1000.);
#3523=VECTOR('',#13037,1000.);
#3524=VECTOR('',#13038,1000.);
#3525=VECTOR('',#13039,1000.);
#3526=VECTOR('',#13040,1000.);
#3527=VECTOR('',#13041,1000.);
#3528=VECTOR('',#13042,1000.);
#3529=VECTOR('',#13043,1000.);
#3530=VECTOR('',#13056,1000.);
#3531=VECTOR('',#13057,1000.);
#3532=VECTOR('',#13060,1000.);
#3533=VECTOR('',#13065,1000.);
#3534=VECTOR('',#13066,1000.);
#3535=VECTOR('',#13071,1000.);
#3536=VECTOR('',#13074,1000.);
#3537=VECTOR('',#13075,1000.);
#3538=VECTOR('',#13080,1000.);
#3539=VECTOR('',#13083,1000.);
#3540=VECTOR('',#13084,1000.);
#3541=VECTOR('',#13087,1000.);
#3542=VECTOR('',#13092,1000.);
#3543=VECTOR('',#13093,1000.);
#3544=VECTOR('',#13098,1000.);
#3545=VECTOR('',#13101,1000.);
#3546=VECTOR('',#13102,1000.);
#3547=VECTOR('',#13107,1000.);
#3548=VECTOR('',#13110,1000.);
#3549=VECTOR('',#13111,1000.);
#3550=VECTOR('',#13114,1000.);
#3551=VECTOR('',#13119,1000.);
#3552=VECTOR('',#13120,1000.);
#3553=VECTOR('',#13125,1000.);
#3554=VECTOR('',#13128,1000.);
#3555=VECTOR('',#13129,1000.);
#3556=VECTOR('',#13134,1000.);
#3557=VECTOR('',#13137,1000.);
#3558=VECTOR('',#13138,1000.);
#3559=VECTOR('',#13141,1000.);
#3560=VECTOR('',#13146,1000.);
#3561=VECTOR('',#13155,1000.);
#3562=VECTOR('',#13156,1000.);
#3563=VECTOR('',#13157,1000.);
#3564=VECTOR('',#13158,1000.);
#3565=VECTOR('',#13159,1000.);
#3566=VECTOR('',#13164,1000.);
#3567=VECTOR('',#13165,1000.);
#3568=VECTOR('',#13166,1000.);
#3569=VECTOR('',#13169,1000.);
#3570=VECTOR('',#13170,1000.);
#3571=VECTOR('',#13171,1000.);
#3572=VECTOR('',#13174,1000.);
#3573=VECTOR('',#13175,1000.);
#3574=VECTOR('',#13176,1000.);
#3575=VECTOR('',#13179,1000.);
#3576=VECTOR('',#13180,1000.);
#3577=VECTOR('',#13183,1000.);
#3578=VECTOR('',#13184,1000.);
#3579=VECTOR('',#13187,1000.);
#3580=VECTOR('',#13188,1000.);
#3581=VECTOR('',#13189,1000.);
#3582=VECTOR('',#13192,1000.);
#3583=VECTOR('',#13193,1000.);
#3584=VECTOR('',#13194,1000.);
#3585=VECTOR('',#13195,1000.);
#3586=VECTOR('',#13196,1000.);
#3587=VECTOR('',#13197,1000.);
#3588=VECTOR('',#13198,1000.);
#3589=VECTOR('',#13199,1000.);
#3590=VECTOR('',#13200,1000.);
#3591=VECTOR('',#13201,1000.);
#3592=VECTOR('',#13202,1000.);
#3593=VECTOR('',#13203,1000.);
#3594=VECTOR('',#13204,1000.);
#3595=VECTOR('',#13205,1000.);
#3596=VECTOR('',#13206,1000.);
#3597=VECTOR('',#13207,1000.);
#3598=VECTOR('',#13208,1000.);
#3599=VECTOR('',#13209,1000.);
#3600=VECTOR('',#13210,1000.);
#3601=VECTOR('',#13211,1000.);
#3602=VECTOR('',#13212,1000.);
#3603=VECTOR('',#13213,1000.);
#3604=VECTOR('',#13214,1000.);
#3605=VECTOR('',#13215,1000.);
#3606=VECTOR('',#13216,1000.);
#3607=VECTOR('',#13217,1000.);
#3608=VECTOR('',#13218,1000.);
#3609=VECTOR('',#13219,1000.);
#3610=VECTOR('',#13220,1000.);
#3611=VECTOR('',#13221,1000.);
#3612=VECTOR('',#13222,1000.);
#3613=VECTOR('',#13223,1000.);
#3614=VECTOR('',#13224,1000.);
#3615=VECTOR('',#13225,1000.);
#3616=VECTOR('',#13226,1000.);
#3617=VECTOR('',#13227,1000.);
#3618=VECTOR('',#13228,1000.);
#3619=VECTOR('',#13231,1000.);
#3620=VECTOR('',#13232,1000.);
#3621=VECTOR('',#13233,1000.);
#3622=VECTOR('',#13234,1000.);
#3623=VECTOR('',#13235,1000.);
#3624=VECTOR('',#13238,1000.);
#3625=VECTOR('',#13239,1000.);
#3626=VECTOR('',#13240,1000.);
#3627=VECTOR('',#13241,1000.);
#3628=VECTOR('',#13242,1000.);
#3629=VECTOR('',#13243,1000.);
#3630=VECTOR('',#13244,1000.);
#3631=VECTOR('',#13245,1000.);
#3632=VECTOR('',#13246,1000.);
#3633=VECTOR('',#13247,1000.);
#3634=VECTOR('',#13248,1000.);
#3635=VECTOR('',#13249,1000.);
#3636=VECTOR('',#13250,1000.);
#3637=VECTOR('',#13251,1000.);
#3638=VECTOR('',#13252,1000.);
#3639=VECTOR('',#13255,1000.);
#3640=VECTOR('',#13260,1000.);
#3641=VECTOR('',#13261,1000.);
#3642=VECTOR('',#13264,1000.);
#3643=VECTOR('',#13273,1000.);
#3644=VECTOR('',#13274,1000.);
#3645=VECTOR('',#13275,1000.);
#3646=VECTOR('',#13276,1000.);
#3647=VECTOR('',#13277,1000.);
#3648=VECTOR('',#13278,1000.);
#3649=VECTOR('',#13279,1000.);
#3650=VECTOR('',#13280,1000.);
#3651=VECTOR('',#13281,1000.);
#3652=VECTOR('',#13282,1000.);
#3653=VECTOR('',#13285,1000.);
#3654=VECTOR('',#13294,1000.);
#3655=VECTOR('',#13295,1000.);
#3656=VECTOR('',#13298,1000.);
#3657=VECTOR('',#13303,1000.);
#3658=VECTOR('',#13304,1000.);
#3659=VECTOR('',#13305,1000.);
#3660=VECTOR('',#13306,1000.);
#3661=VECTOR('',#13307,1000.);
#3662=VECTOR('',#13308,1000.);
#3663=VECTOR('',#13309,1000.);
#3664=VECTOR('',#13310,1000.);
#3665=VECTOR('',#13311,1000.);
#3666=VECTOR('',#13312,1000.);
#3667=VECTOR('',#13313,1000.);
#3668=VECTOR('',#13314,1000.);
#3669=VECTOR('',#13315,1000.);
#3670=VECTOR('',#13316,1000.);
#3671=VECTOR('',#13327,1000.);
#3672=VECTOR('',#13328,1000.);
#3673=VECTOR('',#13329,1000.);
#3674=VECTOR('',#13332,1000.);
#3675=VECTOR('',#13333,1000.);
#3676=VECTOR('',#13338,1000.);
#3677=VECTOR('',#13339,1000.);
#3678=VECTOR('',#13340,1000.);
#3679=VECTOR('',#13343,1000.);
#3680=VECTOR('',#13344,1000.);
#3681=VECTOR('',#13347,1000.);
#3682=VECTOR('',#13350,1000.);
#3683=VECTOR('',#13355,1000.);
#3684=VECTOR('',#13356,1000.);
#3685=VECTOR('',#13357,1000.);
#3686=VECTOR('',#13358,1000.);
#3687=VECTOR('',#13361,1000.);
#3688=VECTOR('',#13362,1000.);
#3689=VECTOR('',#13367,1000.);
#3690=VECTOR('',#13368,1000.);
#3691=VECTOR('',#13369,1000.);
#3692=VECTOR('',#13372,1000.);
#3693=VECTOR('',#13373,1000.);
#3694=VECTOR('',#13376,1000.);
#3695=VECTOR('',#13377,1000.);
#3696=VECTOR('',#13378,1000.);
#3697=VECTOR('',#13381,1000.);
#3698=VECTOR('',#13382,1000.);
#3699=VECTOR('',#13385,1000.);
#3700=VECTOR('',#13386,1000.);
#3701=VECTOR('',#13389,1000.);
#3702=VECTOR('',#13390,1000.);
#3703=VECTOR('',#13391,1000.);
#3704=VECTOR('',#13394,1000.);
#3705=VECTOR('',#13395,1000.);
#3706=VECTOR('',#13396,1000.);
#3707=VECTOR('',#13397,1000.);
#3708=VECTOR('',#13400,1000.);
#3709=VECTOR('',#13401,1000.);
#3710=VECTOR('',#13404,1000.);
#3711=VECTOR('',#13405,1000.);
#3712=VECTOR('',#13406,1000.);
#3713=VECTOR('',#13409,1000.);
#3714=VECTOR('',#13412,1000.);
#3715=VECTOR('',#13415,1000.);
#3716=VECTOR('',#13418,1000.);
#3717=VECTOR('',#13419,1000.);
#3718=VECTOR('',#13422,1000.);
#3719=VECTOR('',#13423,1000.);
#3720=VECTOR('',#13426,1000.);
#3721=VECTOR('',#13427,1000.);
#3722=VECTOR('',#13428,1000.);
#3723=VECTOR('',#13433,1000.);
#3724=VECTOR('',#13434,1000.);
#3725=VECTOR('',#13437,1000.);
#3726=VECTOR('',#13438,1000.);
#3727=VECTOR('',#13439,1000.);
#3728=VECTOR('',#13442,1000.);
#3729=VECTOR('',#13445,1000.);
#3730=VECTOR('',#13448,1000.);
#3731=VECTOR('',#13451,1000.);
#3732=VECTOR('',#13452,1000.);
#3733=VECTOR('',#13455,1000.);
#3734=VECTOR('',#13456,1000.);
#3735=VECTOR('',#13459,1000.);
#3736=VECTOR('',#13460,1000.);
#3737=VECTOR('',#13461,1000.);
#3738=VECTOR('',#13464,1000.);
#3739=VECTOR('',#13471,1000.);
#3740=VECTOR('',#13472,1000.);
#3741=VECTOR('',#13475,1000.);
#3742=VECTOR('',#13476,1000.);
#3743=VECTOR('',#13477,1000.);
#3744=VECTOR('',#13478,1000.);
#3745=VECTOR('',#13481,1000.);
#3746=VECTOR('',#13482,1000.);
#3747=VECTOR('',#13483,1000.);
#3748=VECTOR('',#13484,1000.);
#3749=VECTOR('',#13487,1000.);
#3750=VECTOR('',#13488,1000.);
#3751=VECTOR('',#13489,1000.);
#3752=VECTOR('',#13490,1000.);
#3753=VECTOR('',#13493,1000.);
#3754=VECTOR('',#13494,1000.);
#3755=VECTOR('',#13495,1000.);
#3756=VECTOR('',#13496,1000.);
#3757=VECTOR('',#13499,1000.);
#3758=VECTOR('',#13500,1000.);
#3759=VECTOR('',#13501,1000.);
#3760=VECTOR('',#13502,1000.);
#3761=VECTOR('',#13505,1000.);
#3762=VECTOR('',#13506,1000.);
#3763=VECTOR('',#13507,1000.);
#3764=VECTOR('',#13510,1000.);
#3765=VECTOR('',#13511,1000.);
#3766=VECTOR('',#13514,1000.);
#3767=VECTOR('',#13515,1000.);
#3768=VECTOR('',#13518,1000.);
#3769=VECTOR('',#13521,1000.);
#3770=VECTOR('',#13524,1000.);
#3771=VECTOR('',#13525,1000.);
#3772=VECTOR('',#13528,1000.);
#3773=VECTOR('',#13529,1000.);
#3774=VECTOR('',#13532,1000.);
#3775=VECTOR('',#13533,1000.);
#3776=VECTOR('',#13534,1000.);
#3777=VECTOR('',#13537,1000.);
#3778=VECTOR('',#13538,1000.);
#3779=VECTOR('',#13541,1000.);
#3780=VECTOR('',#13544,1000.);
#3781=VECTOR('',#13545,1000.);
#3782=VECTOR('',#13548,1000.);
#3783=VECTOR('',#13549,1000.);
#3784=VECTOR('',#13550,1000.);
#3785=VECTOR('',#13553,1000.);
#3786=VECTOR('',#13554,1000.);
#3787=VECTOR('',#13557,1000.);
#3788=VECTOR('',#13558,1000.);
#3789=VECTOR('',#13561,1000.);
#3790=VECTOR('',#13562,1000.);
#3791=VECTOR('',#13565,1000.);
#3792=VECTOR('',#13568,1000.);
#3793=VECTOR('',#13571,1000.);
#3794=VECTOR('',#13574,1000.);
#3795=VECTOR('',#13647,1000.);
#3796=VECTOR('',#13650,1000.);
#3797=VECTOR('',#13651,1000.);
#3798=VECTOR('',#13654,1000.);
#3799=VECTOR('',#13657,1000.);
#3800=VECTOR('',#13660,1000.);
#3801=VECTOR('',#13663,1000.);
#3802=VECTOR('',#13666,1000.);
#3803=VECTOR('',#13667,1000.);
#3804=VECTOR('',#13670,1000.);
#3805=VECTOR('',#13671,1000.);
#3806=VECTOR('',#13674,1000.);
#3807=VECTOR('',#13675,1000.);
#3808=VECTOR('',#13676,1000.);
#3809=VECTOR('',#13679,1000.);
#3810=VECTOR('',#13682,1000.);
#3811=VECTOR('',#13685,1000.);
#3812=VECTOR('',#13688,1000.);
#3813=VECTOR('',#13689,1000.);
#3814=VECTOR('',#13692,1000.);
#3815=VECTOR('',#13693,1000.);
#3816=VECTOR('',#13696,1000.);
#3817=VECTOR('',#13697,1000.);
#3818=VECTOR('',#13700,1000.);
#3819=VECTOR('',#13701,1000.);
#3820=VECTOR('',#13704,1000.);
#3821=VECTOR('',#13707,1000.);
#3822=VECTOR('',#13710,1000.);
#3823=VECTOR('',#13711,1000.);
#3824=VECTOR('',#13714,1000.);
#3825=VECTOR('',#13715,1000.);
#3826=VECTOR('',#13716,1000.);
#3827=VECTOR('',#13719,1000.);
#3828=VECTOR('',#13720,1000.);
#3829=VECTOR('',#13723,1000.);
#3830=VECTOR('',#13724,1000.);
#3831=VECTOR('',#13725,1000.);
#3832=VECTOR('',#13728,1000.);
#3833=VECTOR('',#13729,1000.);
#3834=VECTOR('',#13732,1000.);
#3835=VECTOR('',#13733,1000.);
#3836=VECTOR('',#13736,1000.);
#3837=VECTOR('',#13737,1000.);
#3838=VECTOR('',#13740,1000.);
#3839=VECTOR('',#13741,1000.);
#3840=VECTOR('',#13746,1000.);
#3841=VECTOR('',#13747,1000.);
#3842=VECTOR('',#13748,1000.);
#3843=VECTOR('',#13753,1000.);
#3844=VECTOR('',#13756,1000.);
#3845=VECTOR('',#13757,1000.);
#3846=VECTOR('',#13758,1000.);
#3847=VECTOR('',#13759,1000.);
#3848=VECTOR('',#13762,1000.);
#3849=VECTOR('',#13763,1000.);
#3850=VECTOR('',#13768,1000.);
#3851=VECTOR('',#13769,1000.);
#3852=VECTOR('',#13772,1000.);
#3853=VECTOR('',#13773,1000.);
#3854=VECTOR('',#13774,1000.);
#3855=VECTOR('',#13775,1000.);
#3856=VECTOR('',#13778,1000.);
#3857=VECTOR('',#13779,1000.);
#3858=VECTOR('',#13780,1000.);
#3859=VECTOR('',#13781,1000.);
#3860=VECTOR('',#13784,1000.);
#3861=VECTOR('',#13785,1000.);
#3862=VECTOR('',#13786,1000.);
#3863=VECTOR('',#13789,1000.);
#3864=VECTOR('',#13790,1000.);
#3865=VECTOR('',#13791,1000.);
#3866=VECTOR('',#13792,1000.);
#3867=VECTOR('',#13795,1000.);
#3868=VECTOR('',#13796,1000.);
#3869=VECTOR('',#13797,1000.);
#3870=VECTOR('',#13798,1000.);
#3871=VECTOR('',#13801,1000.);
#3872=VECTOR('',#13802,1000.);
#3873=VECTOR('',#13803,1000.);
#3874=VECTOR('',#13806,1000.);
#3875=VECTOR('',#13809,1000.);
#3876=VECTOR('',#13812,1000.);
#3877=VECTOR('',#13815,1000.);
#3878=VECTOR('',#13816,1000.);
#3879=VECTOR('',#13819,1000.);
#3880=VECTOR('',#13820,1000.);
#3881=VECTOR('',#13821,1000.);
#3882=VECTOR('',#13824,1000.);
#3883=VECTOR('',#13825,1000.);
#3884=VECTOR('',#13828,1000.);
#3885=VECTOR('',#13829,1000.);
#3886=VECTOR('',#13832,1000.);
#3887=VECTOR('',#13833,1000.);
#3888=VECTOR('',#13836,1000.);
#3889=VECTOR('',#13839,1000.);
#3890=VECTOR('',#13842,1000.);
#3891=VECTOR('',#13847,1000.);
#3892=VECTOR('',#13850,1000.);
#3893=VECTOR('',#13853,1000.);
#3894=VECTOR('',#13854,1000.);
#3895=VECTOR('',#13857,1000.);
#3896=VECTOR('',#13858,1000.);
#3897=VECTOR('',#13859,1000.);
#3898=VECTOR('',#13860,1000.);
#3899=VECTOR('',#13861,1000.);
#3900=VECTOR('',#13862,1000.);
#3901=VECTOR('',#13863,1000.);
#3902=VECTOR('',#13864,1000.);
#3903=VECTOR('',#13867,1000.);
#3904=VECTOR('',#13868,1000.);
#3905=VECTOR('',#13869,1000.);
#3906=VECTOR('',#13874,1000.);
#3907=VECTOR('',#13877,1000.);
#3908=VECTOR('',#13878,1000.);
#3909=VECTOR('',#13879,1000.);
#3910=VECTOR('',#13880,1000.);
#3911=VECTOR('',#13881,1000.);
#3912=VECTOR('',#13886,1000.);
#3913=VECTOR('',#13891,1000.);
#3914=VECTOR('',#13898,1000.);
#3915=VECTOR('',#13903,1000.);
#3916=VECTOR('',#13906,1000.);
#3917=VECTOR('',#13907,1000.);
#3918=VECTOR('',#13910,1000.);
#3919=VECTOR('',#13911,1000.);
#3920=VECTOR('',#13914,1000.);
#3921=VECTOR('',#13919,1000.);
#3922=VECTOR('',#13924,1000.);
#3923=VECTOR('',#13925,1000.);
#3924=VECTOR('',#13928,1000.);
#3925=VECTOR('',#13949,1000.);
#3926=VECTOR('',#13954,1000.);
#3927=VECTOR('',#13959,1000.);
#3928=VECTOR('',#13960,1000.);
#3929=VECTOR('',#13961,1000.);
#3930=VECTOR('',#13962,1000.);
#3931=VECTOR('',#13963,1000.);
#3932=VECTOR('',#13968,1000.);
#3933=VECTOR('',#13971,1000.);
#3934=VECTOR('',#13972,1000.);
#3935=VECTOR('',#13975,1000.);
#3936=VECTOR('',#13976,1000.);
#3937=VECTOR('',#13979,1000.);
#3938=VECTOR('',#13980,1000.);
#3939=VECTOR('',#13995,1000.);
#3940=VECTOR('',#13996,1000.);
#3941=VECTOR('',#13997,1000.);
#3942=VECTOR('',#14000,1000.);
#3943=VECTOR('',#14001,1000.);
#3944=VECTOR('',#14004,1000.);
#3945=VECTOR('',#14005,1000.);
#3946=VECTOR('',#14008,1000.);
#3947=VECTOR('',#14011,1000.);
#3948=VECTOR('',#14012,1000.);
#3949=VECTOR('',#14013,1000.);
#3950=VECTOR('',#14016,1000.);
#3951=VECTOR('',#14017,1000.);
#3952=VECTOR('',#14020,1000.);
#3953=VECTOR('',#14021,1000.);
#3954=VECTOR('',#14024,1000.);
#4314=CIRCLE('',#11217,5.5);
#4315=CIRCLE('',#11218,5.5);
#4316=CIRCLE('',#11220,14.);
#4317=CIRCLE('',#11221,14.);
#4318=CIRCLE('',#11223,1.35);
#4319=CIRCLE('',#11224,1.35);
#4320=CIRCLE('',#11226,1.35);
#4321=CIRCLE('',#11227,1.35);
#4322=CIRCLE('',#11229,1.35);
#4323=CIRCLE('',#11230,1.35);
#4324=CIRCLE('',#11232,1.35);
#4325=CIRCLE('',#11233,1.35);
#4326=CIRCLE('',#11235,1.35);
#4327=CIRCLE('',#11236,1.35);
#4328=CIRCLE('',#11238,1.35);
#4329=CIRCLE('',#11239,1.35);
#4330=CIRCLE('',#11241,1.35);
#4331=CIRCLE('',#11242,1.35);
#4332=CIRCLE('',#11244,1.35);
#4333=CIRCLE('',#11245,1.35);
#4334=CIRCLE('',#11247,1.35);
#4335=CIRCLE('',#11248,1.35);
#4336=CIRCLE('',#11250,1.35);
#4337=CIRCLE('',#11251,1.35);
#4338=CIRCLE('',#11253,1.35);
#4339=CIRCLE('',#11254,1.35);
#4340=CIRCLE('',#11256,1.35);
#4341=CIRCLE('',#11257,1.35);
#4342=CIRCLE('',#11259,5.);
#4343=CIRCLE('',#11260,5.);
#4344=CIRCLE('',#11262,7.5);
#4345=CIRCLE('',#11263,7.5);
#4346=CIRCLE('',#11265,2.75);
#4347=CIRCLE('',#11266,2.75);
#4348=CIRCLE('',#11268,5.);
#4349=CIRCLE('',#11269,5.);
#4350=CIRCLE('',#11271,7.25);
#4351=CIRCLE('',#11272,7.25);
#4352=CIRCLE('',#11274,14.);
#4353=CIRCLE('',#11275,14.);
#4354=CIRCLE('',#11277,4.75);
#4355=CIRCLE('',#11278,4.75);
#4356=CIRCLE('',#11280,2.75);
#4357=CIRCLE('',#11281,2.75);
#4358=CIRCLE('',#11284,2.);
#4359=CIRCLE('',#11285,2.);
#4360=CIRCLE('',#11287,1.5);
#4361=CIRCLE('',#11288,1.5);
#4362=CIRCLE('',#11290,1.5);
#4363=CIRCLE('',#11291,1.5);
#4364=CIRCLE('',#11293,1.5);
#4365=CIRCLE('',#11294,1.5);
#4366=CIRCLE('',#11297,0.49999972876243);
#4367=CIRCLE('',#11298,1.50000000000168);
#4368=CIRCLE('',#11299,0.499999999994099);
#4369=CIRCLE('',#11300,1.49999999999602);
#4370=CIRCLE('',#11307,2.);
#4371=CIRCLE('',#11308,2.);
#4372=CIRCLE('',#11310,2.);
#4373=CIRCLE('',#11311,2.);
#4374=CIRCLE('',#11313,2.);
#4375=CIRCLE('',#11314,2.);
#4376=CIRCLE('',#11316,3.);
#4377=CIRCLE('',#11317,3.);
#4378=CIRCLE('',#11318,3.);
#4379=CIRCLE('',#11319,3.);
#4380=CIRCLE('',#11320,3.);
#4381=CIRCLE('',#11321,1.5);
#4382=CIRCLE('',#11322,2.35);
#4383=CIRCLE('',#11323,0.999999999999999);
#4384=CIRCLE('',#11324,0.999999999999999);
#4385=CIRCLE('',#11325,2.35);
#4386=CIRCLE('',#11326,1.);
#4387=CIRCLE('',#11327,1.);
#4388=CIRCLE('',#11328,2.35);
#4389=CIRCLE('',#11329,0.999999999999999);
#4390=CIRCLE('',#11330,0.999999999999999);
#4391=CIRCLE('',#11331,2.35);
#4392=CIRCLE('',#11332,1.50000000000001);
#4393=CIRCLE('',#11333,2.);
#4394=CIRCLE('',#11334,3.);
#4395=CIRCLE('',#11336,3.5);
#4396=CIRCLE('',#11337,3.5);
#4397=CIRCLE('',#11339,2.);
#4398=CIRCLE('',#11341,2.);
#4399=CIRCLE('',#11342,2.);
#4400=CIRCLE('',#11344,2.);
#4401=CIRCLE('',#11345,2.);
#4402=CIRCLE('',#11347,1.5);
#4403=CIRCLE('',#11349,1.5);
#4404=CIRCLE('',#11351,3.);
#4405=CIRCLE('',#11352,3.);
#4406=CIRCLE('',#11353,0.999999999999999);
#4407=CIRCLE('',#11354,0.999999999999999);
#4408=CIRCLE('',#11355,3.);
#4409=CIRCLE('',#11356,3.);
#4410=CIRCLE('',#11357,3.);
#4411=CIRCLE('',#11358,3.);
#4412=CIRCLE('',#11360,0.999999999999996);
#4413=CIRCLE('',#11362,0.99999999999999);
#4414=CIRCLE('',#11370,3.);
#4415=CIRCLE('',#11373,3.);
#4416=CIRCLE('',#11376,3.);
#4417=CIRCLE('',#11377,3.);
#4418=CIRCLE('',#11378,3.);
#4419=CIRCLE('',#11381,3.);
#4420=CIRCLE('',#11382,3.);
#4421=CIRCLE('',#11383,3.);
#4422=CIRCLE('',#11386,3.);
#4423=CIRCLE('',#11389,3.);
#4424=CIRCLE('',#11391,1.5);
#4425=CIRCLE('',#11392,2.00000000000001);
#4426=CIRCLE('',#11395,2.35);
#4427=CIRCLE('',#11398,0.999999999999057);
#4428=CIRCLE('',#11401,1.00000000000512);
#4429=CIRCLE('',#11404,2.35);
#4430=CIRCLE('',#11407,0.999999999999075);
#4431=CIRCLE('',#11410,1.00000000000602);
#4432=CIRCLE('',#11413,2.35);
#4433=CIRCLE('',#11416,1.00000000000513);
#4434=CIRCLE('',#11419,1.00000000000602);
#4435=CIRCLE('',#11422,2.35);
#4436=CIRCLE('',#11424,2.00000000000002);
#4437=CIRCLE('',#11426,1.5);
#4438=CIRCLE('',#11429,3.85000089750977);
#4439=CIRCLE('',#11430,3.85000061127743);
#4440=CIRCLE('',#11431,3.84999875153457);
#4441=CIRCLE('',#11432,3.84999771098492);
#4442=CIRCLE('',#11439,3.);
#4443=CIRCLE('',#11442,3.);
#4444=CIRCLE('',#11443,3.);
#4445=CIRCLE('',#11444,3.);
#4446=CIRCLE('',#11447,3.);
#4447=CIRCLE('',#11448,3.);
#4448=CIRCLE('',#11449,3.);
#4449=CIRCLE('',#11452,3.);
#4450=CIRCLE('',#11455,3.);
#4451=CIRCLE('',#11457,3.);
#4452=CIRCLE('',#11463,2.);
#4453=CIRCLE('',#11465,2.);
#4454=CIRCLE('',#11522,1.5);
#4455=CIRCLE('',#11524,1.5);
#4456=CIRCLE('',#11526,1.5);
#4457=CIRCLE('',#11528,1.5);
#4458=CIRCLE('',#11529,1.5);
#4459=CIRCLE('',#11531,1.5);
#4460=CIRCLE('',#11532,1.5);
#4461=CIRCLE('',#11534,1.5);
#4462=CIRCLE('',#11536,1.5);
#4463=CIRCLE('',#11538,1.5);
#4464=CIRCLE('',#11539,1.5);
#4465=CIRCLE('',#11541,1.5);
#4466=CIRCLE('',#11542,1.5);
#4467=CIRCLE('',#11544,1.5);
#4468=CIRCLE('',#11546,1.5);
#4469=CIRCLE('',#11548,1.5);
#4470=CIRCLE('',#11549,1.5);
#4471=CIRCLE('',#11551,1.5);
#4472=CIRCLE('',#11552,1.5);
#4473=CIRCLE('',#11554,1.5);
#4474=CIRCLE('',#11583,2.);
#4475=CIRCLE('',#11585,2.);
#4809=VERTEX_POINT('',#15690);
#4810=VERTEX_POINT('',#15692);
#4811=VERTEX_POINT('',#15696);
#4812=VERTEX_POINT('',#15698);
#4813=VERTEX_POINT('',#15702);
#4814=VERTEX_POINT('',#15704);
#4815=VERTEX_POINT('',#15708);
#4816=VERTEX_POINT('',#15710);
#4817=VERTEX_POINT('',#15714);
#4818=VERTEX_POINT('',#15716);
#4819=VERTEX_POINT('',#15720);
#4820=VERTEX_POINT('',#15722);
#4821=VERTEX_POINT('',#15726);
#4822=VERTEX_POINT('',#15728);
#4823=VERTEX_POINT('',#15732);
#4824=VERTEX_POINT('',#15734);
#4825=VERTEX_POINT('',#15738);
#4826=VERTEX_POINT('',#15740);
#4827=VERTEX_POINT('',#15744);
#4828=VERTEX_POINT('',#15746);
#4829=VERTEX_POINT('',#15750);
#4830=VERTEX_POINT('',#15752);
#4831=VERTEX_POINT('',#15756);
#4832=VERTEX_POINT('',#15758);
#4833=VERTEX_POINT('',#15762);
#4834=VERTEX_POINT('',#15764);
#4835=VERTEX_POINT('',#15768);
#4836=VERTEX_POINT('',#15770);
#4837=VERTEX_POINT('',#15774);
#4838=VERTEX_POINT('',#15776);
#4839=VERTEX_POINT('',#15780);
#4840=VERTEX_POINT('',#15782);
#4841=VERTEX_POINT('',#15786);
#4842=VERTEX_POINT('',#15788);
#4843=VERTEX_POINT('',#15792);
#4844=VERTEX_POINT('',#15794);
#4845=VERTEX_POINT('',#15798);
#4846=VERTEX_POINT('',#15800);
#4847=VERTEX_POINT('',#15804);
#4848=VERTEX_POINT('',#15806);
#4849=VERTEX_POINT('',#15810);
#4850=VERTEX_POINT('',#15812);
#4851=VERTEX_POINT('',#15816);
#4852=VERTEX_POINT('',#15818);
#4853=VERTEX_POINT('',#15822);
#4854=VERTEX_POINT('',#15823);
#4855=VERTEX_POINT('',#15825);
#4856=VERTEX_POINT('',#15827);
#4857=VERTEX_POINT('',#15831);
#4858=VERTEX_POINT('',#15833);
#4859=VERTEX_POINT('',#15837);
#4860=VERTEX_POINT('',#15838);
#4861=VERTEX_POINT('',#15843);
#4862=VERTEX_POINT('',#15844);
#4863=VERTEX_POINT('',#15849);
#4864=VERTEX_POINT('',#15851);
#4865=VERTEX_POINT('',#15856);
#4866=VERTEX_POINT('',#15858);
#4867=VERTEX_POINT('',#15860);
#4868=VERTEX_POINT('',#15862);
#4869=VERTEX_POINT('',#15864);
#4870=VERTEX_POINT('',#15866);
#4871=VERTEX_POINT('',#15868);
#4872=VERTEX_POINT('',#15870);
#4873=VERTEX_POINT('',#15872);
#4874=VERTEX_POINT('',#15874);
#4875=VERTEX_POINT('',#15876);
#4876=VERTEX_POINT('',#15878);
#4877=VERTEX_POINT('',#15880);
#4878=VERTEX_POINT('',#15882);
#4879=VERTEX_POINT('',#15884);
#4880=VERTEX_POINT('',#15886);
#4881=VERTEX_POINT('',#15904);
#4882=VERTEX_POINT('',#15922);
#4883=VERTEX_POINT('',#15926);
#4884=VERTEX_POINT('',#15927);
#4885=VERTEX_POINT('',#15929);
#4886=VERTEX_POINT('',#16119);
#4887=VERTEX_POINT('',#16120);
#4888=VERTEX_POINT('',#16174);
#4889=VERTEX_POINT('',#16179);
#4890=VERTEX_POINT('',#16238);
#4891=VERTEX_POINT('',#16240);
#4892=VERTEX_POINT('',#16242);
#4893=VERTEX_POINT('',#16297);
#4894=VERTEX_POINT('',#16298);
#4895=VERTEX_POINT('',#16303);
#4896=VERTEX_POINT('',#16304);
#4897=VERTEX_POINT('',#16309);
#4898=VERTEX_POINT('',#16310);
#4899=VERTEX_POINT('',#16315);
#4900=VERTEX_POINT('',#16316);
#4901=VERTEX_POINT('',#16318);
#4902=VERTEX_POINT('',#16320);
#4903=VERTEX_POINT('',#16322);
#4904=VERTEX_POINT('',#16324);
#4905=VERTEX_POINT('',#16326);
#4906=VERTEX_POINT('',#16328);
#4907=VERTEX_POINT('',#16330);
#4908=VERTEX_POINT('',#16332);
#4909=VERTEX_POINT('',#16334);
#4910=VERTEX_POINT('',#16337);
#4911=VERTEX_POINT('',#16339);
#4912=VERTEX_POINT('',#16341);
#4913=VERTEX_POINT('',#16343);
#4914=VERTEX_POINT('',#16345);
#4915=VERTEX_POINT('',#16347);
#4916=VERTEX_POINT('',#16349);
#4917=VERTEX_POINT('',#16351);
#4918=VERTEX_POINT('',#16353);
#4919=VERTEX_POINT('',#16355);
#4920=VERTEX_POINT('',#16357);
#4921=VERTEX_POINT('',#16359);
#4922=VERTEX_POINT('',#16361);
#4923=VERTEX_POINT('',#16363);
#4924=VERTEX_POINT('',#16365);
#4925=VERTEX_POINT('',#16367);
#4926=VERTEX_POINT('',#16369);
#4927=VERTEX_POINT('',#16371);
#4928=VERTEX_POINT('',#16373);
#4929=VERTEX_POINT('',#16375);
#4930=VERTEX_POINT('',#16377);
#4931=VERTEX_POINT('',#16379);
#4932=VERTEX_POINT('',#16382);
#4933=VERTEX_POINT('',#16384);
#4934=VERTEX_POINT('',#16388);
#4935=VERTEX_POINT('',#16390);
#4936=VERTEX_POINT('',#16394);
#4937=VERTEX_POINT('',#16398);
#4938=VERTEX_POINT('',#16400);
#4939=VERTEX_POINT('',#16404);
#4940=VERTEX_POINT('',#16406);
#4941=VERTEX_POINT('',#16414);
#4942=VERTEX_POINT('',#16415);
#4943=VERTEX_POINT('',#16417);
#4944=VERTEX_POINT('',#16419);
#4945=VERTEX_POINT('',#16424);
#4946=VERTEX_POINT('',#16426);
#4947=VERTEX_POINT('',#16428);
#4948=VERTEX_POINT('',#16430);
#4949=VERTEX_POINT('',#16432);
#4950=VERTEX_POINT('',#16434);
#4951=VERTEX_POINT('',#16436);
#4952=VERTEX_POINT('',#16438);
#4953=VERTEX_POINT('',#16535);
#4954=VERTEX_POINT('',#16536);
#4955=VERTEX_POINT('',#16538);
#4956=VERTEX_POINT('',#16541);
#4957=VERTEX_POINT('',#16543);
#4958=VERTEX_POINT('',#16547);
#4959=VERTEX_POINT('',#16551);
#4960=VERTEX_POINT('',#16552);
#4961=VERTEX_POINT('',#16554);
#4962=VERTEX_POINT('',#16556);
#4963=VERTEX_POINT('',#16558);
#4964=VERTEX_POINT('',#16560);
#4965=VERTEX_POINT('',#16562);
#4966=VERTEX_POINT('',#16564);
#4967=VERTEX_POINT('',#16566);
#4968=VERTEX_POINT('',#16568);
#4969=VERTEX_POINT('',#16570);
#4970=VERTEX_POINT('',#16572);
#4971=VERTEX_POINT('',#16574);
#4972=VERTEX_POINT('',#16576);
#4973=VERTEX_POINT('',#16578);
#4974=VERTEX_POINT('',#16581);
#4975=VERTEX_POINT('',#16583);
#4976=VERTEX_POINT('',#16585);
#4977=VERTEX_POINT('',#16587);
#4978=VERTEX_POINT('',#16589);
#4979=VERTEX_POINT('',#16591);
#4980=VERTEX_POINT('',#16593);
#4981=VERTEX_POINT('',#16595);
#4982=VERTEX_POINT('',#16597);
#4983=VERTEX_POINT('',#16599);
#4984=VERTEX_POINT('',#16601);
#4985=VERTEX_POINT('',#16603);
#4986=VERTEX_POINT('',#16605);
#4987=VERTEX_POINT('',#16607);
#4988=VERTEX_POINT('',#16609);
#4989=VERTEX_POINT('',#16611);
#4990=VERTEX_POINT('',#16613);
#4991=VERTEX_POINT('',#16615);
#4992=VERTEX_POINT('',#16617);
#4993=VERTEX_POINT('',#16619);
#4994=VERTEX_POINT('',#16621);
#4995=VERTEX_POINT('',#16623);
#4996=VERTEX_POINT('',#16627);
#4997=VERTEX_POINT('',#16631);
#4998=VERTEX_POINT('',#16632);
#4999=VERTEX_POINT('',#16634);
#5000=VERTEX_POINT('',#16636);
#5001=VERTEX_POINT('',#16641);
#5002=VERTEX_POINT('',#16643);
#5003=VERTEX_POINT('',#16647);
#5004=VERTEX_POINT('',#16649);
#5005=VERTEX_POINT('',#16651);
#5006=VERTEX_POINT('',#16653);
#5007=VERTEX_POINT('',#16655);
#5008=VERTEX_POINT('',#16657);
#5009=VERTEX_POINT('',#16659);
#5010=VERTEX_POINT('',#16661);
#5011=VERTEX_POINT('',#16663);
#5012=VERTEX_POINT('',#16665);
#5013=VERTEX_POINT('',#16667);
#5014=VERTEX_POINT('',#16669);
#5015=VERTEX_POINT('',#16671);
#5016=VERTEX_POINT('',#16675);
#5017=VERTEX_POINT('',#16679);
#5018=VERTEX_POINT('',#16683);
#5019=VERTEX_POINT('',#16684);
#5020=VERTEX_POINT('',#16686);
#5021=VERTEX_POINT('',#16691);
#5022=VERTEX_POINT('',#16693);
#5023=VERTEX_POINT('',#16695);
#5024=VERTEX_POINT('',#16697);
#5025=VERTEX_POINT('',#16699);
#5026=VERTEX_POINT('',#16701);
#5027=VERTEX_POINT('',#16703);
#5028=VERTEX_POINT('',#16705);
#5029=VERTEX_POINT('',#16707);
#5030=VERTEX_POINT('',#16711);
#5031=VERTEX_POINT('',#16713);
#5032=VERTEX_POINT('',#16718);
#5033=VERTEX_POINT('',#16722);
#5034=VERTEX_POINT('',#16726);
#5035=VERTEX_POINT('',#16728);
#5036=VERTEX_POINT('',#16730);
#5037=VERTEX_POINT('',#16732);
#5038=VERTEX_POINT('',#16734);
#5039=VERTEX_POINT('',#16736);
#5040=VERTEX_POINT('',#16738);
#5041=VERTEX_POINT('',#16740);
#5042=VERTEX_POINT('',#16742);
#5043=VERTEX_POINT('',#16744);
#5044=VERTEX_POINT('',#16746);
#5045=VERTEX_POINT('',#16748);
#5046=VERTEX_POINT('',#16750);
#5047=VERTEX_POINT('',#16756);
#5048=VERTEX_POINT('',#16760);
#5049=VERTEX_POINT('',#16764);
#5050=VERTEX_POINT('',#16768);
#5051=VERTEX_POINT('',#16769);
#5052=VERTEX_POINT('',#16777);
#5053=VERTEX_POINT('',#16781);
#5054=VERTEX_POINT('',#16786);
#5055=VERTEX_POINT('',#16788);
#5056=VERTEX_POINT('',#16795);
#5057=VERTEX_POINT('',#16799);
#5058=VERTEX_POINT('',#16801);
#5059=VERTEX_POINT('',#16808);
#5060=VERTEX_POINT('',#16812);
#5061=VERTEX_POINT('',#16813);
#5062=VERTEX_POINT('',#16821);
#5063=VERTEX_POINT('',#16825);
#5064=VERTEX_POINT('',#16830);
#5065=VERTEX_POINT('',#16832);
#5066=VERTEX_POINT('',#16839);
#5067=VERTEX_POINT('',#16843);
#5068=VERTEX_POINT('',#16845);
#5069=VERTEX_POINT('',#16852);
#5070=VERTEX_POINT('',#16856);
#5071=VERTEX_POINT('',#16857);
#5072=VERTEX_POINT('',#16865);
#5073=VERTEX_POINT('',#16869);
#5074=VERTEX_POINT('',#16874);
#5075=VERTEX_POINT('',#16876);
#5076=VERTEX_POINT('',#16883);
#5077=VERTEX_POINT('',#16887);
#5078=VERTEX_POINT('',#16889);
#5079=VERTEX_POINT('',#16896);
#5080=VERTEX_POINT('',#16900);
#5081=VERTEX_POINT('',#16906);
#5082=VERTEX_POINT('',#16908);
#5083=VERTEX_POINT('',#16910);
#5084=VERTEX_POINT('',#16912);
#5085=VERTEX_POINT('',#16916);
#5086=VERTEX_POINT('',#16917);
#5087=VERTEX_POINT('',#16919);
#5088=VERTEX_POINT('',#16921);
#5089=VERTEX_POINT('',#16923);
#5090=VERTEX_POINT('',#16925);
#5091=VERTEX_POINT('',#16927);
#5092=VERTEX_POINT('',#16929);
#5093=VERTEX_POINT('',#16931);
#5094=VERTEX_POINT('',#16933);
#5095=VERTEX_POINT('',#16935);
#5096=VERTEX_POINT('',#16937);
#5097=VERTEX_POINT('',#16939);
#5098=VERTEX_POINT('',#16941);
#5099=VERTEX_POINT('',#16946);
#5100=VERTEX_POINT('',#16950);
#5101=VERTEX_POINT('',#16952);
#5102=VERTEX_POINT('',#16956);
#5103=VERTEX_POINT('',#16957);
#5104=VERTEX_POINT('',#16959);
#5105=VERTEX_POINT('',#16961);
#5106=VERTEX_POINT('',#16963);
#5107=VERTEX_POINT('',#16965);
#5108=VERTEX_POINT('',#16967);
#5109=VERTEX_POINT('',#16969);
#5110=VERTEX_POINT('',#16971);
#5111=VERTEX_POINT('',#16974);
#5112=VERTEX_POINT('',#16976);
#5113=VERTEX_POINT('',#16978);
#5114=VERTEX_POINT('',#16980);
#5115=VERTEX_POINT('',#16982);
#5116=VERTEX_POINT('',#16984);
#5117=VERTEX_POINT('',#16986);
#5118=VERTEX_POINT('',#16988);
#5119=VERTEX_POINT('',#16990);
#5120=VERTEX_POINT('',#16992);
#5121=VERTEX_POINT('',#16994);
#5122=VERTEX_POINT('',#16996);
#5123=VERTEX_POINT('',#16998);
#5124=VERTEX_POINT('',#17000);
#5125=VERTEX_POINT('',#17002);
#5126=VERTEX_POINT('',#17004);
#5127=VERTEX_POINT('',#17006);
#5128=VERTEX_POINT('',#17009);
#5129=VERTEX_POINT('',#17011);
#5130=VERTEX_POINT('',#17013);
#5131=VERTEX_POINT('',#17015);
#5132=VERTEX_POINT('',#17017);
#5133=VERTEX_POINT('',#17019);
#5134=VERTEX_POINT('',#17021);
#5135=VERTEX_POINT('',#17023);
#5136=VERTEX_POINT('',#17025);
#5137=VERTEX_POINT('',#17029);
#5138=VERTEX_POINT('',#17031);
#5139=VERTEX_POINT('',#17033);
#5140=VERTEX_POINT('',#17035);
#5141=VERTEX_POINT('',#17039);
#5142=VERTEX_POINT('',#17040);
#5143=VERTEX_POINT('',#17042);
#5144=VERTEX_POINT('',#17045);
#5145=VERTEX_POINT('',#17047);
#5146=VERTEX_POINT('',#17049);
#5147=VERTEX_POINT('',#17051);
#5148=VERTEX_POINT('',#17053);
#5149=VERTEX_POINT('',#17055);
#5150=VERTEX_POINT('',#17057);
#5151=VERTEX_POINT('',#17059);
#5152=VERTEX_POINT('',#17061);
#5153=VERTEX_POINT('',#17063);
#5154=VERTEX_POINT('',#17065);
#5155=VERTEX_POINT('',#17069);
#5156=VERTEX_POINT('',#17073);
#5157=VERTEX_POINT('',#17077);
#5158=VERTEX_POINT('',#17079);
#5159=VERTEX_POINT('',#17084);
#5160=VERTEX_POINT('',#17085);
#5161=VERTEX_POINT('',#17088);
#5162=VERTEX_POINT('',#17090);
#5163=VERTEX_POINT('',#17092);
#5164=VERTEX_POINT('',#17094);
#5165=VERTEX_POINT('',#17096);
#5166=VERTEX_POINT('',#17098);
#5167=VERTEX_POINT('',#17100);
#5168=VERTEX_POINT('',#17104);
#5169=VERTEX_POINT('',#17107);
#5170=VERTEX_POINT('',#17111);
#5171=VERTEX_POINT('',#17115);
#5172=VERTEX_POINT('',#17119);
#5173=VERTEX_POINT('',#17120);
#5174=VERTEX_POINT('',#17123);
#5175=VERTEX_POINT('',#17125);
#5176=VERTEX_POINT('',#17127);
#5177=VERTEX_POINT('',#17129);
#5178=VERTEX_POINT('',#17131);
#5179=VERTEX_POINT('',#17133);
#5180=VERTEX_POINT('',#17135);
#5181=VERTEX_POINT('',#17137);
#5182=VERTEX_POINT('',#17139);
#5183=VERTEX_POINT('',#17141);
#5184=VERTEX_POINT('',#17143);
#5185=VERTEX_POINT('',#17151);
#5186=VERTEX_POINT('',#17153);
#5187=VERTEX_POINT('',#17161);
#5188=VERTEX_POINT('',#17166);
#5189=VERTEX_POINT('',#17167);
#5190=VERTEX_POINT('',#17170);
#5191=VERTEX_POINT('',#17174);
#5192=VERTEX_POINT('',#17178);
#5193=VERTEX_POINT('',#17180);
#5194=VERTEX_POINT('',#17182);
#5195=VERTEX_POINT('',#17190);
#5196=VERTEX_POINT('',#17192);
#5197=VERTEX_POINT('',#17196);
#5198=VERTEX_POINT('',#17200);
#5199=VERTEX_POINT('',#17202);
#5200=VERTEX_POINT('',#17206);
#5201=VERTEX_POINT('',#17210);
#5202=VERTEX_POINT('',#17214);
#5203=VERTEX_POINT('',#17215);
#5204=VERTEX_POINT('',#17220);
#5205=VERTEX_POINT('',#17223);
#5206=VERTEX_POINT('',#17227);
#5207=VERTEX_POINT('',#17232);
#5208=VERTEX_POINT('',#17242);
#5209=VERTEX_POINT('',#17246);
#5210=VERTEX_POINT('',#17251);
#5211=VERTEX_POINT('',#17256);
#5212=VERTEX_POINT('',#17261);
#5213=VERTEX_POINT('',#17271);
#5214=VERTEX_POINT('',#17275);
#5215=VERTEX_POINT('',#17280);
#5216=VERTEX_POINT('',#17288);
#5217=VERTEX_POINT('',#17292);
#5218=VERTEX_POINT('',#17294);
#5219=VERTEX_POINT('',#17296);
#5220=VERTEX_POINT('',#17300);
#5221=VERTEX_POINT('',#17302);
#5222=VERTEX_POINT('',#17304);
#5223=VERTEX_POINT('',#17308);
#5224=VERTEX_POINT('',#17310);
#5225=VERTEX_POINT('',#17312);
#5226=VERTEX_POINT('',#17316);
#5227=VERTEX_POINT('',#17318);
#5228=VERTEX_POINT('',#17320);
#5229=VERTEX_POINT('',#17324);
#5230=VERTEX_POINT('',#17326);
#5231=VERTEX_POINT('',#17328);
#5232=VERTEX_POINT('',#17332);
#5233=VERTEX_POINT('',#17334);
#5234=VERTEX_POINT('',#17338);
#5235=VERTEX_POINT('',#17349);
#5236=VERTEX_POINT('',#17353);
#5237=VERTEX_POINT('',#17357);
#5238=VERTEX_POINT('',#17359);
#5239=VERTEX_POINT('',#17363);
#5240=VERTEX_POINT('',#17369);
#5241=VERTEX_POINT('',#17373);
#5242=VERTEX_POINT('',#17375);
#5243=VERTEX_POINT('',#17379);
#5244=VERTEX_POINT('',#17383);
#5245=VERTEX_POINT('',#17387);
#5246=VERTEX_POINT('',#17436);
#5247=VERTEX_POINT('',#17448);
#5248=VERTEX_POINT('',#17452);
#5249=VERTEX_POINT('',#17457);
#5250=VERTEX_POINT('',#17467);
#5251=VERTEX_POINT('',#17471);
#5252=VERTEX_POINT('',#17475);
#5253=VERTEX_POINT('',#17479);
#5254=VERTEX_POINT('',#17487);
#5255=VERTEX_POINT('',#17492);
#5256=VERTEX_POINT('',#17496);
#5257=VERTEX_POINT('',#17500);
#5258=VERTEX_POINT('',#17502);
#5259=VERTEX_POINT('',#17506);
#5260=VERTEX_POINT('',#17510);
#5261=VERTEX_POINT('',#17514);
#5262=VERTEX_POINT('',#17518);
#5263=VERTEX_POINT('',#17522);
#5264=VERTEX_POINT('',#17524);
#5265=VERTEX_POINT('',#17526);
#5266=VERTEX_POINT('',#17530);
#5267=VERTEX_POINT('',#17534);
#5268=VERTEX_POINT('',#17536);
#5269=VERTEX_POINT('',#17538);
#5270=VERTEX_POINT('',#17546);
#5271=VERTEX_POINT('',#17550);
#5272=VERTEX_POINT('',#17552);
#5273=VERTEX_POINT('',#17554);
#5274=VERTEX_POINT('',#17558);
#5275=VERTEX_POINT('',#17559);
#5276=VERTEX_POINT('',#17562);
#5277=VERTEX_POINT('',#17566);
#5278=VERTEX_POINT('',#17568);
#5279=VERTEX_POINT('',#17572);
#5280=VERTEX_POINT('',#17574);
#5281=VERTEX_POINT('',#17576);
#5282=VERTEX_POINT('',#17580);
#5283=VERTEX_POINT('',#17581);
#5284=VERTEX_POINT('',#17584);
#5285=VERTEX_POINT('',#17588);
#5286=VERTEX_POINT('',#17590);
#5287=VERTEX_POINT('',#17600);
#5288=VERTEX_POINT('',#17604);
#5289=VERTEX_POINT('',#17606);
#5290=VERTEX_POINT('',#17610);
#5291=VERTEX_POINT('',#17614);
#5292=VERTEX_POINT('',#17618);
#5293=VERTEX_POINT('',#17633);
#5294=VERTEX_POINT('',#17637);
#5295=VERTEX_POINT('',#17639);
#5296=VERTEX_POINT('',#17642);
#5297=VERTEX_POINT('',#17645);
#5298=VERTEX_POINT('',#17650);
#5299=VERTEX_POINT('',#17659);
#5300=VERTEX_POINT('',#17660);
#5301=VERTEX_POINT('',#17662);
#5302=VERTEX_POINT('',#17664);
#5303=VERTEX_POINT('',#17681);
#5304=VERTEX_POINT('',#18420);
#5305=VERTEX_POINT('',#18421);
#5306=VERTEX_POINT('',#18423);
#5307=VERTEX_POINT('',#18425);
#5308=VERTEX_POINT('',#18432);
#5309=VERTEX_POINT('',#18448);
#5310=VERTEX_POINT('',#18449);
#5311=VERTEX_POINT('',#18454);
#5312=VERTEX_POINT('',#18458);
#5313=VERTEX_POINT('',#18728);
#5314=VERTEX_POINT('',#18729);
#5315=VERTEX_POINT('',#18734);
#5316=VERTEX_POINT('',#18738);
#5825=EDGE_CURVE('',#4809,#4809,#4314,.T.);
#5826=EDGE_CURVE('',#4809,#4810,#2353,.T.);
#5827=EDGE_CURVE('',#4810,#4810,#4315,.T.);
#5828=EDGE_CURVE('',#4811,#4811,#4316,.T.);
#5829=EDGE_CURVE('',#4811,#4812,#2354,.T.);
#5830=EDGE_CURVE('',#4812,#4812,#4317,.T.);
#5831=EDGE_CURVE('',#4813,#4813,#4318,.T.);
#5832=EDGE_CURVE('',#4813,#4814,#2355,.T.);
#5833=EDGE_CURVE('',#4814,#4814,#4319,.T.);
#5834=EDGE_CURVE('',#4815,#4815,#4320,.T.);
#5835=EDGE_CURVE('',#4815,#4816,#2356,.T.);
#5836=EDGE_CURVE('',#4816,#4816,#4321,.T.);
#5837=EDGE_CURVE('',#4817,#4817,#4322,.T.);
#5838=EDGE_CURVE('',#4817,#4818,#2357,.T.);
#5839=EDGE_CURVE('',#4818,#4818,#4323,.T.);
#5840=EDGE_CURVE('',#4819,#4819,#4324,.T.);
#5841=EDGE_CURVE('',#4819,#4820,#2358,.T.);
#5842=EDGE_CURVE('',#4820,#4820,#4325,.T.);
#5843=EDGE_CURVE('',#4821,#4821,#4326,.T.);
#5844=EDGE_CURVE('',#4821,#4822,#2359,.T.);
#5845=EDGE_CURVE('',#4822,#4822,#4327,.T.);
#5846=EDGE_CURVE('',#4823,#4823,#4328,.T.);
#5847=EDGE_CURVE('',#4823,#4824,#2360,.T.);
#5848=EDGE_CURVE('',#4824,#4824,#4329,.T.);
#5849=EDGE_CURVE('',#4825,#4825,#4330,.T.);
#5850=EDGE_CURVE('',#4825,#4826,#2361,.T.);
#5851=EDGE_CURVE('',#4826,#4826,#4331,.T.);
#5852=EDGE_CURVE('',#4827,#4827,#4332,.T.);
#5853=EDGE_CURVE('',#4827,#4828,#2362,.T.);
#5854=EDGE_CURVE('',#4828,#4828,#4333,.T.);
#5855=EDGE_CURVE('',#4829,#4829,#4334,.T.);
#5856=EDGE_CURVE('',#4829,#4830,#2363,.T.);
#5857=EDGE_CURVE('',#4830,#4830,#4335,.T.);
#5858=EDGE_CURVE('',#4831,#4831,#4336,.T.);
#5859=EDGE_CURVE('',#4831,#4832,#2364,.T.);
#5860=EDGE_CURVE('',#4832,#4832,#4337,.T.);
#5861=EDGE_CURVE('',#4833,#4833,#4338,.T.);
#5862=EDGE_CURVE('',#4833,#4834,#2365,.T.);
#5863=EDGE_CURVE('',#4834,#4834,#4339,.T.);
#5864=EDGE_CURVE('',#4835,#4835,#4340,.T.);
#5865=EDGE_CURVE('',#4835,#4836,#2366,.T.);
#5866=EDGE_CURVE('',#4836,#4836,#4341,.T.);
#5867=EDGE_CURVE('',#4837,#4837,#4342,.T.);
#5868=EDGE_CURVE('',#4837,#4838,#2367,.T.);
#5869=EDGE_CURVE('',#4838,#4838,#4343,.T.);
#5870=EDGE_CURVE('',#4839,#4839,#4344,.T.);
#5871=EDGE_CURVE('',#4839,#4840,#2368,.T.);
#5872=EDGE_CURVE('',#4840,#4840,#4345,.T.);
#5873=EDGE_CURVE('',#4841,#4841,#4346,.T.);
#5874=EDGE_CURVE('',#4841,#4842,#2369,.T.);
#5875=EDGE_CURVE('',#4842,#4842,#4347,.T.);
#5876=EDGE_CURVE('',#4843,#4843,#4348,.T.);
#5877=EDGE_CURVE('',#4843,#4844,#2370,.T.);
#5878=EDGE_CURVE('',#4844,#4844,#4349,.T.);
#5879=EDGE_CURVE('',#4845,#4845,#4350,.T.);
#5880=EDGE_CURVE('',#4845,#4846,#2371,.T.);
#5881=EDGE_CURVE('',#4846,#4846,#4351,.T.);
#5882=EDGE_CURVE('',#4847,#4847,#4352,.T.);
#5883=EDGE_CURVE('',#4847,#4848,#2372,.T.);
#5884=EDGE_CURVE('',#4848,#4848,#4353,.T.);
#5885=EDGE_CURVE('',#4849,#4849,#4354,.T.);
#5886=EDGE_CURVE('',#4849,#4850,#2373,.T.);
#5887=EDGE_CURVE('',#4850,#4850,#4355,.T.);
#5888=EDGE_CURVE('',#4851,#4851,#4356,.T.);
#5889=EDGE_CURVE('',#4851,#4852,#2374,.T.);
#5890=EDGE_CURVE('',#4852,#4852,#4357,.T.);
#5891=EDGE_CURVE('',#4853,#4854,#2375,.T.);
#5892=EDGE_CURVE('',#4854,#4855,#2376,.T.);
#5893=EDGE_CURVE('',#4855,#4856,#2377,.T.);
#5894=EDGE_CURVE('',#4856,#4853,#2378,.T.);
#5895=EDGE_CURVE('',#4854,#4857,#4358,.T.);
#5896=EDGE_CURVE('',#4857,#4858,#2379,.T.);
#5897=EDGE_CURVE('',#4858,#4855,#4359,.T.);
#5898=EDGE_CURVE('',#4859,#4860,#2380,.T.);
#5899=EDGE_CURVE('',#4860,#4854,#4360,.T.);
#5900=EDGE_CURVE('',#4853,#4859,#4361,.T.);
#5901=EDGE_CURVE('',#4861,#4862,#2381,.T.);
#5902=EDGE_CURVE('',#4862,#4853,#4362,.T.);
#5903=EDGE_CURVE('',#4856,#4861,#4363,.T.);
#5904=EDGE_CURVE('',#4855,#4863,#4364,.T.);
#5905=EDGE_CURVE('',#4863,#4864,#2382,.T.);
#5906=EDGE_CURVE('',#4864,#4856,#4365,.T.);
#5907=EDGE_CURVE('',#4865,#4857,#2383,.T.);
#5908=EDGE_CURVE('',#4866,#4865,#2384,.T.);
#5909=EDGE_CURVE('',#4866,#4867,#2385,.T.);
#5910=EDGE_CURVE('',#4867,#4868,#2386,.T.);
#5911=EDGE_CURVE('',#4868,#4869,#2387,.T.);
#5912=EDGE_CURVE('',#4870,#4869,#2388,.T.);
#5913=EDGE_CURVE('',#4870,#4871,#2389,.T.);
#5914=EDGE_CURVE('',#4871,#4872,#2390,.T.);
#5915=EDGE_CURVE('',#4872,#4873,#2391,.T.);
#5916=EDGE_CURVE('',#4873,#4874,#2392,.T.);
#5917=EDGE_CURVE('',#4874,#4875,#2393,.T.);
#5918=EDGE_CURVE('',#4876,#4875,#2394,.T.);
#5919=EDGE_CURVE('',#4876,#4877,#2395,.T.);
#5920=EDGE_CURVE('',#4877,#4878,#2396,.T.);
#5921=EDGE_CURVE('',#4878,#4879,#2397,.T.);
#5922=EDGE_CURVE('',#4880,#4879,#2398,.T.);
#5923=EDGE_CURVE('',#4858,#4880,#2399,.T.);
#5924=EDGE_CURVE('',#4860,#4881,#4366,.T.);
#5925=EDGE_CURVE('',#4881,#4857,#4367,.T.);
#5926=EDGE_CURVE('',#4882,#4863,#4368,.T.);
#5927=EDGE_CURVE('',#4858,#4882,#4369,.T.);
#5928=EDGE_CURVE('',#4883,#4884,#2400,.T.);
#5929=EDGE_CURVE('',#4884,#4885,#2401,.T.);
#5930=EDGE_CURVE('',#4885,#4881,#2402,.T.);
#5931=EDGE_CURVE('',#4883,#4859,#264,.T.);
#5932=EDGE_CURVE('',#4862,#4859,#265,.T.);
#5933=EDGE_CURVE('',#4886,#4887,#2403,.T.);
#5934=EDGE_CURVE('',#4887,#4862,#266,.T.);
#5935=EDGE_CURVE('',#4888,#4861,#267,.T.);
#5936=EDGE_CURVE('',#4888,#4889,#2404,.T.);
#5937=EDGE_CURVE('',#4889,#4886,#2405,.T.);
#5938=EDGE_CURVE('',#4864,#4861,#268,.T.);
#5939=EDGE_CURVE('',#4882,#4890,#2406,.T.);
#5940=EDGE_CURVE('',#4890,#4891,#2407,.T.);
#5941=EDGE_CURVE('',#4891,#4892,#2408,.T.);
#5942=EDGE_CURVE('',#4892,#4864,#269,.T.);
#5943=EDGE_CURVE('',#4893,#4894,#2409,.T.);
#5944=EDGE_CURVE('',#4894,#4879,#4370,.T.);
#5945=EDGE_CURVE('',#4878,#4893,#4371,.T.);
#5946=EDGE_CURVE('',#4895,#4896,#2410,.T.);
#5947=EDGE_CURVE('',#4896,#4877,#4372,.T.);
#5948=EDGE_CURVE('',#4876,#4895,#4373,.T.);
#5949=EDGE_CURVE('',#4897,#4898,#2411,.T.);
#5950=EDGE_CURVE('',#4898,#4875,#4374,.T.);
#5951=EDGE_CURVE('',#4874,#4897,#4375,.T.);
#5952=EDGE_CURVE('',#4899,#4900,#2412,.T.);
#5953=EDGE_CURVE('',#4901,#4899,#4376,.T.);
#5954=EDGE_CURVE('',#4902,#4901,#2413,.T.);
#5955=EDGE_CURVE('',#4903,#4902,#4377,.T.);
#5956=EDGE_CURVE('',#4904,#4903,#2414,.T.);
#5957=EDGE_CURVE('',#4905,#4904,#4378,.T.);
#5958=EDGE_CURVE('',#4906,#4905,#2415,.T.);
#5959=EDGE_CURVE('',#4907,#4906,#4379,.T.);
#5960=EDGE_CURVE('',#4908,#4907,#2416,.T.);
#5961=EDGE_CURVE('',#4909,#4908,#4380,.T.);
#5962=EDGE_CURVE('',#4897,#4909,#2417,.T.);
#5963=EDGE_CURVE('',#4910,#4873,#4381,.T.);
#5964=EDGE_CURVE('',#4911,#4910,#2418,.T.);
#5965=EDGE_CURVE('',#4912,#4911,#4382,.T.);
#5966=EDGE_CURVE('',#4913,#4912,#2419,.T.);
#5967=EDGE_CURVE('',#4914,#4913,#4383,.T.);
#5968=EDGE_CURVE('',#4915,#4914,#2420,.T.);
#5969=EDGE_CURVE('',#4916,#4915,#4384,.T.);
#5970=EDGE_CURVE('',#4917,#4916,#2421,.T.);
#5971=EDGE_CURVE('',#4918,#4917,#4385,.T.);
#5972=EDGE_CURVE('',#4919,#4918,#2422,.T.);
#5973=EDGE_CURVE('',#4920,#4919,#4386,.T.);
#5974=EDGE_CURVE('',#4921,#4920,#2423,.T.);
#5975=EDGE_CURVE('',#4922,#4921,#4387,.T.);
#5976=EDGE_CURVE('',#4923,#4922,#2424,.T.);
#5977=EDGE_CURVE('',#4924,#4923,#4388,.T.);
#5978=EDGE_CURVE('',#4925,#4924,#2425,.T.);
#5979=EDGE_CURVE('',#4926,#4925,#4389,.T.);
#5980=EDGE_CURVE('',#4927,#4926,#2426,.T.);
#5981=EDGE_CURVE('',#4928,#4927,#4390,.T.);
#5982=EDGE_CURVE('',#4929,#4928,#2427,.T.);
#5983=EDGE_CURVE('',#4930,#4929,#4391,.T.);
#5984=EDGE_CURVE('',#4931,#4930,#2428,.T.);
#5985=EDGE_CURVE('',#4872,#4931,#4392,.T.);
#5986=EDGE_CURVE('',#4932,#4871,#4393,.T.);
#5987=EDGE_CURVE('',#4933,#4932,#2429,.T.);
#5988=EDGE_CURVE('',#4900,#4933,#4394,.T.);
#5989=EDGE_CURVE('',#4934,#4873,#4395,.T.);
#5990=EDGE_CURVE('',#4872,#4935,#4396,.T.);
#5991=EDGE_CURVE('',#4935,#4934,#2430,.T.);
#5992=EDGE_CURVE('',#4870,#4936,#4397,.T.);
#5993=EDGE_CURVE('',#4936,#4932,#2431,.T.);
#5994=EDGE_CURVE('',#4868,#4937,#4398,.T.);
#5995=EDGE_CURVE('',#4937,#4938,#2432,.T.);
#5996=EDGE_CURVE('',#4938,#4869,#4399,.T.);
#5997=EDGE_CURVE('',#4866,#4939,#4400,.T.);
#5998=EDGE_CURVE('',#4939,#4940,#2433,.T.);
#5999=EDGE_CURVE('',#4940,#4867,#4401,.T.);
#6000=EDGE_CURVE('',#4885,#4865,#4402,.T.);
#6001=EDGE_CURVE('',#4880,#4890,#4403,.T.);
#6002=EDGE_CURVE('',#4941,#4942,#4404,.T.);
#6003=EDGE_CURVE('',#4942,#4943,#2434,.T.);
#6004=EDGE_CURVE('',#4943,#4944,#4405,.T.);
#6005=EDGE_CURVE('',#4944,#4939,#2435,.T.);
#6006=EDGE_CURVE('',#4884,#4886,#4406,.T.);
#6007=EDGE_CURVE('',#4889,#4891,#4407,.T.);
#6008=EDGE_CURVE('',#4894,#4945,#2436,.T.);
#6009=EDGE_CURVE('',#4945,#4946,#4408,.T.);
#6010=EDGE_CURVE('',#4946,#4947,#2437,.T.);
#6011=EDGE_CURVE('',#4947,#4948,#4409,.T.);
#6012=EDGE_CURVE('',#4948,#4949,#2438,.T.);
#6013=EDGE_CURVE('',#4949,#4950,#4410,.T.);
#6014=EDGE_CURVE('',#4950,#4951,#2439,.T.);
#6015=EDGE_CURVE('',#4951,#4952,#4411,.T.);
#6016=EDGE_CURVE('',#4952,#4941,#2440,.T.);
#6017=EDGE_CURVE('',#4883,#4887,#4412,.T.);
#6018=EDGE_CURVE('',#4888,#4892,#4413,.T.);
#6019=EDGE_CURVE('',#4953,#4954,#2441,.T.);
#6020=EDGE_CURVE('',#4955,#4954,#2442,.T.);
#6021=EDGE_CURVE('',#4955,#4945,#2443,.T.);
#6022=EDGE_CURVE('',#4893,#4956,#2444,.T.);
#6023=EDGE_CURVE('',#4956,#4957,#2445,.T.);
#6024=EDGE_CURVE('',#4957,#4953,#2446,.T.);
#6025=EDGE_CURVE('',#4958,#4896,#2447,.T.);
#6026=EDGE_CURVE('',#4956,#4958,#2448,.T.);
#6027=EDGE_CURVE('',#4959,#4960,#2449,.T.);
#6028=EDGE_CURVE('',#4960,#4961,#2450,.T.);
#6029=EDGE_CURVE('',#4961,#4962,#2451,.T.);
#6030=EDGE_CURVE('',#4962,#4963,#2452,.T.);
#6031=EDGE_CURVE('',#4963,#4964,#2453,.T.);
#6032=EDGE_CURVE('',#4964,#4965,#2454,.T.);
#6033=EDGE_CURVE('',#4965,#4966,#2455,.T.);
#6034=EDGE_CURVE('',#4966,#4967,#2456,.T.);
#6035=EDGE_CURVE('',#4967,#4968,#2457,.T.);
#6036=EDGE_CURVE('',#4968,#4969,#2458,.T.);
#6037=EDGE_CURVE('',#4969,#4970,#2459,.T.);
#6038=EDGE_CURVE('',#4970,#4971,#2460,.T.);
#6039=EDGE_CURVE('',#4971,#4972,#2461,.T.);
#6040=EDGE_CURVE('',#4972,#4973,#2462,.T.);
#6041=EDGE_CURVE('',#4973,#4958,#2463,.T.);
#6042=EDGE_CURVE('',#4895,#4974,#2464,.T.);
#6043=EDGE_CURVE('',#4974,#4975,#2465,.T.);
#6044=EDGE_CURVE('',#4975,#4976,#2466,.T.);
#6045=EDGE_CURVE('',#4976,#4977,#2467,.T.);
#6046=EDGE_CURVE('',#4977,#4978,#2468,.T.);
#6047=EDGE_CURVE('',#4978,#4979,#2469,.T.);
#6048=EDGE_CURVE('',#4979,#4980,#2470,.T.);
#6049=EDGE_CURVE('',#4980,#4981,#2471,.T.);
#6050=EDGE_CURVE('',#4981,#4982,#2472,.T.);
#6051=EDGE_CURVE('',#4982,#4983,#2473,.T.);
#6052=EDGE_CURVE('',#4983,#4984,#2474,.T.);
#6053=EDGE_CURVE('',#4984,#4985,#2475,.T.);
#6054=EDGE_CURVE('',#4985,#4986,#2476,.T.);
#6055=EDGE_CURVE('',#4986,#4987,#2477,.T.);
#6056=EDGE_CURVE('',#4987,#4988,#2478,.T.);
#6057=EDGE_CURVE('',#4988,#4989,#2479,.T.);
#6058=EDGE_CURVE('',#4989,#4990,#2480,.T.);
#6059=EDGE_CURVE('',#4990,#4991,#2481,.T.);
#6060=EDGE_CURVE('',#4991,#4992,#2482,.T.);
#6061=EDGE_CURVE('',#4992,#4993,#2483,.T.);
#6062=EDGE_CURVE('',#4993,#4994,#2484,.T.);
#6063=EDGE_CURVE('',#4994,#4995,#2485,.T.);
#6064=EDGE_CURVE('',#4995,#4959,#2486,.T.);
#6065=EDGE_CURVE('',#4898,#4996,#2487,.T.);
#6066=EDGE_CURVE('',#4996,#4974,#2488,.T.);
#6067=EDGE_CURVE('',#4997,#4998,#2489,.T.);
#6068=EDGE_CURVE('',#4999,#4998,#2490,.T.);
#6069=EDGE_CURVE('',#5000,#4999,#2491,.T.);
#6070=EDGE_CURVE('',#4996,#5000,#2492,.T.);
#6071=EDGE_CURVE('',#4997,#4909,#2493,.T.);
#6072=EDGE_CURVE('',#4933,#5001,#2494,.T.);
#6073=EDGE_CURVE('',#5001,#5002,#4414,.T.);
#6074=EDGE_CURVE('',#5002,#4900,#2495,.T.);
#6075=EDGE_CURVE('',#5003,#5002,#2496,.T.);
#6076=EDGE_CURVE('',#5004,#5003,#2497,.T.);
#6077=EDGE_CURVE('',#5005,#5004,#2498,.T.);
#6078=EDGE_CURVE('',#5006,#5005,#2499,.T.);
#6079=EDGE_CURVE('',#5007,#5006,#2500,.T.);
#6080=EDGE_CURVE('',#5008,#5007,#2501,.T.);
#6081=EDGE_CURVE('',#5009,#5008,#2502,.T.);
#6082=EDGE_CURVE('',#5010,#5009,#2503,.T.);
#6083=EDGE_CURVE('',#5011,#5010,#2504,.T.);
#6084=EDGE_CURVE('',#5012,#5011,#2505,.T.);
#6085=EDGE_CURVE('',#5013,#5012,#2506,.T.);
#6086=EDGE_CURVE('',#5014,#5013,#2507,.T.);
#6087=EDGE_CURVE('',#5015,#5014,#2508,.T.);
#6088=EDGE_CURVE('',#4899,#5015,#2509,.T.);
#6089=EDGE_CURVE('',#5015,#5016,#4415,.T.);
#6090=EDGE_CURVE('',#5016,#4901,#2510,.T.);
#6091=EDGE_CURVE('',#5017,#5016,#2511,.T.);
#6092=EDGE_CURVE('',#4902,#5017,#2512,.T.);
#6093=EDGE_CURVE('',#5018,#5019,#4416,.T.);
#6094=EDGE_CURVE('',#5019,#5020,#4417,.T.);
#6095=EDGE_CURVE('',#5020,#4903,#2513,.T.);
#6096=EDGE_CURVE('',#5017,#5018,#4418,.T.);
#6097=EDGE_CURVE('',#5021,#5020,#2514,.T.);
#6098=EDGE_CURVE('',#5022,#5021,#2515,.T.);
#6099=EDGE_CURVE('',#5023,#5022,#2516,.T.);
#6100=EDGE_CURVE('',#5024,#5023,#2517,.T.);
#6101=EDGE_CURVE('',#5025,#5024,#2518,.T.);
#6102=EDGE_CURVE('',#5026,#5025,#2519,.T.);
#6103=EDGE_CURVE('',#5027,#5026,#2520,.T.);
#6104=EDGE_CURVE('',#5028,#5027,#2521,.T.);
#6105=EDGE_CURVE('',#5029,#5028,#2522,.T.);
#6106=EDGE_CURVE('',#4904,#5029,#2523,.T.);
#6107=EDGE_CURVE('',#5030,#4992,#4419,.T.);
#6108=EDGE_CURVE('',#4992,#5031,#4420,.T.);
#6109=EDGE_CURVE('',#5031,#4905,#2524,.T.);
#6110=EDGE_CURVE('',#5029,#5030,#4421,.T.);
#6111=EDGE_CURVE('',#5032,#5031,#2525,.T.);
#6112=EDGE_CURVE('',#4906,#5032,#2526,.T.);
#6113=EDGE_CURVE('',#5032,#5033,#4422,.T.);
#6114=EDGE_CURVE('',#5033,#4907,#2527,.T.);
#6115=EDGE_CURVE('',#5034,#5033,#2528,.T.);
#6116=EDGE_CURVE('',#5035,#5034,#2529,.T.);
#6117=EDGE_CURVE('',#5036,#5035,#2530,.T.);
#6118=EDGE_CURVE('',#5037,#5036,#2531,.T.);
#6119=EDGE_CURVE('',#5038,#5037,#2532,.T.);
#6120=EDGE_CURVE('',#5039,#5038,#2533,.T.);
#6121=EDGE_CURVE('',#5040,#5039,#2534,.T.);
#6122=EDGE_CURVE('',#5041,#5040,#2535,.T.);
#6123=EDGE_CURVE('',#5042,#5041,#2536,.T.);
#6124=EDGE_CURVE('',#5043,#5042,#2537,.T.);
#6125=EDGE_CURVE('',#5044,#5043,#2538,.T.);
#6126=EDGE_CURVE('',#5045,#5044,#2539,.T.);
#6127=EDGE_CURVE('',#5046,#5045,#2540,.T.);
#6128=EDGE_CURVE('',#4908,#5046,#2541,.T.);
#6129=EDGE_CURVE('',#5046,#4997,#4423,.T.);
#6130=EDGE_CURVE('',#4934,#5047,#4424,.T.);
#6131=EDGE_CURVE('',#5047,#4910,#4425,.T.);
#6132=EDGE_CURVE('',#5048,#5047,#2542,.T.);
#6133=EDGE_CURVE('',#4911,#5048,#2543,.T.);
#6134=EDGE_CURVE('',#4912,#5049,#2544,.T.);
#6135=EDGE_CURVE('',#5049,#5048,#4426,.T.);
#6136=EDGE_CURVE('',#5050,#5051,#270,.T.);
#6137=EDGE_CURVE('',#4913,#5050,#2545,.T.);
#6138=EDGE_CURVE('',#5051,#5049,#2546,.T.);
#6139=EDGE_CURVE('',#5052,#5050,#4427,.T.);
#6140=EDGE_CURVE('',#5052,#4914,#2547,.T.);
#6141=EDGE_CURVE('',#5053,#5052,#271,.T.);
#6142=EDGE_CURVE('',#5053,#5054,#2548,.T.);
#6143=EDGE_CURVE('',#5055,#5054,#272,.T.);
#6144=EDGE_CURVE('',#5055,#4915,#2549,.T.);
#6145=EDGE_CURVE('',#5056,#5055,#4428,.T.);
#6146=EDGE_CURVE('',#5056,#4916,#2550,.T.);
#6147=EDGE_CURVE('',#4917,#5057,#2551,.T.);
#6148=EDGE_CURVE('',#5058,#5056,#273,.T.);
#6149=EDGE_CURVE('',#5057,#5058,#2552,.T.);
#6150=EDGE_CURVE('',#4918,#5059,#2553,.T.);
#6151=EDGE_CURVE('',#5059,#5057,#4429,.T.);
#6152=EDGE_CURVE('',#5060,#5061,#274,.T.);
#6153=EDGE_CURVE('',#4919,#5060,#2554,.T.);
#6154=EDGE_CURVE('',#5061,#5059,#2555,.T.);
#6155=EDGE_CURVE('',#5062,#5060,#4430,.T.);
#6156=EDGE_CURVE('',#5062,#4920,#2556,.T.);
#6157=EDGE_CURVE('',#5063,#5062,#275,.T.);
#6158=EDGE_CURVE('',#5063,#5064,#2557,.T.);
#6159=EDGE_CURVE('',#5065,#5064,#276,.T.);
#6160=EDGE_CURVE('',#5065,#4921,#2558,.T.);
#6161=EDGE_CURVE('',#5066,#5065,#4431,.T.);
#6162=EDGE_CURVE('',#5066,#4922,#2559,.T.);
#6163=EDGE_CURVE('',#4923,#5067,#2560,.T.);
#6164=EDGE_CURVE('',#5068,#5066,#277,.T.);
#6165=EDGE_CURVE('',#5067,#5068,#2561,.T.);
#6166=EDGE_CURVE('',#4924,#5069,#2562,.T.);
#6167=EDGE_CURVE('',#5069,#5067,#4432,.T.);
#6168=EDGE_CURVE('',#5070,#5071,#278,.T.);
#6169=EDGE_CURVE('',#4925,#5070,#2563,.T.);
#6170=EDGE_CURVE('',#5071,#5069,#2564,.T.);
#6171=EDGE_CURVE('',#5072,#5070,#4433,.T.);
#6172=EDGE_CURVE('',#5072,#4926,#2565,.T.);
#6173=EDGE_CURVE('',#5073,#5072,#279,.T.);
#6174=EDGE_CURVE('',#5073,#5074,#2566,.T.);
#6175=EDGE_CURVE('',#5075,#5074,#280,.T.);
#6176=EDGE_CURVE('',#5075,#4927,#2567,.T.);
#6177=EDGE_CURVE('',#5076,#5075,#4434,.T.);
#6178=EDGE_CURVE('',#5076,#4928,#2568,.T.);
#6179=EDGE_CURVE('',#4929,#5077,#2569,.T.);
#6180=EDGE_CURVE('',#5078,#5076,#281,.T.);
#6181=EDGE_CURVE('',#5077,#5078,#2570,.T.);
#6182=EDGE_CURVE('',#4930,#5079,#2571,.T.);
#6183=EDGE_CURVE('',#5079,#5077,#4435,.T.);
#6184=EDGE_CURVE('',#5080,#5079,#2572,.T.);
#6185=EDGE_CURVE('',#4931,#5080,#4436,.T.);
#6186=EDGE_CURVE('',#5080,#4935,#4437,.T.);
#6187=EDGE_CURVE('',#5081,#4936,#2573,.T.);
#6188=EDGE_CURVE('',#5082,#5081,#2574,.T.);
#6189=EDGE_CURVE('',#5083,#5082,#2575,.T.);
#6190=EDGE_CURVE('',#5084,#5083,#2576,.T.);
#6191=EDGE_CURVE('',#5001,#5084,#2577,.T.);
#6192=EDGE_CURVE('',#5085,#5086,#4438,.T.);
#6193=EDGE_CURVE('',#5087,#5085,#2578,.T.);
#6194=EDGE_CURVE('',#5088,#5087,#2579,.T.);
#6195=EDGE_CURVE('',#5089,#5088,#2580,.T.);
#6196=EDGE_CURVE('',#5090,#5089,#4439,.T.);
#6197=EDGE_CURVE('',#5091,#5090,#2581,.T.);
#6198=EDGE_CURVE('',#5092,#5091,#2582,.T.);
#6199=EDGE_CURVE('',#5093,#5092,#2583,.T.);
#6200=EDGE_CURVE('',#5094,#5093,#4440,.T.);
#6201=EDGE_CURVE('',#5095,#5094,#2584,.T.);
#6202=EDGE_CURVE('',#5096,#5095,#2585,.T.);
#6203=EDGE_CURVE('',#5097,#5096,#2586,.T.);
#6204=EDGE_CURVE('',#5098,#5097,#4441,.T.);
#6205=EDGE_CURVE('',#4934,#5098,#2587,.T.);
#6206=EDGE_CURVE('',#5086,#4935,#2588,.T.);
#6207=EDGE_CURVE('',#5099,#5081,#2589,.T.);
#6208=EDGE_CURVE('',#4938,#5099,#2590,.T.);
#6209=EDGE_CURVE('',#5100,#4940,#2591,.T.);
#6210=EDGE_CURVE('',#5101,#5100,#2592,.T.);
#6211=EDGE_CURVE('',#4937,#5101,#2593,.T.);
#6212=EDGE_CURVE('',#5102,#5103,#2594,.T.);
#6213=EDGE_CURVE('',#5103,#5104,#2595,.T.);
#6214=EDGE_CURVE('',#5104,#5105,#2596,.T.);
#6215=EDGE_CURVE('',#5105,#5106,#2597,.T.);
#6216=EDGE_CURVE('',#5106,#5107,#2598,.T.);
#6217=EDGE_CURVE('',#5107,#5108,#2599,.T.);
#6218=EDGE_CURVE('',#5108,#5109,#2600,.T.);
#6219=EDGE_CURVE('',#5109,#5110,#2601,.T.);
#6220=EDGE_CURVE('',#5110,#5018,#2602,.T.);
#6221=EDGE_CURVE('',#5018,#5111,#2603,.T.);
#6222=EDGE_CURVE('',#5111,#5112,#2604,.T.);
#6223=EDGE_CURVE('',#5112,#5113,#2605,.T.);
#6224=EDGE_CURVE('',#5113,#5114,#2606,.T.);
#6225=EDGE_CURVE('',#5114,#5115,#2607,.T.);
#6226=EDGE_CURVE('',#5115,#5116,#2608,.T.);
#6227=EDGE_CURVE('',#5116,#5117,#2609,.T.);
#6228=EDGE_CURVE('',#5117,#5118,#2610,.T.);
#6229=EDGE_CURVE('',#5118,#5119,#2611,.T.);
#6230=EDGE_CURVE('',#5119,#5120,#2612,.T.);
#6231=EDGE_CURVE('',#5120,#5121,#2613,.T.);
#6232=EDGE_CURVE('',#5121,#5122,#2614,.T.);
#6233=EDGE_CURVE('',#5122,#5123,#2615,.T.);
#6234=EDGE_CURVE('',#5123,#5124,#2616,.T.);
#6235=EDGE_CURVE('',#5124,#5125,#2617,.T.);
#6236=EDGE_CURVE('',#5125,#5126,#2618,.T.);
#6237=EDGE_CURVE('',#5126,#5127,#2619,.T.);
#6238=EDGE_CURVE('',#5127,#5099,#2620,.T.);
#6239=EDGE_CURVE('',#5101,#5128,#2621,.T.);
#6240=EDGE_CURVE('',#5128,#5129,#2622,.T.);
#6241=EDGE_CURVE('',#5129,#5130,#2623,.T.);
#6242=EDGE_CURVE('',#5130,#5131,#2624,.T.);
#6243=EDGE_CURVE('',#5131,#5132,#2625,.T.);
#6244=EDGE_CURVE('',#5132,#5133,#2626,.T.);
#6245=EDGE_CURVE('',#5133,#5134,#2627,.T.);
#6246=EDGE_CURVE('',#5134,#5135,#2628,.T.);
#6247=EDGE_CURVE('',#5135,#5136,#2629,.T.);
#6248=EDGE_CURVE('',#5136,#5102,#2630,.T.);
#6249=EDGE_CURVE('',#4944,#5137,#2631,.T.);
#6250=EDGE_CURVE('',#5138,#5137,#2632,.T.);
#6251=EDGE_CURVE('',#5138,#5139,#2633,.T.);
#6252=EDGE_CURVE('',#5139,#5140,#2634,.T.);
#6253=EDGE_CURVE('',#5140,#5100,#2635,.T.);
#6254=EDGE_CURVE('',#5141,#5142,#2636,.T.);
#6255=EDGE_CURVE('',#5142,#5143,#2637,.T.);
#6256=EDGE_CURVE('',#5143,#4943,#2638,.T.);
#6257=EDGE_CURVE('',#4942,#5144,#2639,.T.);
#6258=EDGE_CURVE('',#5144,#5145,#2640,.T.);
#6259=EDGE_CURVE('',#5145,#5146,#2641,.T.);
#6260=EDGE_CURVE('',#5146,#5147,#2642,.T.);
#6261=EDGE_CURVE('',#5147,#5148,#2643,.T.);
#6262=EDGE_CURVE('',#5148,#5149,#2644,.T.);
#6263=EDGE_CURVE('',#5149,#5150,#2645,.T.);
#6264=EDGE_CURVE('',#5150,#5151,#2646,.T.);
#6265=EDGE_CURVE('',#5151,#5152,#2647,.T.);
#6266=EDGE_CURVE('',#5152,#5153,#2648,.T.);
#6267=EDGE_CURVE('',#5153,#5154,#2649,.T.);
#6268=EDGE_CURVE('',#5154,#5141,#2650,.T.);
#6269=EDGE_CURVE('',#4941,#5155,#2651,.T.);
#6270=EDGE_CURVE('',#5155,#5144,#4442,.T.);
#6271=EDGE_CURVE('',#4952,#5156,#2652,.T.);
#6272=EDGE_CURVE('',#5156,#5155,#2653,.T.);
#6273=EDGE_CURVE('',#4951,#5157,#2654,.T.);
#6274=EDGE_CURVE('',#5157,#5158,#4443,.T.);
#6275=EDGE_CURVE('',#5158,#5104,#4444,.T.);
#6276=EDGE_CURVE('',#5104,#5156,#4445,.T.);
#6277=EDGE_CURVE('',#5159,#5160,#2655,.T.);
#6278=EDGE_CURVE('',#5160,#5157,#2656,.T.);
#6279=EDGE_CURVE('',#4950,#5161,#2657,.T.);
#6280=EDGE_CURVE('',#5161,#5162,#2658,.T.);
#6281=EDGE_CURVE('',#5162,#5163,#2659,.T.);
#6282=EDGE_CURVE('',#5163,#5164,#2660,.T.);
#6283=EDGE_CURVE('',#5164,#5165,#2661,.T.);
#6284=EDGE_CURVE('',#5165,#5166,#2662,.T.);
#6285=EDGE_CURVE('',#5166,#5167,#2663,.T.);
#6286=EDGE_CURVE('',#5167,#5159,#2664,.T.);
#6287=EDGE_CURVE('',#4949,#5168,#2665,.T.);
#6288=EDGE_CURVE('',#5168,#4962,#4446,.T.);
#6289=EDGE_CURVE('',#4962,#5169,#4447,.T.);
#6290=EDGE_CURVE('',#5169,#5161,#4448,.T.);
#6291=EDGE_CURVE('',#4948,#5170,#2666,.T.);
#6292=EDGE_CURVE('',#5170,#5168,#2667,.T.);
#6293=EDGE_CURVE('',#4947,#5171,#2668,.T.);
#6294=EDGE_CURVE('',#5171,#5170,#4449,.T.);
#6295=EDGE_CURVE('',#5172,#5173,#2669,.T.);
#6296=EDGE_CURVE('',#5173,#5171,#2670,.T.);
#6297=EDGE_CURVE('',#4946,#5174,#2671,.T.);
#6298=EDGE_CURVE('',#5174,#5175,#2672,.T.);
#6299=EDGE_CURVE('',#5175,#5176,#2673,.T.);
#6300=EDGE_CURVE('',#5176,#5177,#2674,.T.);
#6301=EDGE_CURVE('',#5177,#5178,#2675,.T.);
#6302=EDGE_CURVE('',#5178,#5179,#2676,.T.);
#6303=EDGE_CURVE('',#5179,#5180,#2677,.T.);
#6304=EDGE_CURVE('',#5180,#5181,#2678,.T.);
#6305=EDGE_CURVE('',#5181,#5182,#2679,.T.);
#6306=EDGE_CURVE('',#5182,#5183,#2680,.T.);
#6307=EDGE_CURVE('',#5183,#5184,#2681,.T.);
#6308=EDGE_CURVE('',#5184,#5172,#2682,.T.);
#6309=EDGE_CURVE('',#4955,#5174,#4450,.T.);
#6310=EDGE_CURVE('',#5143,#5137,#4451,.T.);
#6311=EDGE_CURVE('',#5185,#4953,#2683,.T.);
#6312=EDGE_CURVE('',#5186,#5185,#2684,.T.);
#6313=EDGE_CURVE('',#4954,#5186,#2685,.T.);
#6314=EDGE_CURVE('',#4973,#4957,#2686,.T.);
#6315=EDGE_CURVE('',#5185,#4972,#2687,.T.);
#6316=EDGE_CURVE('',#4960,#5187,#2688,.T.);
#6317=EDGE_CURVE('',#5187,#5169,#2689,.T.);
#6318=EDGE_CURVE('',#5169,#4961,#2690,.T.);
#6319=EDGE_CURVE('',#5188,#5189,#2691,.T.);
#6320=EDGE_CURVE('',#5187,#5188,#2692,.T.);
#6321=EDGE_CURVE('',#5190,#4959,#4452,.T.);
#6322=EDGE_CURVE('',#5189,#5190,#2693,.T.);
#6323=EDGE_CURVE('',#5191,#5190,#2694,.T.);
#6324=EDGE_CURVE('',#4995,#5191,#4453,.T.);
#6325=EDGE_CURVE('',#5192,#5191,#2695,.T.);
#6326=EDGE_CURVE('',#4994,#5193,#2696,.T.);
#6327=EDGE_CURVE('',#5193,#5194,#2697,.T.);
#6328=EDGE_CURVE('',#5194,#5192,#2698,.T.);
#6329=EDGE_CURVE('',#5193,#5030,#2699,.T.);
#6330=EDGE_CURVE('',#5030,#4993,#2700,.T.);
#6331=EDGE_CURVE('',#4991,#5195,#2701,.T.);
#6332=EDGE_CURVE('',#5195,#5196,#2702,.T.);
#6333=EDGE_CURVE('',#5196,#5034,#2703,.T.);
#6334=EDGE_CURVE('',#5197,#5195,#2704,.T.);
#6335=EDGE_CURVE('',#4990,#5197,#2705,.T.);
#6336=EDGE_CURVE('',#5198,#4988,#2706,.T.);
#6337=EDGE_CURVE('',#5199,#5198,#2707,.T.);
#6338=EDGE_CURVE('',#4989,#5199,#2708,.T.);
#6339=EDGE_CURVE('',#5200,#4987,#2709,.T.);
#6340=EDGE_CURVE('',#5198,#5200,#2710,.T.);
#6341=EDGE_CURVE('',#5200,#5201,#2711,.T.);
#6342=EDGE_CURVE('',#5201,#4986,#2712,.T.);
#6343=EDGE_CURVE('',#5202,#5203,#2713,.T.);
#6344=EDGE_CURVE('',#5203,#4985,#2714,.T.);
#6345=EDGE_CURVE('',#4984,#5202,#2715,.T.);
#6346=EDGE_CURVE('',#5035,#5204,#2716,.T.);
#6347=EDGE_CURVE('',#5204,#5202,#2717,.T.);
#6348=EDGE_CURVE('',#4983,#5205,#2718,.T.);
#6349=EDGE_CURVE('',#5205,#5036,#2719,.T.);
#6350=EDGE_CURVE('',#5206,#4982,#2720,.T.);
#6351=EDGE_CURVE('',#5206,#4983,#2721,.T.);
#6352=EDGE_CURVE('',#4981,#5040,#2722,.T.);
#6353=EDGE_CURVE('',#5039,#5207,#2723,.T.);
#6354=EDGE_CURVE('',#5207,#4982,#2724,.T.);
#6355=EDGE_CURVE('',#5041,#4980,#2725,.T.);
#6356=EDGE_CURVE('',#4979,#5042,#2726,.T.);
#6357=EDGE_CURVE('',#5043,#4978,#2727,.T.);
#6358=EDGE_CURVE('',#4977,#5208,#2728,.T.);
#6359=EDGE_CURVE('',#5208,#5044,#2729,.T.);
#6360=EDGE_CURVE('',#5209,#4976,#2730,.T.);
#6361=EDGE_CURVE('',#5209,#4977,#2731,.T.);
#6362=EDGE_CURVE('',#4975,#5000,#2732,.T.);
#6363=EDGE_CURVE('',#4999,#5210,#2733,.T.);
#6364=EDGE_CURVE('',#5210,#4976,#2734,.T.);
#6365=EDGE_CURVE('',#4971,#5211,#2735,.T.);
#6366=EDGE_CURVE('',#4972,#5211,#2736,.T.);
#6367=EDGE_CURVE('',#5177,#4970,#2737,.T.);
#6368=EDGE_CURVE('',#5212,#5176,#2738,.T.);
#6369=EDGE_CURVE('',#4971,#5212,#2739,.T.);
#6370=EDGE_CURVE('',#4969,#5178,#2740,.T.);
#6371=EDGE_CURVE('',#5179,#4968,#2741,.T.);
#6372=EDGE_CURVE('',#4967,#5180,#2742,.T.);
#6373=EDGE_CURVE('',#5213,#4966,#2743,.T.);
#6374=EDGE_CURVE('',#5181,#5213,#2744,.T.);
#6375=EDGE_CURVE('',#4965,#5214,#2745,.T.);
#6376=EDGE_CURVE('',#4966,#5214,#2746,.T.);
#6377=EDGE_CURVE('',#5172,#4964,#2747,.T.);
#6378=EDGE_CURVE('',#5215,#5184,#2748,.T.);
#6379=EDGE_CURVE('',#4965,#5215,#2749,.T.);
#6380=EDGE_CURVE('',#4963,#5173,#2750,.T.);
#6381=EDGE_CURVE('',#5216,#5210,#2751,.T.);
#6382=EDGE_CURVE('',#4998,#5216,#2752,.T.);
#6383=EDGE_CURVE('',#5217,#5019,#2753,.T.);
#6384=EDGE_CURVE('',#5218,#5217,#2754,.T.);
#6385=EDGE_CURVE('',#5219,#5218,#2755,.T.);
#6386=EDGE_CURVE('',#5021,#5219,#2756,.T.);
#6387=EDGE_CURVE('',#5220,#5010,#2757,.T.);
#6388=EDGE_CURVE('',#5221,#5220,#2758,.T.);
#6389=EDGE_CURVE('',#5222,#5221,#2759,.T.);
#6390=EDGE_CURVE('',#5011,#5222,#2760,.T.);
#6391=EDGE_CURVE('',#5223,#5084,#2761,.T.);
#6392=EDGE_CURVE('',#5224,#5223,#2762,.T.);
#6393=EDGE_CURVE('',#5225,#5224,#2763,.T.);
#6394=EDGE_CURVE('',#5003,#5225,#2764,.T.);
#6395=EDGE_CURVE('',#5226,#5028,#2765,.T.);
#6396=EDGE_CURVE('',#5227,#5226,#2766,.T.);
#6397=EDGE_CURVE('',#5228,#5227,#2767,.T.);
#6398=EDGE_CURVE('',#5030,#5228,#2768,.T.);
#6399=EDGE_CURVE('',#5229,#5037,#2769,.T.);
#6400=EDGE_CURVE('',#5230,#5229,#2770,.T.);
#6401=EDGE_CURVE('',#5231,#5230,#2771,.T.);
#6402=EDGE_CURVE('',#5038,#5231,#2772,.T.);
#6403=EDGE_CURVE('',#5232,#5045,#2773,.T.);
#6404=EDGE_CURVE('',#5233,#5232,#2774,.T.);
#6405=EDGE_CURVE('',#5216,#5233,#2775,.T.);
#6406=EDGE_CURVE('',#5225,#5234,#2776,.T.);
#6407=EDGE_CURVE('',#5234,#5004,#2777,.T.);
#6408=EDGE_CURVE('',#5006,#5123,#2778,.T.);
#6409=EDGE_CURVE('',#5124,#5005,#2779,.T.);
#6410=EDGE_CURVE('',#5122,#5007,#2780,.T.);
#6411=EDGE_CURVE('',#5008,#5121,#2781,.T.);
#6412=EDGE_CURVE('',#5235,#5220,#2782,.T.);
#6413=EDGE_CURVE('',#5009,#5235,#2783,.T.);
#6414=EDGE_CURVE('',#5222,#5236,#2784,.T.);
#6415=EDGE_CURVE('',#5236,#5012,#2785,.T.);
#6416=EDGE_CURVE('',#5014,#5237,#2786,.T.);
#6417=EDGE_CURVE('',#5238,#5013,#2787,.T.);
#6418=EDGE_CURVE('',#5237,#5238,#2788,.T.);
#6419=EDGE_CURVE('',#5237,#5239,#2789,.T.);
#6420=EDGE_CURVE('',#5239,#5111,#2790,.T.);
#6421=EDGE_CURVE('',#5019,#5110,#2791,.T.);
#6422=EDGE_CURVE('',#5219,#5240,#2792,.T.);
#6423=EDGE_CURVE('',#5240,#5022,#2793,.T.);
#6424=EDGE_CURVE('',#5024,#5241,#2794,.T.);
#6425=EDGE_CURVE('',#5242,#5023,#2795,.T.);
#6426=EDGE_CURVE('',#5241,#5242,#2796,.T.);
#6427=EDGE_CURVE('',#5243,#5025,#2797,.T.);
#6428=EDGE_CURVE('',#5241,#5243,#2798,.T.);
#6429=EDGE_CURVE('',#5026,#5244,#2799,.T.);
#6430=EDGE_CURVE('',#5244,#5243,#2800,.T.);
#6431=EDGE_CURVE('',#5245,#5226,#2801,.T.);
#6432=EDGE_CURVE('',#5027,#5245,#2802,.T.);
#6433=EDGE_CURVE('',#5204,#5196,#2803,.T.);
#6434=EDGE_CURVE('',#5205,#5229,#2804,.T.);
#6435=EDGE_CURVE('',#5231,#5207,#2805,.T.);
#6436=EDGE_CURVE('',#5208,#5232,#2806,.T.);
#6437=EDGE_CURVE('',#5098,#5048,#4454,.T.);
#6438=EDGE_CURVE('',#5097,#5049,#4455,.T.);
#6439=EDGE_CURVE('',#5096,#5051,#4456,.T.);
#6440=EDGE_CURVE('',#5053,#5096,#4457,.T.);
#6441=EDGE_CURVE('',#5095,#5054,#4458,.T.);
#6442=EDGE_CURVE('',#5094,#5057,#4459,.T.);
#6443=EDGE_CURVE('',#5058,#5095,#4460,.T.);
#6444=EDGE_CURVE('',#5093,#5059,#4461,.T.);
#6445=EDGE_CURVE('',#5092,#5061,#4462,.T.);
#6446=EDGE_CURVE('',#5063,#5092,#4463,.T.);
#6447=EDGE_CURVE('',#5091,#5064,#4464,.T.);
#6448=EDGE_CURVE('',#5090,#5067,#4465,.T.);
#6449=EDGE_CURVE('',#5068,#5091,#4466,.T.);
#6450=EDGE_CURVE('',#5089,#5069,#4467,.T.);
#6451=EDGE_CURVE('',#5088,#5071,#4468,.T.);
#6452=EDGE_CURVE('',#5073,#5088,#4469,.T.);
#6453=EDGE_CURVE('',#5087,#5074,#4470,.T.);
#6454=EDGE_CURVE('',#5085,#5077,#4471,.T.);
#6455=EDGE_CURVE('',#5078,#5087,#4472,.T.);
#6456=EDGE_CURVE('',#5086,#5079,#4473,.T.);
#6457=EDGE_CURVE('',#5082,#5127,#2807,.T.);
#6458=EDGE_CURVE('',#5126,#5246,#2808,.T.);
#6459=EDGE_CURVE('',#5246,#5083,#2809,.T.);
#6460=EDGE_CURVE('',#5246,#5223,#2810,.T.);
#6461=EDGE_CURVE('',#5140,#5128,#2811,.T.);
#6462=EDGE_CURVE('',#5145,#5103,#2812,.T.);
#6463=EDGE_CURVE('',#5102,#5146,#2813,.T.);
#6464=EDGE_CURVE('',#5247,#5136,#2814,.T.);
#6465=EDGE_CURVE('',#5147,#5247,#2815,.T.);
#6466=EDGE_CURVE('',#5135,#5248,#2816,.T.);
#6467=EDGE_CURVE('',#5136,#5248,#2817,.T.);
#6468=EDGE_CURVE('',#5151,#5134,#2818,.T.);
#6469=EDGE_CURVE('',#5249,#5150,#2819,.T.);
#6470=EDGE_CURVE('',#5135,#5249,#2820,.T.);
#6471=EDGE_CURVE('',#5133,#5152,#2821,.T.);
#6472=EDGE_CURVE('',#5153,#5132,#2822,.T.);
#6473=EDGE_CURVE('',#5131,#5154,#2823,.T.);
#6474=EDGE_CURVE('',#5250,#5130,#2824,.T.);
#6475=EDGE_CURVE('',#5141,#5250,#2825,.T.);
#6476=EDGE_CURVE('',#5129,#5251,#2826,.T.);
#6477=EDGE_CURVE('',#5130,#5251,#2827,.T.);
#6478=EDGE_CURVE('',#5252,#5139,#2828,.T.);
#6479=EDGE_CURVE('',#5129,#5252,#2829,.T.);
#6480=EDGE_CURVE('',#5125,#5253,#2830,.T.);
#6481=EDGE_CURVE('',#5253,#5126,#2831,.T.);
#6482=EDGE_CURVE('',#5234,#5125,#2832,.T.);
#6483=EDGE_CURVE('',#5120,#5235,#2833,.T.);
#6484=EDGE_CURVE('',#5119,#5254,#2834,.T.);
#6485=EDGE_CURVE('',#5254,#5120,#2835,.T.);
#6486=EDGE_CURVE('',#5236,#5119,#2836,.T.);
#6487=EDGE_CURVE('',#5118,#5255,#2837,.T.);
#6488=EDGE_CURVE('',#5255,#5238,#2838,.T.);
#6489=EDGE_CURVE('',#5256,#5255,#2839,.T.);
#6490=EDGE_CURVE('',#5117,#5256,#2840,.T.);
#6491=EDGE_CURVE('',#5257,#5115,#2841,.T.);
#6492=EDGE_CURVE('',#5258,#5257,#2842,.T.);
#6493=EDGE_CURVE('',#5116,#5258,#2843,.T.);
#6494=EDGE_CURVE('',#5259,#5114,#2844,.T.);
#6495=EDGE_CURVE('',#5257,#5259,#2845,.T.);
#6496=EDGE_CURVE('',#5259,#5260,#2846,.T.);
#6497=EDGE_CURVE('',#5260,#5113,#2847,.T.);
#6498=EDGE_CURVE('',#5239,#5261,#2848,.T.);
#6499=EDGE_CURVE('',#5261,#5112,#2849,.T.);
#6500=EDGE_CURVE('',#5262,#5109,#2850,.T.);
#6501=EDGE_CURVE('',#5019,#5262,#2851,.T.);
#6502=EDGE_CURVE('',#5108,#5263,#4474,.T.);
#6503=EDGE_CURVE('',#5263,#5264,#2852,.T.);
#6504=EDGE_CURVE('',#5264,#5265,#2853,.T.);
#6505=EDGE_CURVE('',#5265,#5262,#2854,.T.);
#6506=EDGE_CURVE('',#5107,#5266,#4475,.T.);
#6507=EDGE_CURVE('',#5266,#5263,#2855,.T.);
#6508=EDGE_CURVE('',#5267,#5106,#2856,.T.);
#6509=EDGE_CURVE('',#5268,#5267,#2857,.T.);
#6510=EDGE_CURVE('',#5269,#5268,#2858,.T.);
#6511=EDGE_CURVE('',#5266,#5269,#2859,.T.);
#6512=EDGE_CURVE('',#5105,#5158,#2860,.T.);
#6513=EDGE_CURVE('',#5158,#5267,#2861,.T.);
#6514=EDGE_CURVE('',#5270,#5138,#2862,.T.);
#6515=EDGE_CURVE('',#5252,#5270,#2863,.T.);
#6516=EDGE_CURVE('',#5271,#5158,#2864,.T.);
#6517=EDGE_CURVE('',#5160,#5272,#2865,.T.);
#6518=EDGE_CURVE('',#5272,#5273,#2866,.T.);
#6519=EDGE_CURVE('',#5273,#5271,#2867,.T.);
#6520=EDGE_CURVE('',#5274,#5275,#2868,.T.);
#6521=EDGE_CURVE('',#5275,#5149,#2869,.T.);
#6522=EDGE_CURVE('',#5148,#5276,#2870,.T.);
#6523=EDGE_CURVE('',#5276,#5274,#2871,.T.);
#6524=EDGE_CURVE('',#5142,#5277,#2872,.T.);
#6525=EDGE_CURVE('',#5277,#5278,#2873,.T.);
#6526=EDGE_CURVE('',#5278,#5270,#2874,.T.);
#6527=EDGE_CURVE('',#5279,#5162,#2875,.T.);
#6528=EDGE_CURVE('',#5169,#5280,#2876,.T.);
#6529=EDGE_CURVE('',#5280,#5281,#2877,.T.);
#6530=EDGE_CURVE('',#5281,#5279,#2878,.T.);
#6531=EDGE_CURVE('',#5282,#5283,#2879,.T.);
#6532=EDGE_CURVE('',#5283,#5183,#2880,.T.);
#6533=EDGE_CURVE('',#5182,#5284,#2881,.T.);
#6534=EDGE_CURVE('',#5284,#5282,#2882,.T.);
#6535=EDGE_CURVE('',#5285,#5175,#2883,.T.);
#6536=EDGE_CURVE('',#5186,#5286,#2884,.T.);
#6537=EDGE_CURVE('',#5286,#5285,#2885,.T.);
#6538=EDGE_CURVE('',#5277,#5250,#2886,.T.);
#6539=EDGE_CURVE('',#5249,#5275,#2887,.T.);
#6540=EDGE_CURVE('',#5276,#5247,#2888,.T.);
#6541=EDGE_CURVE('',#5287,#5159,#2889,.T.);
#6542=EDGE_CURVE('',#5272,#5287,#2890,.T.);
#6543=EDGE_CURVE('',#5166,#5288,#2891,.T.);
#6544=EDGE_CURVE('',#5288,#5289,#2892,.T.);
#6545=EDGE_CURVE('',#5289,#5167,#2893,.T.);
#6546=EDGE_CURVE('',#5290,#5165,#2894,.T.);
#6547=EDGE_CURVE('',#5288,#5290,#2895,.T.);
#6548=EDGE_CURVE('',#5164,#5291,#2896,.T.);
#6549=EDGE_CURVE('',#5291,#5290,#2897,.T.);
#6550=EDGE_CURVE('',#5292,#5279,#2898,.T.);
#6551=EDGE_CURVE('',#5163,#5292,#2899,.T.);
#6552=EDGE_CURVE('',#5215,#5283,#2900,.T.);
#6553=EDGE_CURVE('',#5284,#5213,#2901,.T.);
#6554=EDGE_CURVE('',#5212,#5285,#2902,.T.);
#6555=EDGE_CURVE('',#5286,#5211,#2903,.T.);
#6556=EDGE_CURVE('',#5280,#5188,#2904,.T.);
#6557=EDGE_CURVE('',#5293,#5189,#2905,.T.);
#6558=EDGE_CURVE('',#5281,#5293,#2906,.T.);
#6559=EDGE_CURVE('',#5294,#5264,#2907,.T.);
#6560=EDGE_CURVE('',#5269,#5295,#2908,.T.);
#6561=EDGE_CURVE('',#5295,#5289,#2909,.T.);
#6562=EDGE_CURVE('',#5291,#5296,#2910,.T.);
#6563=EDGE_CURVE('',#5296,#5189,#2911,.T.);
#6564=EDGE_CURVE('',#5192,#5297,#2912,.T.);
#6565=EDGE_CURVE('',#5297,#5244,#2913,.T.);
#6566=EDGE_CURVE('',#5242,#5294,#2914,.T.);
#6567=EDGE_CURVE('',#5227,#5298,#2915,.T.);
#6568=EDGE_CURVE('',#5298,#5192,#2916,.T.);
#6569=EDGE_CURVE('',#5194,#5228,#2917,.T.);
#6570=EDGE_CURVE('',#5197,#5203,#2918,.T.);
#6571=EDGE_CURVE('',#5201,#5199,#2919,.T.);
#6572=EDGE_CURVE('',#5299,#5300,#2920,.T.);
#6573=EDGE_CURVE('',#5301,#5299,#2921,.T.);
#6574=EDGE_CURVE('',#5302,#5301,#2922,.T.);
#6575=EDGE_CURVE('',#5300,#5302,#2923,.T.);
#6576=EDGE_CURVE('',#5206,#5230,#2924,.T.);
#6577=EDGE_CURVE('',#5209,#5233,#2925,.T.);
#6578=EDGE_CURVE('',#5282,#5214,#2926,.T.);
#6579=EDGE_CURVE('',#5265,#5217,#2927,.T.);
#6580=EDGE_CURVE('',#5264,#5303,#2928,.T.);
#6581=EDGE_CURVE('',#5303,#5218,#2929,.T.);
#6582=EDGE_CURVE('',#5303,#5294,#2930,.T.);
#6583=EDGE_CURVE('',#5294,#5240,#2931,.T.);
#6584=EDGE_CURVE('',#5254,#5221,#2932,.T.);
#6585=EDGE_CURVE('',#5253,#5224,#2933,.T.);
#6586=EDGE_CURVE('',#5245,#5297,#2934,.T.);
#6587=EDGE_CURVE('',#5297,#5298,#2935,.T.);
#6588=EDGE_CURVE('',#5256,#5261,#2936,.T.);
#6589=EDGE_CURVE('',#5053,#5051,#282,.T.);
#6590=EDGE_CURVE('',#5058,#5054,#283,.T.);
#6591=EDGE_CURVE('',#5063,#5061,#284,.T.);
#6592=EDGE_CURVE('',#5068,#5064,#285,.T.);
#6593=EDGE_CURVE('',#5073,#5071,#286,.T.);
#6594=EDGE_CURVE('',#5078,#5074,#287,.T.);
#6595=EDGE_CURVE('',#5274,#5248,#2937,.T.);
#6596=EDGE_CURVE('',#5278,#5251,#2938,.T.);
#6597=EDGE_CURVE('',#5260,#5258,#2939,.T.);
#6598=EDGE_CURVE('',#5304,#5305,#2940,.T.);
#6599=EDGE_CURVE('',#5306,#5304,#2941,.T.);
#6600=EDGE_CURVE('',#5307,#5306,#2942,.T.);
#6601=EDGE_CURVE('',#5305,#5307,#2943,.T.);
#6602=EDGE_CURVE('',#5268,#5271,#2944,.T.);
#6603=EDGE_CURVE('',#5308,#5273,#2945,.T.);
#6604=EDGE_CURVE('',#5269,#5308,#2946,.T.);
#6605=EDGE_CURVE('',#5308,#5295,#2947,.T.);
#6606=EDGE_CURVE('',#5295,#5287,#2948,.T.);
#6607=EDGE_CURVE('',#5296,#5293,#2949,.T.);
#6608=EDGE_CURVE('',#5292,#5296,#2950,.T.);
#6609=EDGE_CURVE('',#5309,#5310,#2951,.T.);
#6610=EDGE_CURVE('',#5310,#5300,#2952,.T.);
#6611=EDGE_CURVE('',#5302,#5309,#2953,.T.);
#6612=EDGE_CURVE('',#5310,#5311,#2954,.T.);
#6613=EDGE_CURVE('',#5311,#5299,#2955,.T.);
#6614=EDGE_CURVE('',#5311,#5312,#2956,.T.);
#6615=EDGE_CURVE('',#5312,#5301,#2957,.T.);
#6616=EDGE_CURVE('',#5312,#5309,#2958,.T.);
#6617=EDGE_CURVE('',#5313,#5314,#2959,.T.);
#6618=EDGE_CURVE('',#5314,#5305,#2960,.T.);
#6619=EDGE_CURVE('',#5307,#5313,#2961,.T.);
#6620=EDGE_CURVE('',#5314,#5315,#2962,.T.);
#6621=EDGE_CURVE('',#5315,#5304,#2963,.T.);
#6622=EDGE_CURVE('',#5315,#5316,#2964,.T.);
#6623=EDGE_CURVE('',#5316,#5306,#2965,.T.);
#6624=EDGE_CURVE('',#5316,#5313,#2966,.T.);
#7445=ORIENTED_EDGE('',*,*,#5825,.T.);
#7446=ORIENTED_EDGE('',*,*,#5826,.T.);
#7447=ORIENTED_EDGE('',*,*,#5827,.F.);
#7448=ORIENTED_EDGE('',*,*,#5826,.F.);
#7449=ORIENTED_EDGE('',*,*,#5828,.T.);
#7450=ORIENTED_EDGE('',*,*,#5829,.T.);
#7451=ORIENTED_EDGE('',*,*,#5830,.T.);
#7452=ORIENTED_EDGE('',*,*,#5829,.F.);
#7453=ORIENTED_EDGE('',*,*,#5831,.F.);
#7454=ORIENTED_EDGE('',*,*,#5832,.T.);
#7455=ORIENTED_EDGE('',*,*,#5833,.T.);
#7456=ORIENTED_EDGE('',*,*,#5832,.F.);
#7457=ORIENTED_EDGE('',*,*,#5834,.F.);
#7458=ORIENTED_EDGE('',*,*,#5835,.T.);
#7459=ORIENTED_EDGE('',*,*,#5836,.T.);
#7460=ORIENTED_EDGE('',*,*,#5835,.F.);
#7461=ORIENTED_EDGE('',*,*,#5837,.F.);
#7462=ORIENTED_EDGE('',*,*,#5838,.T.);
#7463=ORIENTED_EDGE('',*,*,#5839,.T.);
#7464=ORIENTED_EDGE('',*,*,#5838,.F.);
#7465=ORIENTED_EDGE('',*,*,#5840,.F.);
#7466=ORIENTED_EDGE('',*,*,#5841,.T.);
#7467=ORIENTED_EDGE('',*,*,#5842,.T.);
#7468=ORIENTED_EDGE('',*,*,#5841,.F.);
#7469=ORIENTED_EDGE('',*,*,#5843,.F.);
#7470=ORIENTED_EDGE('',*,*,#5844,.T.);
#7471=ORIENTED_EDGE('',*,*,#5845,.T.);
#7472=ORIENTED_EDGE('',*,*,#5844,.F.);
#7473=ORIENTED_EDGE('',*,*,#5846,.F.);
#7474=ORIENTED_EDGE('',*,*,#5847,.T.);
#7475=ORIENTED_EDGE('',*,*,#5848,.T.);
#7476=ORIENTED_EDGE('',*,*,#5847,.F.);
#7477=ORIENTED_EDGE('',*,*,#5849,.F.);
#7478=ORIENTED_EDGE('',*,*,#5850,.T.);
#7479=ORIENTED_EDGE('',*,*,#5851,.F.);
#7480=ORIENTED_EDGE('',*,*,#5850,.F.);
#7481=ORIENTED_EDGE('',*,*,#5852,.F.);
#7482=ORIENTED_EDGE('',*,*,#5853,.T.);
#7483=ORIENTED_EDGE('',*,*,#5854,.F.);
#7484=ORIENTED_EDGE('',*,*,#5853,.F.);
#7485=ORIENTED_EDGE('',*,*,#5855,.F.);
#7486=ORIENTED_EDGE('',*,*,#5856,.T.);
#7487=ORIENTED_EDGE('',*,*,#5857,.F.);
#7488=ORIENTED_EDGE('',*,*,#5856,.F.);
#7489=ORIENTED_EDGE('',*,*,#5858,.F.);
#7490=ORIENTED_EDGE('',*,*,#5859,.T.);
#7491=ORIENTED_EDGE('',*,*,#5860,.F.);
#7492=ORIENTED_EDGE('',*,*,#5859,.F.);
#7493=ORIENTED_EDGE('',*,*,#5861,.F.);
#7494=ORIENTED_EDGE('',*,*,#5862,.T.);
#7495=ORIENTED_EDGE('',*,*,#5863,.F.);
#7496=ORIENTED_EDGE('',*,*,#5862,.F.);
#7497=ORIENTED_EDGE('',*,*,#5864,.F.);
#7498=ORIENTED_EDGE('',*,*,#5865,.T.);
#7499=ORIENTED_EDGE('',*,*,#5866,.F.);
#7500=ORIENTED_EDGE('',*,*,#5865,.F.);
#7501=ORIENTED_EDGE('',*,*,#5867,.T.);
#7502=ORIENTED_EDGE('',*,*,#5868,.T.);
#7503=ORIENTED_EDGE('',*,*,#5869,.T.);
#7504=ORIENTED_EDGE('',*,*,#5868,.F.);
#7505=ORIENTED_EDGE('',*,*,#5870,.T.);
#7506=ORIENTED_EDGE('',*,*,#5871,.T.);
#7507=ORIENTED_EDGE('',*,*,#5872,.F.);
#7508=ORIENTED_EDGE('',*,*,#5871,.F.);
#7509=ORIENTED_EDGE('',*,*,#5873,.T.);
#7510=ORIENTED_EDGE('',*,*,#5874,.T.);
#7511=ORIENTED_EDGE('',*,*,#5875,.T.);
#7512=ORIENTED_EDGE('',*,*,#5874,.F.);
#7513=ORIENTED_EDGE('',*,*,#5876,.T.);
#7514=ORIENTED_EDGE('',*,*,#5877,.T.);
#7515=ORIENTED_EDGE('',*,*,#5878,.T.);
#7516=ORIENTED_EDGE('',*,*,#5877,.F.);
#7517=ORIENTED_EDGE('',*,*,#5879,.T.);
#7518=ORIENTED_EDGE('',*,*,#5880,.T.);
#7519=ORIENTED_EDGE('',*,*,#5881,.T.);
#7520=ORIENTED_EDGE('',*,*,#5880,.F.);
#7521=ORIENTED_EDGE('',*,*,#5882,.T.);
#7522=ORIENTED_EDGE('',*,*,#5883,.T.);
#7523=ORIENTED_EDGE('',*,*,#5884,.T.);
#7524=ORIENTED_EDGE('',*,*,#5883,.F.);
#7525=ORIENTED_EDGE('',*,*,#5885,.T.);
#7526=ORIENTED_EDGE('',*,*,#5886,.T.);
#7527=ORIENTED_EDGE('',*,*,#5887,.F.);
#7528=ORIENTED_EDGE('',*,*,#5886,.F.);
#7529=ORIENTED_EDGE('',*,*,#5888,.T.);
#7530=ORIENTED_EDGE('',*,*,#5889,.T.);
#7531=ORIENTED_EDGE('',*,*,#5890,.F.);
#7532=ORIENTED_EDGE('',*,*,#5889,.F.);
#7533=ORIENTED_EDGE('',*,*,#5891,.T.);
#7534=ORIENTED_EDGE('',*,*,#5892,.T.);
#7535=ORIENTED_EDGE('',*,*,#5893,.T.);
#7536=ORIENTED_EDGE('',*,*,#5894,.T.);
#7537=ORIENTED_EDGE('',*,*,#5827,.T.);
#7538=ORIENTED_EDGE('',*,*,#5895,.T.);
#7539=ORIENTED_EDGE('',*,*,#5896,.T.);
#7540=ORIENTED_EDGE('',*,*,#5897,.T.);
#7541=ORIENTED_EDGE('',*,*,#5892,.F.);
#7542=ORIENTED_EDGE('',*,*,#5898,.T.);
#7543=ORIENTED_EDGE('',*,*,#5899,.T.);
#7544=ORIENTED_EDGE('',*,*,#5891,.F.);
#7545=ORIENTED_EDGE('',*,*,#5900,.T.);
#7546=ORIENTED_EDGE('',*,*,#5901,.T.);
#7547=ORIENTED_EDGE('',*,*,#5902,.T.);
#7548=ORIENTED_EDGE('',*,*,#5894,.F.);
#7549=ORIENTED_EDGE('',*,*,#5903,.T.);
#7550=ORIENTED_EDGE('',*,*,#5893,.F.);
#7551=ORIENTED_EDGE('',*,*,#5904,.T.);
#7552=ORIENTED_EDGE('',*,*,#5905,.T.);
#7553=ORIENTED_EDGE('',*,*,#5906,.T.);
#7554=ORIENTED_EDGE('',*,*,#5828,.F.);
#7555=ORIENTED_EDGE('',*,*,#5825,.F.);
#7556=ORIENTED_EDGE('',*,*,#5907,.F.);
#7557=ORIENTED_EDGE('',*,*,#5908,.F.);
#7558=ORIENTED_EDGE('',*,*,#5909,.T.);
#7559=ORIENTED_EDGE('',*,*,#5910,.T.);
#7560=ORIENTED_EDGE('',*,*,#5911,.T.);
#7561=ORIENTED_EDGE('',*,*,#5912,.F.);
#7562=ORIENTED_EDGE('',*,*,#5913,.T.);
#7563=ORIENTED_EDGE('',*,*,#5914,.T.);
#7564=ORIENTED_EDGE('',*,*,#5915,.T.);
#7565=ORIENTED_EDGE('',*,*,#5916,.T.);
#7566=ORIENTED_EDGE('',*,*,#5917,.T.);
#7567=ORIENTED_EDGE('',*,*,#5918,.F.);
#7568=ORIENTED_EDGE('',*,*,#5919,.T.);
#7569=ORIENTED_EDGE('',*,*,#5920,.T.);
#7570=ORIENTED_EDGE('',*,*,#5921,.T.);
#7571=ORIENTED_EDGE('',*,*,#5922,.F.);
#7572=ORIENTED_EDGE('',*,*,#5923,.F.);
#7573=ORIENTED_EDGE('',*,*,#5896,.F.);
#7574=ORIENTED_EDGE('',*,*,#5924,.T.);
#7575=ORIENTED_EDGE('',*,*,#5925,.T.);
#7576=ORIENTED_EDGE('',*,*,#5895,.F.);
#7577=ORIENTED_EDGE('',*,*,#5899,.F.);
#7578=ORIENTED_EDGE('',*,*,#5926,.T.);
#7579=ORIENTED_EDGE('',*,*,#5904,.F.);
#7580=ORIENTED_EDGE('',*,*,#5897,.F.);
#7581=ORIENTED_EDGE('',*,*,#5927,.T.);
#7582=ORIENTED_EDGE('',*,*,#5928,.T.);
#7583=ORIENTED_EDGE('',*,*,#5929,.T.);
#7584=ORIENTED_EDGE('',*,*,#5930,.T.);
#7585=ORIENTED_EDGE('',*,*,#5924,.F.);
#7586=ORIENTED_EDGE('',*,*,#5898,.F.);
#7587=ORIENTED_EDGE('',*,*,#5931,.F.);
#7588=ORIENTED_EDGE('',*,*,#5900,.F.);
#7589=ORIENTED_EDGE('',*,*,#5902,.F.);
#7590=ORIENTED_EDGE('',*,*,#5932,.T.);
#7591=ORIENTED_EDGE('',*,*,#5933,.T.);
#7592=ORIENTED_EDGE('',*,*,#5934,.T.);
#7593=ORIENTED_EDGE('',*,*,#5901,.F.);
#7594=ORIENTED_EDGE('',*,*,#5935,.F.);
#7595=ORIENTED_EDGE('',*,*,#5936,.T.);
#7596=ORIENTED_EDGE('',*,*,#5937,.T.);
#7597=ORIENTED_EDGE('',*,*,#5903,.F.);
#7598=ORIENTED_EDGE('',*,*,#5906,.F.);
#7599=ORIENTED_EDGE('',*,*,#5938,.T.);
#7600=ORIENTED_EDGE('',*,*,#5905,.F.);
#7601=ORIENTED_EDGE('',*,*,#5926,.F.);
#7602=ORIENTED_EDGE('',*,*,#5939,.T.);
#7603=ORIENTED_EDGE('',*,*,#5940,.T.);
#7604=ORIENTED_EDGE('',*,*,#5941,.T.);
#7605=ORIENTED_EDGE('',*,*,#5942,.T.);
#7606=ORIENTED_EDGE('',*,*,#5943,.T.);
#7607=ORIENTED_EDGE('',*,*,#5944,.T.);
#7608=ORIENTED_EDGE('',*,*,#5921,.F.);
#7609=ORIENTED_EDGE('',*,*,#5945,.T.);
#7610=ORIENTED_EDGE('',*,*,#5946,.T.);
#7611=ORIENTED_EDGE('',*,*,#5947,.T.);
#7612=ORIENTED_EDGE('',*,*,#5919,.F.);
#7613=ORIENTED_EDGE('',*,*,#5948,.T.);
#7614=ORIENTED_EDGE('',*,*,#5949,.T.);
#7615=ORIENTED_EDGE('',*,*,#5950,.T.);
#7616=ORIENTED_EDGE('',*,*,#5917,.F.);
#7617=ORIENTED_EDGE('',*,*,#5951,.T.);
#7618=ORIENTED_EDGE('',*,*,#5952,.F.);
#7619=ORIENTED_EDGE('',*,*,#5953,.F.);
#7620=ORIENTED_EDGE('',*,*,#5954,.F.);
#7621=ORIENTED_EDGE('',*,*,#5955,.F.);
#7622=ORIENTED_EDGE('',*,*,#5956,.F.);
#7623=ORIENTED_EDGE('',*,*,#5957,.F.);
#7624=ORIENTED_EDGE('',*,*,#5958,.F.);
#7625=ORIENTED_EDGE('',*,*,#5959,.F.);
#7626=ORIENTED_EDGE('',*,*,#5960,.F.);
#7627=ORIENTED_EDGE('',*,*,#5961,.F.);
#7628=ORIENTED_EDGE('',*,*,#5962,.F.);
#7629=ORIENTED_EDGE('',*,*,#5951,.F.);
#7630=ORIENTED_EDGE('',*,*,#5916,.F.);
#7631=ORIENTED_EDGE('',*,*,#5963,.F.);
#7632=ORIENTED_EDGE('',*,*,#5964,.F.);
#7633=ORIENTED_EDGE('',*,*,#5965,.F.);
#7634=ORIENTED_EDGE('',*,*,#5966,.F.);
#7635=ORIENTED_EDGE('',*,*,#5967,.F.);
#7636=ORIENTED_EDGE('',*,*,#5968,.F.);
#7637=ORIENTED_EDGE('',*,*,#5969,.F.);
#7638=ORIENTED_EDGE('',*,*,#5970,.F.);
#7639=ORIENTED_EDGE('',*,*,#5971,.F.);
#7640=ORIENTED_EDGE('',*,*,#5972,.F.);
#7641=ORIENTED_EDGE('',*,*,#5973,.F.);
#7642=ORIENTED_EDGE('',*,*,#5974,.F.);
#7643=ORIENTED_EDGE('',*,*,#5975,.F.);
#7644=ORIENTED_EDGE('',*,*,#5976,.F.);
#7645=ORIENTED_EDGE('',*,*,#5977,.F.);
#7646=ORIENTED_EDGE('',*,*,#5978,.F.);
#7647=ORIENTED_EDGE('',*,*,#5979,.F.);
#7648=ORIENTED_EDGE('',*,*,#5980,.F.);
#7649=ORIENTED_EDGE('',*,*,#5981,.F.);
#7650=ORIENTED_EDGE('',*,*,#5982,.F.);
#7651=ORIENTED_EDGE('',*,*,#5983,.F.);
#7652=ORIENTED_EDGE('',*,*,#5984,.F.);
#7653=ORIENTED_EDGE('',*,*,#5985,.F.);
#7654=ORIENTED_EDGE('',*,*,#5914,.F.);
#7655=ORIENTED_EDGE('',*,*,#5986,.F.);
#7656=ORIENTED_EDGE('',*,*,#5987,.F.);
#7657=ORIENTED_EDGE('',*,*,#5988,.F.);
#7658=ORIENTED_EDGE('',*,*,#5833,.F.);
#7659=ORIENTED_EDGE('',*,*,#5836,.F.);
#7660=ORIENTED_EDGE('',*,*,#5839,.F.);
#7661=ORIENTED_EDGE('',*,*,#5842,.F.);
#7662=ORIENTED_EDGE('',*,*,#5845,.F.);
#7663=ORIENTED_EDGE('',*,*,#5848,.F.);
#7664=ORIENTED_EDGE('',*,*,#5989,.T.);
#7665=ORIENTED_EDGE('',*,*,#5915,.F.);
#7666=ORIENTED_EDGE('',*,*,#5990,.T.);
#7667=ORIENTED_EDGE('',*,*,#5991,.T.);
#7668=ORIENTED_EDGE('',*,*,#5913,.F.);
#7669=ORIENTED_EDGE('',*,*,#5992,.T.);
#7670=ORIENTED_EDGE('',*,*,#5993,.T.);
#7671=ORIENTED_EDGE('',*,*,#5986,.T.);
#7672=ORIENTED_EDGE('',*,*,#5911,.F.);
#7673=ORIENTED_EDGE('',*,*,#5994,.T.);
#7674=ORIENTED_EDGE('',*,*,#5995,.T.);
#7675=ORIENTED_EDGE('',*,*,#5996,.T.);
#7676=ORIENTED_EDGE('',*,*,#5909,.F.);
#7677=ORIENTED_EDGE('',*,*,#5997,.T.);
#7678=ORIENTED_EDGE('',*,*,#5998,.T.);
#7679=ORIENTED_EDGE('',*,*,#5999,.T.);
#7680=ORIENTED_EDGE('',*,*,#5907,.T.);
#7681=ORIENTED_EDGE('',*,*,#5925,.F.);
#7682=ORIENTED_EDGE('',*,*,#5930,.F.);
#7683=ORIENTED_EDGE('',*,*,#6000,.T.);
#7684=ORIENTED_EDGE('',*,*,#5939,.F.);
#7685=ORIENTED_EDGE('',*,*,#5927,.F.);
#7686=ORIENTED_EDGE('',*,*,#5923,.T.);
#7687=ORIENTED_EDGE('',*,*,#6001,.T.);
#7688=ORIENTED_EDGE('',*,*,#6002,.T.);
#7689=ORIENTED_EDGE('',*,*,#6003,.T.);
#7690=ORIENTED_EDGE('',*,*,#6004,.T.);
#7691=ORIENTED_EDGE('',*,*,#6005,.T.);
#7692=ORIENTED_EDGE('',*,*,#5997,.F.);
#7693=ORIENTED_EDGE('',*,*,#5908,.T.);
#7694=ORIENTED_EDGE('',*,*,#6000,.F.);
#7695=ORIENTED_EDGE('',*,*,#5929,.F.);
#7696=ORIENTED_EDGE('',*,*,#6006,.T.);
#7697=ORIENTED_EDGE('',*,*,#5937,.F.);
#7698=ORIENTED_EDGE('',*,*,#6007,.T.);
#7699=ORIENTED_EDGE('',*,*,#5940,.F.);
#7700=ORIENTED_EDGE('',*,*,#6001,.F.);
#7701=ORIENTED_EDGE('',*,*,#5922,.T.);
#7702=ORIENTED_EDGE('',*,*,#5944,.F.);
#7703=ORIENTED_EDGE('',*,*,#6008,.T.);
#7704=ORIENTED_EDGE('',*,*,#6009,.T.);
#7705=ORIENTED_EDGE('',*,*,#6010,.T.);
#7706=ORIENTED_EDGE('',*,*,#6011,.T.);
#7707=ORIENTED_EDGE('',*,*,#6012,.T.);
#7708=ORIENTED_EDGE('',*,*,#6013,.T.);
#7709=ORIENTED_EDGE('',*,*,#6014,.T.);
#7710=ORIENTED_EDGE('',*,*,#6015,.T.);
#7711=ORIENTED_EDGE('',*,*,#6016,.T.);
#7712=ORIENTED_EDGE('',*,*,#5849,.T.);
#7713=ORIENTED_EDGE('',*,*,#5852,.T.);
#7714=ORIENTED_EDGE('',*,*,#5855,.T.);
#7715=ORIENTED_EDGE('',*,*,#5858,.T.);
#7716=ORIENTED_EDGE('',*,*,#5861,.T.);
#7717=ORIENTED_EDGE('',*,*,#5864,.T.);
#7718=ORIENTED_EDGE('',*,*,#6006,.F.);
#7719=ORIENTED_EDGE('',*,*,#5928,.F.);
#7720=ORIENTED_EDGE('',*,*,#6017,.T.);
#7721=ORIENTED_EDGE('',*,*,#5933,.F.);
#7722=ORIENTED_EDGE('',*,*,#5934,.F.);
#7723=ORIENTED_EDGE('',*,*,#6017,.F.);
#7724=ORIENTED_EDGE('',*,*,#5931,.T.);
#7725=ORIENTED_EDGE('',*,*,#5932,.F.);
#7726=ORIENTED_EDGE('',*,*,#6007,.F.);
#7727=ORIENTED_EDGE('',*,*,#5936,.F.);
#7728=ORIENTED_EDGE('',*,*,#6018,.T.);
#7729=ORIENTED_EDGE('',*,*,#5941,.F.);
#7730=ORIENTED_EDGE('',*,*,#5942,.F.);
#7731=ORIENTED_EDGE('',*,*,#6018,.F.);
#7732=ORIENTED_EDGE('',*,*,#5935,.T.);
#7733=ORIENTED_EDGE('',*,*,#5938,.F.);
#7734=ORIENTED_EDGE('',*,*,#5830,.F.);
#7735=ORIENTED_EDGE('',*,*,#5867,.F.);
#7736=ORIENTED_EDGE('',*,*,#6019,.T.);
#7737=ORIENTED_EDGE('',*,*,#6020,.F.);
#7738=ORIENTED_EDGE('',*,*,#6021,.T.);
#7739=ORIENTED_EDGE('',*,*,#6008,.F.);
#7740=ORIENTED_EDGE('',*,*,#5943,.F.);
#7741=ORIENTED_EDGE('',*,*,#6022,.T.);
#7742=ORIENTED_EDGE('',*,*,#6023,.T.);
#7743=ORIENTED_EDGE('',*,*,#6024,.T.);
#7744=ORIENTED_EDGE('',*,*,#5920,.F.);
#7745=ORIENTED_EDGE('',*,*,#5947,.F.);
#7746=ORIENTED_EDGE('',*,*,#6025,.F.);
#7747=ORIENTED_EDGE('',*,*,#6026,.F.);
#7748=ORIENTED_EDGE('',*,*,#6022,.F.);
#7749=ORIENTED_EDGE('',*,*,#5945,.F.);
#7750=ORIENTED_EDGE('',*,*,#6027,.T.);
#7751=ORIENTED_EDGE('',*,*,#6028,.T.);
#7752=ORIENTED_EDGE('',*,*,#6029,.T.);
#7753=ORIENTED_EDGE('',*,*,#6030,.T.);
#7754=ORIENTED_EDGE('',*,*,#6031,.T.);
#7755=ORIENTED_EDGE('',*,*,#6032,.T.);
#7756=ORIENTED_EDGE('',*,*,#6033,.T.);
#7757=ORIENTED_EDGE('',*,*,#6034,.T.);
#7758=ORIENTED_EDGE('',*,*,#6035,.T.);
#7759=ORIENTED_EDGE('',*,*,#6036,.T.);
#7760=ORIENTED_EDGE('',*,*,#6037,.T.);
#7761=ORIENTED_EDGE('',*,*,#6038,.T.);
#7762=ORIENTED_EDGE('',*,*,#6039,.T.);
#7763=ORIENTED_EDGE('',*,*,#6040,.T.);
#7764=ORIENTED_EDGE('',*,*,#6041,.T.);
#7765=ORIENTED_EDGE('',*,*,#6025,.T.);
#7766=ORIENTED_EDGE('',*,*,#5946,.F.);
#7767=ORIENTED_EDGE('',*,*,#6042,.T.);
#7768=ORIENTED_EDGE('',*,*,#6043,.T.);
#7769=ORIENTED_EDGE('',*,*,#6044,.T.);
#7770=ORIENTED_EDGE('',*,*,#6045,.T.);
#7771=ORIENTED_EDGE('',*,*,#6046,.T.);
#7772=ORIENTED_EDGE('',*,*,#6047,.T.);
#7773=ORIENTED_EDGE('',*,*,#6048,.T.);
#7774=ORIENTED_EDGE('',*,*,#6049,.T.);
#7775=ORIENTED_EDGE('',*,*,#6050,.T.);
#7776=ORIENTED_EDGE('',*,*,#6051,.T.);
#7777=ORIENTED_EDGE('',*,*,#6052,.T.);
#7778=ORIENTED_EDGE('',*,*,#6053,.T.);
#7779=ORIENTED_EDGE('',*,*,#6054,.T.);
#7780=ORIENTED_EDGE('',*,*,#6055,.T.);
#7781=ORIENTED_EDGE('',*,*,#6056,.T.);
#7782=ORIENTED_EDGE('',*,*,#6057,.T.);
#7783=ORIENTED_EDGE('',*,*,#6058,.T.);
#7784=ORIENTED_EDGE('',*,*,#6059,.T.);
#7785=ORIENTED_EDGE('',*,*,#6060,.T.);
#7786=ORIENTED_EDGE('',*,*,#6061,.T.);
#7787=ORIENTED_EDGE('',*,*,#6062,.T.);
#7788=ORIENTED_EDGE('',*,*,#6063,.T.);
#7789=ORIENTED_EDGE('',*,*,#6064,.T.);
#7790=ORIENTED_EDGE('',*,*,#5948,.F.);
#7791=ORIENTED_EDGE('',*,*,#5918,.T.);
#7792=ORIENTED_EDGE('',*,*,#5950,.F.);
#7793=ORIENTED_EDGE('',*,*,#6065,.T.);
#7794=ORIENTED_EDGE('',*,*,#6066,.T.);
#7795=ORIENTED_EDGE('',*,*,#6042,.F.);
#7796=ORIENTED_EDGE('',*,*,#6067,.T.);
#7797=ORIENTED_EDGE('',*,*,#6068,.F.);
#7798=ORIENTED_EDGE('',*,*,#6069,.F.);
#7799=ORIENTED_EDGE('',*,*,#6070,.F.);
#7800=ORIENTED_EDGE('',*,*,#6065,.F.);
#7801=ORIENTED_EDGE('',*,*,#5949,.F.);
#7802=ORIENTED_EDGE('',*,*,#5962,.T.);
#7803=ORIENTED_EDGE('',*,*,#6071,.F.);
#7804=ORIENTED_EDGE('',*,*,#6072,.T.);
#7805=ORIENTED_EDGE('',*,*,#6073,.T.);
#7806=ORIENTED_EDGE('',*,*,#6074,.T.);
#7807=ORIENTED_EDGE('',*,*,#5988,.T.);
#7808=ORIENTED_EDGE('',*,*,#6075,.F.);
#7809=ORIENTED_EDGE('',*,*,#6076,.F.);
#7810=ORIENTED_EDGE('',*,*,#6077,.F.);
#7811=ORIENTED_EDGE('',*,*,#6078,.F.);
#7812=ORIENTED_EDGE('',*,*,#6079,.F.);
#7813=ORIENTED_EDGE('',*,*,#6080,.F.);
#7814=ORIENTED_EDGE('',*,*,#6081,.F.);
#7815=ORIENTED_EDGE('',*,*,#6082,.F.);
#7816=ORIENTED_EDGE('',*,*,#6083,.F.);
#7817=ORIENTED_EDGE('',*,*,#6084,.F.);
#7818=ORIENTED_EDGE('',*,*,#6085,.F.);
#7819=ORIENTED_EDGE('',*,*,#6086,.F.);
#7820=ORIENTED_EDGE('',*,*,#6087,.F.);
#7821=ORIENTED_EDGE('',*,*,#6088,.F.);
#7822=ORIENTED_EDGE('',*,*,#5952,.T.);
#7823=ORIENTED_EDGE('',*,*,#6074,.F.);
#7824=ORIENTED_EDGE('',*,*,#6088,.T.);
#7825=ORIENTED_EDGE('',*,*,#6089,.T.);
#7826=ORIENTED_EDGE('',*,*,#6090,.T.);
#7827=ORIENTED_EDGE('',*,*,#5953,.T.);
#7828=ORIENTED_EDGE('',*,*,#6091,.F.);
#7829=ORIENTED_EDGE('',*,*,#6092,.F.);
#7830=ORIENTED_EDGE('',*,*,#5954,.T.);
#7831=ORIENTED_EDGE('',*,*,#6090,.F.);
#7832=ORIENTED_EDGE('',*,*,#6093,.T.);
#7833=ORIENTED_EDGE('',*,*,#6094,.T.);
#7834=ORIENTED_EDGE('',*,*,#6095,.T.);
#7835=ORIENTED_EDGE('',*,*,#5955,.T.);
#7836=ORIENTED_EDGE('',*,*,#6092,.T.);
#7837=ORIENTED_EDGE('',*,*,#6096,.T.);
#7838=ORIENTED_EDGE('',*,*,#6097,.F.);
#7839=ORIENTED_EDGE('',*,*,#6098,.F.);
#7840=ORIENTED_EDGE('',*,*,#6099,.F.);
#7841=ORIENTED_EDGE('',*,*,#6100,.F.);
#7842=ORIENTED_EDGE('',*,*,#6101,.F.);
#7843=ORIENTED_EDGE('',*,*,#6102,.F.);
#7844=ORIENTED_EDGE('',*,*,#6103,.F.);
#7845=ORIENTED_EDGE('',*,*,#6104,.F.);
#7846=ORIENTED_EDGE('',*,*,#6105,.F.);
#7847=ORIENTED_EDGE('',*,*,#6106,.F.);
#7848=ORIENTED_EDGE('',*,*,#5956,.T.);
#7849=ORIENTED_EDGE('',*,*,#6095,.F.);
#7850=ORIENTED_EDGE('',*,*,#6107,.T.);
#7851=ORIENTED_EDGE('',*,*,#6108,.T.);
#7852=ORIENTED_EDGE('',*,*,#6109,.T.);
#7853=ORIENTED_EDGE('',*,*,#5957,.T.);
#7854=ORIENTED_EDGE('',*,*,#6106,.T.);
#7855=ORIENTED_EDGE('',*,*,#6110,.T.);
#7856=ORIENTED_EDGE('',*,*,#6111,.F.);
#7857=ORIENTED_EDGE('',*,*,#6112,.F.);
#7858=ORIENTED_EDGE('',*,*,#5958,.T.);
#7859=ORIENTED_EDGE('',*,*,#6109,.F.);
#7860=ORIENTED_EDGE('',*,*,#6112,.T.);
#7861=ORIENTED_EDGE('',*,*,#6113,.T.);
#7862=ORIENTED_EDGE('',*,*,#6114,.T.);
#7863=ORIENTED_EDGE('',*,*,#5959,.T.);
#7864=ORIENTED_EDGE('',*,*,#6115,.F.);
#7865=ORIENTED_EDGE('',*,*,#6116,.F.);
#7866=ORIENTED_EDGE('',*,*,#6117,.F.);
#7867=ORIENTED_EDGE('',*,*,#6118,.F.);
#7868=ORIENTED_EDGE('',*,*,#6119,.F.);
#7869=ORIENTED_EDGE('',*,*,#6120,.F.);
#7870=ORIENTED_EDGE('',*,*,#6121,.F.);
#7871=ORIENTED_EDGE('',*,*,#6122,.F.);
#7872=ORIENTED_EDGE('',*,*,#6123,.F.);
#7873=ORIENTED_EDGE('',*,*,#6124,.F.);
#7874=ORIENTED_EDGE('',*,*,#6125,.F.);
#7875=ORIENTED_EDGE('',*,*,#6126,.F.);
#7876=ORIENTED_EDGE('',*,*,#6127,.F.);
#7877=ORIENTED_EDGE('',*,*,#6128,.F.);
#7878=ORIENTED_EDGE('',*,*,#5960,.T.);
#7879=ORIENTED_EDGE('',*,*,#6114,.F.);
#7880=ORIENTED_EDGE('',*,*,#6128,.T.);
#7881=ORIENTED_EDGE('',*,*,#6129,.T.);
#7882=ORIENTED_EDGE('',*,*,#6071,.T.);
#7883=ORIENTED_EDGE('',*,*,#5961,.T.);
#7884=ORIENTED_EDGE('',*,*,#5989,.F.);
#7885=ORIENTED_EDGE('',*,*,#6130,.T.);
#7886=ORIENTED_EDGE('',*,*,#6131,.T.);
#7887=ORIENTED_EDGE('',*,*,#5963,.T.);
#7888=ORIENTED_EDGE('',*,*,#6132,.F.);
#7889=ORIENTED_EDGE('',*,*,#6133,.F.);
#7890=ORIENTED_EDGE('',*,*,#5964,.T.);
#7891=ORIENTED_EDGE('',*,*,#6131,.F.);
#7892=ORIENTED_EDGE('',*,*,#6134,.F.);
#7893=ORIENTED_EDGE('',*,*,#5965,.T.);
#7894=ORIENTED_EDGE('',*,*,#6133,.T.);
#7895=ORIENTED_EDGE('',*,*,#6135,.F.);
#7896=ORIENTED_EDGE('',*,*,#6136,.F.);
#7897=ORIENTED_EDGE('',*,*,#6137,.F.);
#7898=ORIENTED_EDGE('',*,*,#5966,.T.);
#7899=ORIENTED_EDGE('',*,*,#6134,.T.);
#7900=ORIENTED_EDGE('',*,*,#6138,.F.);
#7901=ORIENTED_EDGE('',*,*,#5967,.T.);
#7902=ORIENTED_EDGE('',*,*,#6137,.T.);
#7903=ORIENTED_EDGE('',*,*,#6139,.F.);
#7904=ORIENTED_EDGE('',*,*,#6140,.T.);
#7905=ORIENTED_EDGE('',*,*,#6140,.F.);
#7906=ORIENTED_EDGE('',*,*,#6141,.F.);
#7907=ORIENTED_EDGE('',*,*,#6142,.T.);
#7908=ORIENTED_EDGE('',*,*,#6143,.F.);
#7909=ORIENTED_EDGE('',*,*,#6144,.T.);
#7910=ORIENTED_EDGE('',*,*,#5968,.T.);
#7911=ORIENTED_EDGE('',*,*,#5969,.T.);
#7912=ORIENTED_EDGE('',*,*,#6144,.F.);
#7913=ORIENTED_EDGE('',*,*,#6145,.F.);
#7914=ORIENTED_EDGE('',*,*,#6146,.T.);
#7915=ORIENTED_EDGE('',*,*,#6147,.F.);
#7916=ORIENTED_EDGE('',*,*,#5970,.T.);
#7917=ORIENTED_EDGE('',*,*,#6146,.F.);
#7918=ORIENTED_EDGE('',*,*,#6148,.F.);
#7919=ORIENTED_EDGE('',*,*,#6149,.F.);
#7920=ORIENTED_EDGE('',*,*,#6150,.F.);
#7921=ORIENTED_EDGE('',*,*,#5971,.T.);
#7922=ORIENTED_EDGE('',*,*,#6147,.T.);
#7923=ORIENTED_EDGE('',*,*,#6151,.F.);
#7924=ORIENTED_EDGE('',*,*,#6152,.F.);
#7925=ORIENTED_EDGE('',*,*,#6153,.F.);
#7926=ORIENTED_EDGE('',*,*,#5972,.T.);
#7927=ORIENTED_EDGE('',*,*,#6150,.T.);
#7928=ORIENTED_EDGE('',*,*,#6154,.F.);
#7929=ORIENTED_EDGE('',*,*,#5973,.T.);
#7930=ORIENTED_EDGE('',*,*,#6153,.T.);
#7931=ORIENTED_EDGE('',*,*,#6155,.F.);
#7932=ORIENTED_EDGE('',*,*,#6156,.T.);
#7933=ORIENTED_EDGE('',*,*,#6156,.F.);
#7934=ORIENTED_EDGE('',*,*,#6157,.F.);
#7935=ORIENTED_EDGE('',*,*,#6158,.T.);
#7936=ORIENTED_EDGE('',*,*,#6159,.F.);
#7937=ORIENTED_EDGE('',*,*,#6160,.T.);
#7938=ORIENTED_EDGE('',*,*,#5974,.T.);
#7939=ORIENTED_EDGE('',*,*,#5975,.T.);
#7940=ORIENTED_EDGE('',*,*,#6160,.F.);
#7941=ORIENTED_EDGE('',*,*,#6161,.F.);
#7942=ORIENTED_EDGE('',*,*,#6162,.T.);
#7943=ORIENTED_EDGE('',*,*,#6163,.F.);
#7944=ORIENTED_EDGE('',*,*,#5976,.T.);
#7945=ORIENTED_EDGE('',*,*,#6162,.F.);
#7946=ORIENTED_EDGE('',*,*,#6164,.F.);
#7947=ORIENTED_EDGE('',*,*,#6165,.F.);
#7948=ORIENTED_EDGE('',*,*,#6166,.F.);
#7949=ORIENTED_EDGE('',*,*,#5977,.T.);
#7950=ORIENTED_EDGE('',*,*,#6163,.T.);
#7951=ORIENTED_EDGE('',*,*,#6167,.F.);
#7952=ORIENTED_EDGE('',*,*,#6168,.F.);
#7953=ORIENTED_EDGE('',*,*,#6169,.F.);
#7954=ORIENTED_EDGE('',*,*,#5978,.T.);
#7955=ORIENTED_EDGE('',*,*,#6166,.T.);
#7956=ORIENTED_EDGE('',*,*,#6170,.F.);
#7957=ORIENTED_EDGE('',*,*,#5979,.T.);
#7958=ORIENTED_EDGE('',*,*,#6169,.T.);
#7959=ORIENTED_EDGE('',*,*,#6171,.F.);
#7960=ORIENTED_EDGE('',*,*,#6172,.T.);
#7961=ORIENTED_EDGE('',*,*,#6172,.F.);
#7962=ORIENTED_EDGE('',*,*,#6173,.F.);
#7963=ORIENTED_EDGE('',*,*,#6174,.T.);
#7964=ORIENTED_EDGE('',*,*,#6175,.F.);
#7965=ORIENTED_EDGE('',*,*,#6176,.T.);
#7966=ORIENTED_EDGE('',*,*,#5980,.T.);
#7967=ORIENTED_EDGE('',*,*,#5981,.T.);
#7968=ORIENTED_EDGE('',*,*,#6176,.F.);
#7969=ORIENTED_EDGE('',*,*,#6177,.F.);
#7970=ORIENTED_EDGE('',*,*,#6178,.T.);
#7971=ORIENTED_EDGE('',*,*,#6179,.F.);
#7972=ORIENTED_EDGE('',*,*,#5982,.T.);
#7973=ORIENTED_EDGE('',*,*,#6178,.F.);
#7974=ORIENTED_EDGE('',*,*,#6180,.F.);
#7975=ORIENTED_EDGE('',*,*,#6181,.F.);
#7976=ORIENTED_EDGE('',*,*,#6182,.F.);
#7977=ORIENTED_EDGE('',*,*,#5983,.T.);
#7978=ORIENTED_EDGE('',*,*,#6179,.T.);
#7979=ORIENTED_EDGE('',*,*,#6183,.F.);
#7980=ORIENTED_EDGE('',*,*,#5984,.T.);
#7981=ORIENTED_EDGE('',*,*,#6182,.T.);
#7982=ORIENTED_EDGE('',*,*,#6184,.F.);
#7983=ORIENTED_EDGE('',*,*,#6185,.F.);
#7984=ORIENTED_EDGE('',*,*,#6185,.T.);
#7985=ORIENTED_EDGE('',*,*,#6186,.T.);
#7986=ORIENTED_EDGE('',*,*,#5990,.F.);
#7987=ORIENTED_EDGE('',*,*,#5985,.T.);
#7988=ORIENTED_EDGE('',*,*,#5987,.T.);
#7989=ORIENTED_EDGE('',*,*,#5993,.F.);
#7990=ORIENTED_EDGE('',*,*,#6187,.F.);
#7991=ORIENTED_EDGE('',*,*,#6188,.F.);
#7992=ORIENTED_EDGE('',*,*,#6189,.F.);
#7993=ORIENTED_EDGE('',*,*,#6190,.F.);
#7994=ORIENTED_EDGE('',*,*,#6191,.F.);
#7995=ORIENTED_EDGE('',*,*,#6072,.F.);
#7996=ORIENTED_EDGE('',*,*,#6192,.F.);
#7997=ORIENTED_EDGE('',*,*,#6193,.F.);
#7998=ORIENTED_EDGE('',*,*,#6194,.F.);
#7999=ORIENTED_EDGE('',*,*,#6195,.F.);
#8000=ORIENTED_EDGE('',*,*,#6196,.F.);
#8001=ORIENTED_EDGE('',*,*,#6197,.F.);
#8002=ORIENTED_EDGE('',*,*,#6198,.F.);
#8003=ORIENTED_EDGE('',*,*,#6199,.F.);
#8004=ORIENTED_EDGE('',*,*,#6200,.F.);
#8005=ORIENTED_EDGE('',*,*,#6201,.F.);
#8006=ORIENTED_EDGE('',*,*,#6202,.F.);
#8007=ORIENTED_EDGE('',*,*,#6203,.F.);
#8008=ORIENTED_EDGE('',*,*,#6204,.F.);
#8009=ORIENTED_EDGE('',*,*,#6205,.F.);
#8010=ORIENTED_EDGE('',*,*,#5991,.F.);
#8011=ORIENTED_EDGE('',*,*,#6206,.F.);
#8012=ORIENTED_EDGE('',*,*,#5870,.F.);
#8013=ORIENTED_EDGE('',*,*,#6207,.T.);
#8014=ORIENTED_EDGE('',*,*,#6187,.T.);
#8015=ORIENTED_EDGE('',*,*,#5992,.F.);
#8016=ORIENTED_EDGE('',*,*,#5912,.T.);
#8017=ORIENTED_EDGE('',*,*,#5996,.F.);
#8018=ORIENTED_EDGE('',*,*,#6208,.T.);
#8019=ORIENTED_EDGE('',*,*,#6209,.F.);
#8020=ORIENTED_EDGE('',*,*,#6210,.F.);
#8021=ORIENTED_EDGE('',*,*,#6211,.F.);
#8022=ORIENTED_EDGE('',*,*,#5994,.F.);
#8023=ORIENTED_EDGE('',*,*,#5910,.F.);
#8024=ORIENTED_EDGE('',*,*,#5999,.F.);
#8025=ORIENTED_EDGE('',*,*,#6212,.T.);
#8026=ORIENTED_EDGE('',*,*,#6213,.T.);
#8027=ORIENTED_EDGE('',*,*,#6214,.T.);
#8028=ORIENTED_EDGE('',*,*,#6215,.T.);
#8029=ORIENTED_EDGE('',*,*,#6216,.T.);
#8030=ORIENTED_EDGE('',*,*,#6217,.T.);
#8031=ORIENTED_EDGE('',*,*,#6218,.T.);
#8032=ORIENTED_EDGE('',*,*,#6219,.T.);
#8033=ORIENTED_EDGE('',*,*,#6220,.T.);
#8034=ORIENTED_EDGE('',*,*,#6221,.T.);
#8035=ORIENTED_EDGE('',*,*,#6222,.T.);
#8036=ORIENTED_EDGE('',*,*,#6223,.T.);
#8037=ORIENTED_EDGE('',*,*,#6224,.T.);
#8038=ORIENTED_EDGE('',*,*,#6225,.T.);
#8039=ORIENTED_EDGE('',*,*,#6226,.T.);
#8040=ORIENTED_EDGE('',*,*,#6227,.T.);
#8041=ORIENTED_EDGE('',*,*,#6228,.T.);
#8042=ORIENTED_EDGE('',*,*,#6229,.T.);
#8043=ORIENTED_EDGE('',*,*,#6230,.T.);
#8044=ORIENTED_EDGE('',*,*,#6231,.T.);
#8045=ORIENTED_EDGE('',*,*,#6232,.T.);
#8046=ORIENTED_EDGE('',*,*,#6233,.T.);
#8047=ORIENTED_EDGE('',*,*,#6234,.T.);
#8048=ORIENTED_EDGE('',*,*,#6235,.T.);
#8049=ORIENTED_EDGE('',*,*,#6236,.T.);
#8050=ORIENTED_EDGE('',*,*,#6237,.T.);
#8051=ORIENTED_EDGE('',*,*,#6238,.T.);
#8052=ORIENTED_EDGE('',*,*,#6208,.F.);
#8053=ORIENTED_EDGE('',*,*,#5995,.F.);
#8054=ORIENTED_EDGE('',*,*,#6211,.T.);
#8055=ORIENTED_EDGE('',*,*,#6239,.T.);
#8056=ORIENTED_EDGE('',*,*,#6240,.T.);
#8057=ORIENTED_EDGE('',*,*,#6241,.T.);
#8058=ORIENTED_EDGE('',*,*,#6242,.T.);
#8059=ORIENTED_EDGE('',*,*,#6243,.T.);
#8060=ORIENTED_EDGE('',*,*,#6244,.T.);
#8061=ORIENTED_EDGE('',*,*,#6245,.T.);
#8062=ORIENTED_EDGE('',*,*,#6246,.T.);
#8063=ORIENTED_EDGE('',*,*,#6247,.T.);
#8064=ORIENTED_EDGE('',*,*,#6248,.T.);
#8065=ORIENTED_EDGE('',*,*,#5998,.F.);
#8066=ORIENTED_EDGE('',*,*,#6005,.F.);
#8067=ORIENTED_EDGE('',*,*,#6249,.T.);
#8068=ORIENTED_EDGE('',*,*,#6250,.F.);
#8069=ORIENTED_EDGE('',*,*,#6251,.T.);
#8070=ORIENTED_EDGE('',*,*,#6252,.T.);
#8071=ORIENTED_EDGE('',*,*,#6253,.T.);
#8072=ORIENTED_EDGE('',*,*,#6209,.T.);
#8073=ORIENTED_EDGE('',*,*,#6254,.T.);
#8074=ORIENTED_EDGE('',*,*,#6255,.T.);
#8075=ORIENTED_EDGE('',*,*,#6256,.T.);
#8076=ORIENTED_EDGE('',*,*,#6003,.F.);
#8077=ORIENTED_EDGE('',*,*,#6257,.T.);
#8078=ORIENTED_EDGE('',*,*,#6258,.T.);
#8079=ORIENTED_EDGE('',*,*,#6259,.T.);
#8080=ORIENTED_EDGE('',*,*,#6260,.T.);
#8081=ORIENTED_EDGE('',*,*,#6261,.T.);
#8082=ORIENTED_EDGE('',*,*,#6262,.T.);
#8083=ORIENTED_EDGE('',*,*,#6263,.T.);
#8084=ORIENTED_EDGE('',*,*,#6264,.T.);
#8085=ORIENTED_EDGE('',*,*,#6265,.T.);
#8086=ORIENTED_EDGE('',*,*,#6266,.T.);
#8087=ORIENTED_EDGE('',*,*,#6267,.T.);
#8088=ORIENTED_EDGE('',*,*,#6268,.T.);
#8089=ORIENTED_EDGE('',*,*,#6257,.F.);
#8090=ORIENTED_EDGE('',*,*,#6002,.F.);
#8091=ORIENTED_EDGE('',*,*,#6269,.T.);
#8092=ORIENTED_EDGE('',*,*,#6270,.T.);
#8093=ORIENTED_EDGE('',*,*,#6271,.T.);
#8094=ORIENTED_EDGE('',*,*,#6272,.T.);
#8095=ORIENTED_EDGE('',*,*,#6269,.F.);
#8096=ORIENTED_EDGE('',*,*,#6016,.F.);
#8097=ORIENTED_EDGE('',*,*,#6271,.F.);
#8098=ORIENTED_EDGE('',*,*,#6015,.F.);
#8099=ORIENTED_EDGE('',*,*,#6273,.T.);
#8100=ORIENTED_EDGE('',*,*,#6274,.T.);
#8101=ORIENTED_EDGE('',*,*,#6275,.T.);
#8102=ORIENTED_EDGE('',*,*,#6276,.T.);
#8103=ORIENTED_EDGE('',*,*,#6277,.T.);
#8104=ORIENTED_EDGE('',*,*,#6278,.T.);
#8105=ORIENTED_EDGE('',*,*,#6273,.F.);
#8106=ORIENTED_EDGE('',*,*,#6014,.F.);
#8107=ORIENTED_EDGE('',*,*,#6279,.T.);
#8108=ORIENTED_EDGE('',*,*,#6280,.T.);
#8109=ORIENTED_EDGE('',*,*,#6281,.T.);
#8110=ORIENTED_EDGE('',*,*,#6282,.T.);
#8111=ORIENTED_EDGE('',*,*,#6283,.T.);
#8112=ORIENTED_EDGE('',*,*,#6284,.T.);
#8113=ORIENTED_EDGE('',*,*,#6285,.T.);
#8114=ORIENTED_EDGE('',*,*,#6286,.T.);
#8115=ORIENTED_EDGE('',*,*,#6279,.F.);
#8116=ORIENTED_EDGE('',*,*,#6013,.F.);
#8117=ORIENTED_EDGE('',*,*,#6287,.T.);
#8118=ORIENTED_EDGE('',*,*,#6288,.T.);
#8119=ORIENTED_EDGE('',*,*,#6289,.T.);
#8120=ORIENTED_EDGE('',*,*,#6290,.T.);
#8121=ORIENTED_EDGE('',*,*,#6291,.T.);
#8122=ORIENTED_EDGE('',*,*,#6292,.T.);
#8123=ORIENTED_EDGE('',*,*,#6287,.F.);
#8124=ORIENTED_EDGE('',*,*,#6012,.F.);
#8125=ORIENTED_EDGE('',*,*,#6291,.F.);
#8126=ORIENTED_EDGE('',*,*,#6011,.F.);
#8127=ORIENTED_EDGE('',*,*,#6293,.T.);
#8128=ORIENTED_EDGE('',*,*,#6294,.T.);
#8129=ORIENTED_EDGE('',*,*,#6295,.T.);
#8130=ORIENTED_EDGE('',*,*,#6296,.T.);
#8131=ORIENTED_EDGE('',*,*,#6293,.F.);
#8132=ORIENTED_EDGE('',*,*,#6010,.F.);
#8133=ORIENTED_EDGE('',*,*,#6297,.T.);
#8134=ORIENTED_EDGE('',*,*,#6298,.T.);
#8135=ORIENTED_EDGE('',*,*,#6299,.T.);
#8136=ORIENTED_EDGE('',*,*,#6300,.T.);
#8137=ORIENTED_EDGE('',*,*,#6301,.T.);
#8138=ORIENTED_EDGE('',*,*,#6302,.T.);
#8139=ORIENTED_EDGE('',*,*,#6303,.T.);
#8140=ORIENTED_EDGE('',*,*,#6304,.T.);
#8141=ORIENTED_EDGE('',*,*,#6305,.T.);
#8142=ORIENTED_EDGE('',*,*,#6306,.T.);
#8143=ORIENTED_EDGE('',*,*,#6307,.T.);
#8144=ORIENTED_EDGE('',*,*,#6308,.T.);
#8145=ORIENTED_EDGE('',*,*,#6297,.F.);
#8146=ORIENTED_EDGE('',*,*,#6009,.F.);
#8147=ORIENTED_EDGE('',*,*,#6021,.F.);
#8148=ORIENTED_EDGE('',*,*,#6309,.T.);
#8149=ORIENTED_EDGE('',*,*,#6249,.F.);
#8150=ORIENTED_EDGE('',*,*,#6004,.F.);
#8151=ORIENTED_EDGE('',*,*,#6256,.F.);
#8152=ORIENTED_EDGE('',*,*,#6310,.T.);
#8153=ORIENTED_EDGE('',*,*,#6311,.F.);
#8154=ORIENTED_EDGE('',*,*,#6312,.F.);
#8155=ORIENTED_EDGE('',*,*,#6313,.F.);
#8156=ORIENTED_EDGE('',*,*,#6019,.F.);
#8157=ORIENTED_EDGE('',*,*,#6024,.F.);
#8158=ORIENTED_EDGE('',*,*,#6314,.F.);
#8159=ORIENTED_EDGE('',*,*,#6040,.F.);
#8160=ORIENTED_EDGE('',*,*,#6315,.F.);
#8161=ORIENTED_EDGE('',*,*,#6311,.T.);
#8162=ORIENTED_EDGE('',*,*,#6023,.F.);
#8163=ORIENTED_EDGE('',*,*,#6026,.T.);
#8164=ORIENTED_EDGE('',*,*,#6041,.F.);
#8165=ORIENTED_EDGE('',*,*,#6314,.T.);
#8166=ORIENTED_EDGE('',*,*,#6028,.F.);
#8167=ORIENTED_EDGE('',*,*,#6316,.T.);
#8168=ORIENTED_EDGE('',*,*,#6317,.T.);
#8169=ORIENTED_EDGE('',*,*,#6318,.T.);
#8170=ORIENTED_EDGE('',*,*,#6319,.F.);
#8171=ORIENTED_EDGE('',*,*,#6320,.F.);
#8172=ORIENTED_EDGE('',*,*,#6316,.F.);
#8173=ORIENTED_EDGE('',*,*,#6027,.F.);
#8174=ORIENTED_EDGE('',*,*,#6321,.F.);
#8175=ORIENTED_EDGE('',*,*,#6322,.F.);
#8176=ORIENTED_EDGE('',*,*,#6323,.T.);
#8177=ORIENTED_EDGE('',*,*,#6321,.T.);
#8178=ORIENTED_EDGE('',*,*,#6064,.F.);
#8179=ORIENTED_EDGE('',*,*,#6324,.T.);
#8180=ORIENTED_EDGE('',*,*,#6325,.T.);
#8181=ORIENTED_EDGE('',*,*,#6324,.F.);
#8182=ORIENTED_EDGE('',*,*,#6063,.F.);
#8183=ORIENTED_EDGE('',*,*,#6326,.T.);
#8184=ORIENTED_EDGE('',*,*,#6327,.T.);
#8185=ORIENTED_EDGE('',*,*,#6328,.T.);
#8186=ORIENTED_EDGE('',*,*,#6329,.F.);
#8187=ORIENTED_EDGE('',*,*,#6326,.F.);
#8188=ORIENTED_EDGE('',*,*,#6062,.F.);
#8189=ORIENTED_EDGE('',*,*,#6330,.F.);
#8190=ORIENTED_EDGE('',*,*,#6330,.T.);
#8191=ORIENTED_EDGE('',*,*,#6061,.F.);
#8192=ORIENTED_EDGE('',*,*,#6107,.F.);
#8193=ORIENTED_EDGE('',*,*,#6113,.F.);
#8194=ORIENTED_EDGE('',*,*,#6111,.T.);
#8195=ORIENTED_EDGE('',*,*,#6108,.F.);
#8196=ORIENTED_EDGE('',*,*,#6060,.F.);
#8197=ORIENTED_EDGE('',*,*,#6331,.T.);
#8198=ORIENTED_EDGE('',*,*,#6332,.T.);
#8199=ORIENTED_EDGE('',*,*,#6333,.T.);
#8200=ORIENTED_EDGE('',*,*,#6115,.T.);
#8201=ORIENTED_EDGE('',*,*,#6334,.T.);
#8202=ORIENTED_EDGE('',*,*,#6331,.F.);
#8203=ORIENTED_EDGE('',*,*,#6059,.F.);
#8204=ORIENTED_EDGE('',*,*,#6335,.T.);
#8205=ORIENTED_EDGE('',*,*,#6057,.F.);
#8206=ORIENTED_EDGE('',*,*,#6336,.F.);
#8207=ORIENTED_EDGE('',*,*,#6337,.F.);
#8208=ORIENTED_EDGE('',*,*,#6338,.F.);
#8209=ORIENTED_EDGE('',*,*,#6339,.F.);
#8210=ORIENTED_EDGE('',*,*,#6340,.F.);
#8211=ORIENTED_EDGE('',*,*,#6336,.T.);
#8212=ORIENTED_EDGE('',*,*,#6056,.F.);
#8213=ORIENTED_EDGE('',*,*,#6341,.F.);
#8214=ORIENTED_EDGE('',*,*,#6339,.T.);
#8215=ORIENTED_EDGE('',*,*,#6055,.F.);
#8216=ORIENTED_EDGE('',*,*,#6342,.F.);
#8217=ORIENTED_EDGE('',*,*,#6343,.T.);
#8218=ORIENTED_EDGE('',*,*,#6344,.T.);
#8219=ORIENTED_EDGE('',*,*,#6053,.F.);
#8220=ORIENTED_EDGE('',*,*,#6345,.T.);
#8221=ORIENTED_EDGE('',*,*,#6117,.T.);
#8222=ORIENTED_EDGE('',*,*,#6346,.T.);
#8223=ORIENTED_EDGE('',*,*,#6347,.T.);
#8224=ORIENTED_EDGE('',*,*,#6345,.F.);
#8225=ORIENTED_EDGE('',*,*,#6052,.F.);
#8226=ORIENTED_EDGE('',*,*,#6348,.T.);
#8227=ORIENTED_EDGE('',*,*,#6349,.T.);
#8228=ORIENTED_EDGE('',*,*,#6350,.F.);
#8229=ORIENTED_EDGE('',*,*,#6351,.T.);
#8230=ORIENTED_EDGE('',*,*,#6051,.F.);
#8231=ORIENTED_EDGE('',*,*,#6352,.T.);
#8232=ORIENTED_EDGE('',*,*,#6121,.T.);
#8233=ORIENTED_EDGE('',*,*,#6353,.T.);
#8234=ORIENTED_EDGE('',*,*,#6354,.T.);
#8235=ORIENTED_EDGE('',*,*,#6050,.F.);
#8236=ORIENTED_EDGE('',*,*,#6355,.F.);
#8237=ORIENTED_EDGE('',*,*,#6122,.T.);
#8238=ORIENTED_EDGE('',*,*,#6352,.F.);
#8239=ORIENTED_EDGE('',*,*,#6049,.F.);
#8240=ORIENTED_EDGE('',*,*,#6355,.T.);
#8241=ORIENTED_EDGE('',*,*,#6048,.F.);
#8242=ORIENTED_EDGE('',*,*,#6356,.T.);
#8243=ORIENTED_EDGE('',*,*,#6123,.T.);
#8244=ORIENTED_EDGE('',*,*,#6357,.F.);
#8245=ORIENTED_EDGE('',*,*,#6124,.T.);
#8246=ORIENTED_EDGE('',*,*,#6356,.F.);
#8247=ORIENTED_EDGE('',*,*,#6047,.F.);
#8248=ORIENTED_EDGE('',*,*,#6357,.T.);
#8249=ORIENTED_EDGE('',*,*,#6046,.F.);
#8250=ORIENTED_EDGE('',*,*,#6358,.T.);
#8251=ORIENTED_EDGE('',*,*,#6359,.T.);
#8252=ORIENTED_EDGE('',*,*,#6125,.T.);
#8253=ORIENTED_EDGE('',*,*,#6360,.F.);
#8254=ORIENTED_EDGE('',*,*,#6361,.T.);
#8255=ORIENTED_EDGE('',*,*,#6045,.F.);
#8256=ORIENTED_EDGE('',*,*,#6362,.T.);
#8257=ORIENTED_EDGE('',*,*,#6069,.T.);
#8258=ORIENTED_EDGE('',*,*,#6363,.T.);
#8259=ORIENTED_EDGE('',*,*,#6364,.T.);
#8260=ORIENTED_EDGE('',*,*,#6044,.F.);
#8261=ORIENTED_EDGE('',*,*,#6066,.F.);
#8262=ORIENTED_EDGE('',*,*,#6070,.T.);
#8263=ORIENTED_EDGE('',*,*,#6362,.F.);
#8264=ORIENTED_EDGE('',*,*,#6043,.F.);
#8265=ORIENTED_EDGE('',*,*,#6365,.T.);
#8266=ORIENTED_EDGE('',*,*,#6366,.F.);
#8267=ORIENTED_EDGE('',*,*,#6039,.F.);
#8268=ORIENTED_EDGE('',*,*,#6038,.F.);
#8269=ORIENTED_EDGE('',*,*,#6367,.F.);
#8270=ORIENTED_EDGE('',*,*,#6300,.F.);
#8271=ORIENTED_EDGE('',*,*,#6368,.F.);
#8272=ORIENTED_EDGE('',*,*,#6369,.F.);
#8273=ORIENTED_EDGE('',*,*,#6301,.F.);
#8274=ORIENTED_EDGE('',*,*,#6367,.T.);
#8275=ORIENTED_EDGE('',*,*,#6037,.F.);
#8276=ORIENTED_EDGE('',*,*,#6370,.T.);
#8277=ORIENTED_EDGE('',*,*,#6036,.F.);
#8278=ORIENTED_EDGE('',*,*,#6371,.F.);
#8279=ORIENTED_EDGE('',*,*,#6302,.F.);
#8280=ORIENTED_EDGE('',*,*,#6370,.F.);
#8281=ORIENTED_EDGE('',*,*,#6303,.F.);
#8282=ORIENTED_EDGE('',*,*,#6371,.T.);
#8283=ORIENTED_EDGE('',*,*,#6035,.F.);
#8284=ORIENTED_EDGE('',*,*,#6372,.T.);
#8285=ORIENTED_EDGE('',*,*,#6304,.F.);
#8286=ORIENTED_EDGE('',*,*,#6372,.F.);
#8287=ORIENTED_EDGE('',*,*,#6034,.F.);
#8288=ORIENTED_EDGE('',*,*,#6373,.F.);
#8289=ORIENTED_EDGE('',*,*,#6374,.F.);
#8290=ORIENTED_EDGE('',*,*,#6375,.T.);
#8291=ORIENTED_EDGE('',*,*,#6376,.F.);
#8292=ORIENTED_EDGE('',*,*,#6033,.F.);
#8293=ORIENTED_EDGE('',*,*,#6032,.F.);
#8294=ORIENTED_EDGE('',*,*,#6377,.F.);
#8295=ORIENTED_EDGE('',*,*,#6308,.F.);
#8296=ORIENTED_EDGE('',*,*,#6378,.F.);
#8297=ORIENTED_EDGE('',*,*,#6379,.F.);
#8298=ORIENTED_EDGE('',*,*,#6295,.F.);
#8299=ORIENTED_EDGE('',*,*,#6377,.T.);
#8300=ORIENTED_EDGE('',*,*,#6031,.F.);
#8301=ORIENTED_EDGE('',*,*,#6380,.T.);
#8302=ORIENTED_EDGE('',*,*,#6292,.F.);
#8303=ORIENTED_EDGE('',*,*,#6294,.F.);
#8304=ORIENTED_EDGE('',*,*,#6296,.F.);
#8305=ORIENTED_EDGE('',*,*,#6380,.F.);
#8306=ORIENTED_EDGE('',*,*,#6030,.F.);
#8307=ORIENTED_EDGE('',*,*,#6288,.F.);
#8308=ORIENTED_EDGE('',*,*,#6289,.F.);
#8309=ORIENTED_EDGE('',*,*,#6029,.F.);
#8310=ORIENTED_EDGE('',*,*,#6318,.F.);
#8311=ORIENTED_EDGE('',*,*,#6381,.T.);
#8312=ORIENTED_EDGE('',*,*,#6363,.F.);
#8313=ORIENTED_EDGE('',*,*,#6068,.T.);
#8314=ORIENTED_EDGE('',*,*,#6382,.T.);
#8315=ORIENTED_EDGE('',*,*,#6094,.F.);
#8316=ORIENTED_EDGE('',*,*,#6383,.F.);
#8317=ORIENTED_EDGE('',*,*,#6384,.F.);
#8318=ORIENTED_EDGE('',*,*,#6385,.F.);
#8319=ORIENTED_EDGE('',*,*,#6386,.F.);
#8320=ORIENTED_EDGE('',*,*,#6097,.T.);
#8321=ORIENTED_EDGE('',*,*,#5831,.T.);
#8322=ORIENTED_EDGE('',*,*,#6387,.F.);
#8323=ORIENTED_EDGE('',*,*,#6388,.F.);
#8324=ORIENTED_EDGE('',*,*,#6389,.F.);
#8325=ORIENTED_EDGE('',*,*,#6390,.F.);
#8326=ORIENTED_EDGE('',*,*,#6083,.T.);
#8327=ORIENTED_EDGE('',*,*,#5834,.T.);
#8328=ORIENTED_EDGE('',*,*,#6191,.T.);
#8329=ORIENTED_EDGE('',*,*,#6391,.F.);
#8330=ORIENTED_EDGE('',*,*,#6392,.F.);
#8331=ORIENTED_EDGE('',*,*,#6393,.F.);
#8332=ORIENTED_EDGE('',*,*,#6394,.F.);
#8333=ORIENTED_EDGE('',*,*,#6075,.T.);
#8334=ORIENTED_EDGE('',*,*,#6073,.F.);
#8335=ORIENTED_EDGE('',*,*,#5837,.T.);
#8336=ORIENTED_EDGE('',*,*,#6105,.T.);
#8337=ORIENTED_EDGE('',*,*,#6395,.F.);
#8338=ORIENTED_EDGE('',*,*,#6396,.F.);
#8339=ORIENTED_EDGE('',*,*,#6397,.F.);
#8340=ORIENTED_EDGE('',*,*,#6398,.F.);
#8341=ORIENTED_EDGE('',*,*,#6110,.F.);
#8342=ORIENTED_EDGE('',*,*,#5840,.T.);
#8343=ORIENTED_EDGE('',*,*,#6399,.F.);
#8344=ORIENTED_EDGE('',*,*,#6400,.F.);
#8345=ORIENTED_EDGE('',*,*,#6401,.F.);
#8346=ORIENTED_EDGE('',*,*,#6402,.F.);
#8347=ORIENTED_EDGE('',*,*,#6119,.T.);
#8348=ORIENTED_EDGE('',*,*,#5843,.T.);
#8349=ORIENTED_EDGE('',*,*,#6127,.T.);
#8350=ORIENTED_EDGE('',*,*,#6403,.F.);
#8351=ORIENTED_EDGE('',*,*,#6404,.F.);
#8352=ORIENTED_EDGE('',*,*,#6405,.F.);
#8353=ORIENTED_EDGE('',*,*,#6382,.F.);
#8354=ORIENTED_EDGE('',*,*,#6067,.F.);
#8355=ORIENTED_EDGE('',*,*,#6129,.F.);
#8356=ORIENTED_EDGE('',*,*,#5846,.T.);
#8357=ORIENTED_EDGE('',*,*,#6406,.T.);
#8358=ORIENTED_EDGE('',*,*,#6407,.T.);
#8359=ORIENTED_EDGE('',*,*,#6076,.T.);
#8360=ORIENTED_EDGE('',*,*,#6394,.T.);
#8361=ORIENTED_EDGE('',*,*,#6408,.F.);
#8362=ORIENTED_EDGE('',*,*,#6078,.T.);
#8363=ORIENTED_EDGE('',*,*,#6409,.F.);
#8364=ORIENTED_EDGE('',*,*,#6234,.F.);
#8365=ORIENTED_EDGE('',*,*,#6410,.T.);
#8366=ORIENTED_EDGE('',*,*,#6079,.T.);
#8367=ORIENTED_EDGE('',*,*,#6408,.T.);
#8368=ORIENTED_EDGE('',*,*,#6233,.F.);
#8369=ORIENTED_EDGE('',*,*,#6411,.F.);
#8370=ORIENTED_EDGE('',*,*,#6080,.T.);
#8371=ORIENTED_EDGE('',*,*,#6410,.F.);
#8372=ORIENTED_EDGE('',*,*,#6232,.F.);
#8373=ORIENTED_EDGE('',*,*,#6412,.T.);
#8374=ORIENTED_EDGE('',*,*,#6387,.T.);
#8375=ORIENTED_EDGE('',*,*,#6082,.T.);
#8376=ORIENTED_EDGE('',*,*,#6413,.T.);
#8377=ORIENTED_EDGE('',*,*,#6414,.T.);
#8378=ORIENTED_EDGE('',*,*,#6415,.T.);
#8379=ORIENTED_EDGE('',*,*,#6084,.T.);
#8380=ORIENTED_EDGE('',*,*,#6390,.T.);
#8381=ORIENTED_EDGE('',*,*,#6416,.F.);
#8382=ORIENTED_EDGE('',*,*,#6086,.T.);
#8383=ORIENTED_EDGE('',*,*,#6417,.F.);
#8384=ORIENTED_EDGE('',*,*,#6418,.F.);
#8385=ORIENTED_EDGE('',*,*,#6096,.F.);
#8386=ORIENTED_EDGE('',*,*,#6091,.T.);
#8387=ORIENTED_EDGE('',*,*,#6089,.F.);
#8388=ORIENTED_EDGE('',*,*,#6087,.T.);
#8389=ORIENTED_EDGE('',*,*,#6416,.T.);
#8390=ORIENTED_EDGE('',*,*,#6419,.T.);
#8391=ORIENTED_EDGE('',*,*,#6420,.T.);
#8392=ORIENTED_EDGE('',*,*,#6221,.F.);
#8393=ORIENTED_EDGE('',*,*,#6093,.F.);
#8394=ORIENTED_EDGE('',*,*,#6220,.F.);
#8395=ORIENTED_EDGE('',*,*,#6421,.F.);
#8396=ORIENTED_EDGE('',*,*,#6422,.T.);
#8397=ORIENTED_EDGE('',*,*,#6423,.T.);
#8398=ORIENTED_EDGE('',*,*,#6098,.T.);
#8399=ORIENTED_EDGE('',*,*,#6386,.T.);
#8400=ORIENTED_EDGE('',*,*,#6424,.F.);
#8401=ORIENTED_EDGE('',*,*,#6100,.T.);
#8402=ORIENTED_EDGE('',*,*,#6425,.F.);
#8403=ORIENTED_EDGE('',*,*,#6426,.F.);
#8404=ORIENTED_EDGE('',*,*,#6427,.T.);
#8405=ORIENTED_EDGE('',*,*,#6101,.T.);
#8406=ORIENTED_EDGE('',*,*,#6424,.T.);
#8407=ORIENTED_EDGE('',*,*,#6428,.T.);
#8408=ORIENTED_EDGE('',*,*,#6429,.F.);
#8409=ORIENTED_EDGE('',*,*,#6102,.T.);
#8410=ORIENTED_EDGE('',*,*,#6427,.F.);
#8411=ORIENTED_EDGE('',*,*,#6430,.F.);
#8412=ORIENTED_EDGE('',*,*,#6431,.T.);
#8413=ORIENTED_EDGE('',*,*,#6395,.T.);
#8414=ORIENTED_EDGE('',*,*,#6104,.T.);
#8415=ORIENTED_EDGE('',*,*,#6432,.T.);
#8416=ORIENTED_EDGE('',*,*,#6346,.F.);
#8417=ORIENTED_EDGE('',*,*,#6116,.T.);
#8418=ORIENTED_EDGE('',*,*,#6333,.F.);
#8419=ORIENTED_EDGE('',*,*,#6433,.F.);
#8420=ORIENTED_EDGE('',*,*,#6434,.T.);
#8421=ORIENTED_EDGE('',*,*,#6399,.T.);
#8422=ORIENTED_EDGE('',*,*,#6118,.T.);
#8423=ORIENTED_EDGE('',*,*,#6349,.F.);
#8424=ORIENTED_EDGE('',*,*,#6435,.T.);
#8425=ORIENTED_EDGE('',*,*,#6353,.F.);
#8426=ORIENTED_EDGE('',*,*,#6120,.T.);
#8427=ORIENTED_EDGE('',*,*,#6402,.T.);
#8428=ORIENTED_EDGE('',*,*,#6436,.T.);
#8429=ORIENTED_EDGE('',*,*,#6403,.T.);
#8430=ORIENTED_EDGE('',*,*,#6126,.T.);
#8431=ORIENTED_EDGE('',*,*,#6359,.F.);
#8432=ORIENTED_EDGE('',*,*,#6132,.T.);
#8433=ORIENTED_EDGE('',*,*,#6130,.F.);
#8434=ORIENTED_EDGE('',*,*,#6205,.T.);
#8435=ORIENTED_EDGE('',*,*,#6437,.T.);
#8436=ORIENTED_EDGE('',*,*,#6135,.T.);
#8437=ORIENTED_EDGE('',*,*,#6437,.F.);
#8438=ORIENTED_EDGE('',*,*,#6204,.T.);
#8439=ORIENTED_EDGE('',*,*,#6438,.T.);
#8440=ORIENTED_EDGE('',*,*,#6138,.T.);
#8441=ORIENTED_EDGE('',*,*,#6438,.F.);
#8442=ORIENTED_EDGE('',*,*,#6203,.T.);
#8443=ORIENTED_EDGE('',*,*,#6439,.T.);
#8444=ORIENTED_EDGE('',*,*,#6142,.F.);
#8445=ORIENTED_EDGE('',*,*,#6440,.T.);
#8446=ORIENTED_EDGE('',*,*,#6202,.T.);
#8447=ORIENTED_EDGE('',*,*,#6441,.T.);
#8448=ORIENTED_EDGE('',*,*,#6201,.T.);
#8449=ORIENTED_EDGE('',*,*,#6442,.T.);
#8450=ORIENTED_EDGE('',*,*,#6149,.T.);
#8451=ORIENTED_EDGE('',*,*,#6443,.T.);
#8452=ORIENTED_EDGE('',*,*,#6151,.T.);
#8453=ORIENTED_EDGE('',*,*,#6442,.F.);
#8454=ORIENTED_EDGE('',*,*,#6200,.T.);
#8455=ORIENTED_EDGE('',*,*,#6444,.T.);
#8456=ORIENTED_EDGE('',*,*,#6154,.T.);
#8457=ORIENTED_EDGE('',*,*,#6444,.F.);
#8458=ORIENTED_EDGE('',*,*,#6199,.T.);
#8459=ORIENTED_EDGE('',*,*,#6445,.T.);
#8460=ORIENTED_EDGE('',*,*,#6158,.F.);
#8461=ORIENTED_EDGE('',*,*,#6446,.T.);
#8462=ORIENTED_EDGE('',*,*,#6198,.T.);
#8463=ORIENTED_EDGE('',*,*,#6447,.T.);
#8464=ORIENTED_EDGE('',*,*,#6197,.T.);
#8465=ORIENTED_EDGE('',*,*,#6448,.T.);
#8466=ORIENTED_EDGE('',*,*,#6165,.T.);
#8467=ORIENTED_EDGE('',*,*,#6449,.T.);
#8468=ORIENTED_EDGE('',*,*,#6167,.T.);
#8469=ORIENTED_EDGE('',*,*,#6448,.F.);
#8470=ORIENTED_EDGE('',*,*,#6196,.T.);
#8471=ORIENTED_EDGE('',*,*,#6450,.T.);
#8472=ORIENTED_EDGE('',*,*,#6170,.T.);
#8473=ORIENTED_EDGE('',*,*,#6450,.F.);
#8474=ORIENTED_EDGE('',*,*,#6195,.T.);
#8475=ORIENTED_EDGE('',*,*,#6451,.T.);
#8476=ORIENTED_EDGE('',*,*,#6174,.F.);
#8477=ORIENTED_EDGE('',*,*,#6452,.T.);
#8478=ORIENTED_EDGE('',*,*,#6194,.T.);
#8479=ORIENTED_EDGE('',*,*,#6453,.T.);
#8480=ORIENTED_EDGE('',*,*,#6193,.T.);
#8481=ORIENTED_EDGE('',*,*,#6454,.T.);
#8482=ORIENTED_EDGE('',*,*,#6181,.T.);
#8483=ORIENTED_EDGE('',*,*,#6455,.T.);
#8484=ORIENTED_EDGE('',*,*,#6183,.T.);
#8485=ORIENTED_EDGE('',*,*,#6454,.F.);
#8486=ORIENTED_EDGE('',*,*,#6192,.T.);
#8487=ORIENTED_EDGE('',*,*,#6456,.T.);
#8488=ORIENTED_EDGE('',*,*,#6184,.T.);
#8489=ORIENTED_EDGE('',*,*,#6456,.F.);
#8490=ORIENTED_EDGE('',*,*,#6206,.T.);
#8491=ORIENTED_EDGE('',*,*,#6186,.F.);
#8492=ORIENTED_EDGE('',*,*,#6457,.F.);
#8493=ORIENTED_EDGE('',*,*,#6188,.T.);
#8494=ORIENTED_EDGE('',*,*,#6207,.F.);
#8495=ORIENTED_EDGE('',*,*,#6238,.F.);
#8496=ORIENTED_EDGE('',*,*,#6457,.T.);
#8497=ORIENTED_EDGE('',*,*,#6237,.F.);
#8498=ORIENTED_EDGE('',*,*,#6458,.T.);
#8499=ORIENTED_EDGE('',*,*,#6459,.T.);
#8500=ORIENTED_EDGE('',*,*,#6189,.T.);
#8501=ORIENTED_EDGE('',*,*,#6460,.T.);
#8502=ORIENTED_EDGE('',*,*,#6391,.T.);
#8503=ORIENTED_EDGE('',*,*,#6190,.T.);
#8504=ORIENTED_EDGE('',*,*,#6459,.F.);
#8505=ORIENTED_EDGE('',*,*,#6253,.F.);
#8506=ORIENTED_EDGE('',*,*,#6461,.T.);
#8507=ORIENTED_EDGE('',*,*,#6239,.F.);
#8508=ORIENTED_EDGE('',*,*,#6210,.T.);
#8509=ORIENTED_EDGE('',*,*,#6272,.F.);
#8510=ORIENTED_EDGE('',*,*,#6276,.F.);
#8511=ORIENTED_EDGE('',*,*,#6213,.F.);
#8512=ORIENTED_EDGE('',*,*,#6462,.F.);
#8513=ORIENTED_EDGE('',*,*,#6258,.F.);
#8514=ORIENTED_EDGE('',*,*,#6270,.F.);
#8515=ORIENTED_EDGE('',*,*,#6259,.F.);
#8516=ORIENTED_EDGE('',*,*,#6462,.T.);
#8517=ORIENTED_EDGE('',*,*,#6212,.F.);
#8518=ORIENTED_EDGE('',*,*,#6463,.T.);
#8519=ORIENTED_EDGE('',*,*,#6260,.F.);
#8520=ORIENTED_EDGE('',*,*,#6463,.F.);
#8521=ORIENTED_EDGE('',*,*,#6248,.F.);
#8522=ORIENTED_EDGE('',*,*,#6464,.F.);
#8523=ORIENTED_EDGE('',*,*,#6465,.F.);
#8524=ORIENTED_EDGE('',*,*,#6466,.T.);
#8525=ORIENTED_EDGE('',*,*,#6467,.F.);
#8526=ORIENTED_EDGE('',*,*,#6247,.F.);
#8527=ORIENTED_EDGE('',*,*,#6246,.F.);
#8528=ORIENTED_EDGE('',*,*,#6468,.F.);
#8529=ORIENTED_EDGE('',*,*,#6264,.F.);
#8530=ORIENTED_EDGE('',*,*,#6469,.F.);
#8531=ORIENTED_EDGE('',*,*,#6470,.F.);
#8532=ORIENTED_EDGE('',*,*,#6265,.F.);
#8533=ORIENTED_EDGE('',*,*,#6468,.T.);
#8534=ORIENTED_EDGE('',*,*,#6245,.F.);
#8535=ORIENTED_EDGE('',*,*,#6471,.T.);
#8536=ORIENTED_EDGE('',*,*,#6266,.F.);
#8537=ORIENTED_EDGE('',*,*,#6471,.F.);
#8538=ORIENTED_EDGE('',*,*,#6244,.F.);
#8539=ORIENTED_EDGE('',*,*,#6472,.F.);
#8540=ORIENTED_EDGE('',*,*,#6267,.F.);
#8541=ORIENTED_EDGE('',*,*,#6472,.T.);
#8542=ORIENTED_EDGE('',*,*,#6243,.F.);
#8543=ORIENTED_EDGE('',*,*,#6473,.T.);
#8544=ORIENTED_EDGE('',*,*,#6268,.F.);
#8545=ORIENTED_EDGE('',*,*,#6473,.F.);
#8546=ORIENTED_EDGE('',*,*,#6242,.F.);
#8547=ORIENTED_EDGE('',*,*,#6474,.F.);
#8548=ORIENTED_EDGE('',*,*,#6475,.F.);
#8549=ORIENTED_EDGE('',*,*,#6476,.T.);
#8550=ORIENTED_EDGE('',*,*,#6477,.F.);
#8551=ORIENTED_EDGE('',*,*,#6241,.F.);
#8552=ORIENTED_EDGE('',*,*,#6240,.F.);
#8553=ORIENTED_EDGE('',*,*,#6461,.F.);
#8554=ORIENTED_EDGE('',*,*,#6252,.F.);
#8555=ORIENTED_EDGE('',*,*,#6478,.F.);
#8556=ORIENTED_EDGE('',*,*,#6479,.F.);
#8557=ORIENTED_EDGE('',*,*,#6480,.T.);
#8558=ORIENTED_EDGE('',*,*,#6481,.T.);
#8559=ORIENTED_EDGE('',*,*,#6236,.F.);
#8560=ORIENTED_EDGE('',*,*,#6409,.T.);
#8561=ORIENTED_EDGE('',*,*,#6077,.T.);
#8562=ORIENTED_EDGE('',*,*,#6407,.F.);
#8563=ORIENTED_EDGE('',*,*,#6482,.T.);
#8564=ORIENTED_EDGE('',*,*,#6235,.F.);
#8565=ORIENTED_EDGE('',*,*,#6411,.T.);
#8566=ORIENTED_EDGE('',*,*,#6231,.F.);
#8567=ORIENTED_EDGE('',*,*,#6483,.T.);
#8568=ORIENTED_EDGE('',*,*,#6413,.F.);
#8569=ORIENTED_EDGE('',*,*,#6081,.T.);
#8570=ORIENTED_EDGE('',*,*,#6484,.T.);
#8571=ORIENTED_EDGE('',*,*,#6485,.T.);
#8572=ORIENTED_EDGE('',*,*,#6230,.F.);
#8573=ORIENTED_EDGE('',*,*,#6486,.T.);
#8574=ORIENTED_EDGE('',*,*,#6229,.F.);
#8575=ORIENTED_EDGE('',*,*,#6487,.T.);
#8576=ORIENTED_EDGE('',*,*,#6488,.T.);
#8577=ORIENTED_EDGE('',*,*,#6417,.T.);
#8578=ORIENTED_EDGE('',*,*,#6085,.T.);
#8579=ORIENTED_EDGE('',*,*,#6415,.F.);
#8580=ORIENTED_EDGE('',*,*,#6489,.T.);
#8581=ORIENTED_EDGE('',*,*,#6487,.F.);
#8582=ORIENTED_EDGE('',*,*,#6228,.F.);
#8583=ORIENTED_EDGE('',*,*,#6490,.T.);
#8584=ORIENTED_EDGE('',*,*,#6226,.F.);
#8585=ORIENTED_EDGE('',*,*,#6491,.F.);
#8586=ORIENTED_EDGE('',*,*,#6492,.F.);
#8587=ORIENTED_EDGE('',*,*,#6493,.F.);
#8588=ORIENTED_EDGE('',*,*,#6494,.F.);
#8589=ORIENTED_EDGE('',*,*,#6495,.F.);
#8590=ORIENTED_EDGE('',*,*,#6491,.T.);
#8591=ORIENTED_EDGE('',*,*,#6225,.F.);
#8592=ORIENTED_EDGE('',*,*,#6496,.F.);
#8593=ORIENTED_EDGE('',*,*,#6494,.T.);
#8594=ORIENTED_EDGE('',*,*,#6224,.F.);
#8595=ORIENTED_EDGE('',*,*,#6497,.F.);
#8596=ORIENTED_EDGE('',*,*,#6498,.T.);
#8597=ORIENTED_EDGE('',*,*,#6499,.T.);
#8598=ORIENTED_EDGE('',*,*,#6222,.F.);
#8599=ORIENTED_EDGE('',*,*,#6420,.F.);
#8600=ORIENTED_EDGE('',*,*,#6421,.T.);
#8601=ORIENTED_EDGE('',*,*,#6219,.F.);
#8602=ORIENTED_EDGE('',*,*,#6500,.F.);
#8603=ORIENTED_EDGE('',*,*,#6501,.F.);
#8604=ORIENTED_EDGE('',*,*,#6218,.F.);
#8605=ORIENTED_EDGE('',*,*,#6502,.T.);
#8606=ORIENTED_EDGE('',*,*,#6503,.T.);
#8607=ORIENTED_EDGE('',*,*,#6504,.T.);
#8608=ORIENTED_EDGE('',*,*,#6505,.T.);
#8609=ORIENTED_EDGE('',*,*,#6500,.T.);
#8610=ORIENTED_EDGE('',*,*,#6217,.F.);
#8611=ORIENTED_EDGE('',*,*,#6506,.T.);
#8612=ORIENTED_EDGE('',*,*,#6507,.T.);
#8613=ORIENTED_EDGE('',*,*,#6502,.F.);
#8614=ORIENTED_EDGE('',*,*,#6508,.F.);
#8615=ORIENTED_EDGE('',*,*,#6509,.F.);
#8616=ORIENTED_EDGE('',*,*,#6510,.F.);
#8617=ORIENTED_EDGE('',*,*,#6511,.F.);
#8618=ORIENTED_EDGE('',*,*,#6506,.F.);
#8619=ORIENTED_EDGE('',*,*,#6216,.F.);
#8620=ORIENTED_EDGE('',*,*,#6508,.T.);
#8621=ORIENTED_EDGE('',*,*,#6215,.F.);
#8622=ORIENTED_EDGE('',*,*,#6512,.T.);
#8623=ORIENTED_EDGE('',*,*,#6513,.T.);
#8624=ORIENTED_EDGE('',*,*,#6512,.F.);
#8625=ORIENTED_EDGE('',*,*,#6214,.F.);
#8626=ORIENTED_EDGE('',*,*,#6275,.F.);
#8627=ORIENTED_EDGE('',*,*,#6514,.F.);
#8628=ORIENTED_EDGE('',*,*,#6515,.F.);
#8629=ORIENTED_EDGE('',*,*,#6478,.T.);
#8630=ORIENTED_EDGE('',*,*,#6251,.F.);
#8631=ORIENTED_EDGE('',*,*,#6516,.T.);
#8632=ORIENTED_EDGE('',*,*,#6274,.F.);
#8633=ORIENTED_EDGE('',*,*,#6278,.F.);
#8634=ORIENTED_EDGE('',*,*,#6517,.T.);
#8635=ORIENTED_EDGE('',*,*,#6518,.T.);
#8636=ORIENTED_EDGE('',*,*,#6519,.T.);
#8637=ORIENTED_EDGE('',*,*,#5851,.T.);
#8638=ORIENTED_EDGE('',*,*,#6520,.T.);
#8639=ORIENTED_EDGE('',*,*,#6521,.T.);
#8640=ORIENTED_EDGE('',*,*,#6262,.F.);
#8641=ORIENTED_EDGE('',*,*,#6522,.T.);
#8642=ORIENTED_EDGE('',*,*,#6523,.T.);
#8643=ORIENTED_EDGE('',*,*,#5854,.T.);
#8644=ORIENTED_EDGE('',*,*,#6514,.T.);
#8645=ORIENTED_EDGE('',*,*,#6250,.T.);
#8646=ORIENTED_EDGE('',*,*,#6310,.F.);
#8647=ORIENTED_EDGE('',*,*,#6255,.F.);
#8648=ORIENTED_EDGE('',*,*,#6524,.T.);
#8649=ORIENTED_EDGE('',*,*,#6525,.T.);
#8650=ORIENTED_EDGE('',*,*,#6526,.T.);
#8651=ORIENTED_EDGE('',*,*,#5857,.T.);
#8652=ORIENTED_EDGE('',*,*,#6527,.T.);
#8653=ORIENTED_EDGE('',*,*,#6280,.F.);
#8654=ORIENTED_EDGE('',*,*,#6290,.F.);
#8655=ORIENTED_EDGE('',*,*,#6528,.T.);
#8656=ORIENTED_EDGE('',*,*,#6529,.T.);
#8657=ORIENTED_EDGE('',*,*,#6530,.T.);
#8658=ORIENTED_EDGE('',*,*,#5860,.T.);
#8659=ORIENTED_EDGE('',*,*,#6531,.T.);
#8660=ORIENTED_EDGE('',*,*,#6532,.T.);
#8661=ORIENTED_EDGE('',*,*,#6306,.F.);
#8662=ORIENTED_EDGE('',*,*,#6533,.T.);
#8663=ORIENTED_EDGE('',*,*,#6534,.T.);
#8664=ORIENTED_EDGE('',*,*,#5863,.T.);
#8665=ORIENTED_EDGE('',*,*,#6535,.T.);
#8666=ORIENTED_EDGE('',*,*,#6298,.F.);
#8667=ORIENTED_EDGE('',*,*,#6309,.F.);
#8668=ORIENTED_EDGE('',*,*,#6020,.T.);
#8669=ORIENTED_EDGE('',*,*,#6313,.T.);
#8670=ORIENTED_EDGE('',*,*,#6536,.T.);
#8671=ORIENTED_EDGE('',*,*,#6537,.T.);
#8672=ORIENTED_EDGE('',*,*,#5866,.T.);
#8673=ORIENTED_EDGE('',*,*,#6475,.T.);
#8674=ORIENTED_EDGE('',*,*,#6538,.F.);
#8675=ORIENTED_EDGE('',*,*,#6524,.F.);
#8676=ORIENTED_EDGE('',*,*,#6254,.F.);
#8677=ORIENTED_EDGE('',*,*,#6521,.F.);
#8678=ORIENTED_EDGE('',*,*,#6539,.F.);
#8679=ORIENTED_EDGE('',*,*,#6469,.T.);
#8680=ORIENTED_EDGE('',*,*,#6263,.F.);
#8681=ORIENTED_EDGE('',*,*,#6465,.T.);
#8682=ORIENTED_EDGE('',*,*,#6540,.F.);
#8683=ORIENTED_EDGE('',*,*,#6522,.F.);
#8684=ORIENTED_EDGE('',*,*,#6261,.F.);
#8685=ORIENTED_EDGE('',*,*,#6541,.F.);
#8686=ORIENTED_EDGE('',*,*,#6542,.F.);
#8687=ORIENTED_EDGE('',*,*,#6517,.F.);
#8688=ORIENTED_EDGE('',*,*,#6277,.F.);
#8689=ORIENTED_EDGE('',*,*,#6285,.F.);
#8690=ORIENTED_EDGE('',*,*,#6543,.T.);
#8691=ORIENTED_EDGE('',*,*,#6544,.T.);
#8692=ORIENTED_EDGE('',*,*,#6545,.T.);
#8693=ORIENTED_EDGE('',*,*,#6284,.F.);
#8694=ORIENTED_EDGE('',*,*,#6546,.F.);
#8695=ORIENTED_EDGE('',*,*,#6547,.F.);
#8696=ORIENTED_EDGE('',*,*,#6543,.F.);
#8697=ORIENTED_EDGE('',*,*,#6283,.F.);
#8698=ORIENTED_EDGE('',*,*,#6548,.T.);
#8699=ORIENTED_EDGE('',*,*,#6549,.T.);
#8700=ORIENTED_EDGE('',*,*,#6546,.T.);
#8701=ORIENTED_EDGE('',*,*,#6527,.F.);
#8702=ORIENTED_EDGE('',*,*,#6550,.F.);
#8703=ORIENTED_EDGE('',*,*,#6551,.F.);
#8704=ORIENTED_EDGE('',*,*,#6281,.F.);
#8705=ORIENTED_EDGE('',*,*,#6532,.F.);
#8706=ORIENTED_EDGE('',*,*,#6552,.F.);
#8707=ORIENTED_EDGE('',*,*,#6378,.T.);
#8708=ORIENTED_EDGE('',*,*,#6307,.F.);
#8709=ORIENTED_EDGE('',*,*,#6374,.T.);
#8710=ORIENTED_EDGE('',*,*,#6553,.F.);
#8711=ORIENTED_EDGE('',*,*,#6533,.F.);
#8712=ORIENTED_EDGE('',*,*,#6305,.F.);
#8713=ORIENTED_EDGE('',*,*,#6535,.F.);
#8714=ORIENTED_EDGE('',*,*,#6554,.F.);
#8715=ORIENTED_EDGE('',*,*,#6368,.T.);
#8716=ORIENTED_EDGE('',*,*,#6299,.F.);
#8717=ORIENTED_EDGE('',*,*,#5869,.F.);
#8718=ORIENTED_EDGE('',*,*,#5873,.F.);
#8719=ORIENTED_EDGE('',*,*,#6366,.T.);
#8720=ORIENTED_EDGE('',*,*,#6555,.F.);
#8721=ORIENTED_EDGE('',*,*,#6536,.F.);
#8722=ORIENTED_EDGE('',*,*,#6312,.T.);
#8723=ORIENTED_EDGE('',*,*,#6315,.T.);
#8724=ORIENTED_EDGE('',*,*,#6320,.T.);
#8725=ORIENTED_EDGE('',*,*,#6556,.F.);
#8726=ORIENTED_EDGE('',*,*,#6528,.F.);
#8727=ORIENTED_EDGE('',*,*,#6317,.F.);
#8728=ORIENTED_EDGE('',*,*,#6557,.F.);
#8729=ORIENTED_EDGE('',*,*,#6558,.F.);
#8730=ORIENTED_EDGE('',*,*,#6529,.F.);
#8731=ORIENTED_EDGE('',*,*,#6556,.T.);
#8732=ORIENTED_EDGE('',*,*,#6319,.T.);
#8733=ORIENTED_EDGE('',*,*,#6559,.T.);
#8734=ORIENTED_EDGE('',*,*,#6503,.F.);
#8735=ORIENTED_EDGE('',*,*,#6507,.F.);
#8736=ORIENTED_EDGE('',*,*,#6511,.T.);
#8737=ORIENTED_EDGE('',*,*,#6560,.T.);
#8738=ORIENTED_EDGE('',*,*,#6561,.T.);
#8739=ORIENTED_EDGE('',*,*,#6544,.F.);
#8740=ORIENTED_EDGE('',*,*,#6547,.T.);
#8741=ORIENTED_EDGE('',*,*,#6549,.F.);
#8742=ORIENTED_EDGE('',*,*,#6562,.T.);
#8743=ORIENTED_EDGE('',*,*,#6563,.T.);
#8744=ORIENTED_EDGE('',*,*,#6322,.T.);
#8745=ORIENTED_EDGE('',*,*,#6323,.F.);
#8746=ORIENTED_EDGE('',*,*,#6325,.F.);
#8747=ORIENTED_EDGE('',*,*,#6564,.T.);
#8748=ORIENTED_EDGE('',*,*,#6565,.T.);
#8749=ORIENTED_EDGE('',*,*,#6430,.T.);
#8750=ORIENTED_EDGE('',*,*,#6428,.F.);
#8751=ORIENTED_EDGE('',*,*,#6426,.T.);
#8752=ORIENTED_EDGE('',*,*,#6566,.T.);
#8753=ORIENTED_EDGE('',*,*,#6567,.T.);
#8754=ORIENTED_EDGE('',*,*,#6568,.T.);
#8755=ORIENTED_EDGE('',*,*,#6328,.F.);
#8756=ORIENTED_EDGE('',*,*,#6569,.T.);
#8757=ORIENTED_EDGE('',*,*,#6397,.T.);
#8758=ORIENTED_EDGE('',*,*,#6569,.F.);
#8759=ORIENTED_EDGE('',*,*,#6327,.F.);
#8760=ORIENTED_EDGE('',*,*,#6329,.T.);
#8761=ORIENTED_EDGE('',*,*,#6398,.T.);
#8762=ORIENTED_EDGE('',*,*,#6347,.F.);
#8763=ORIENTED_EDGE('',*,*,#6433,.T.);
#8764=ORIENTED_EDGE('',*,*,#6332,.F.);
#8765=ORIENTED_EDGE('',*,*,#6334,.F.);
#8766=ORIENTED_EDGE('',*,*,#6570,.T.);
#8767=ORIENTED_EDGE('',*,*,#6343,.F.);
#8768=ORIENTED_EDGE('',*,*,#6338,.T.);
#8769=ORIENTED_EDGE('',*,*,#6571,.F.);
#8770=ORIENTED_EDGE('',*,*,#6342,.T.);
#8771=ORIENTED_EDGE('',*,*,#6054,.F.);
#8772=ORIENTED_EDGE('',*,*,#6344,.F.);
#8773=ORIENTED_EDGE('',*,*,#6570,.F.);
#8774=ORIENTED_EDGE('',*,*,#6335,.F.);
#8775=ORIENTED_EDGE('',*,*,#6058,.F.);
#8776=ORIENTED_EDGE('',*,*,#6572,.F.);
#8777=ORIENTED_EDGE('',*,*,#6573,.F.);
#8778=ORIENTED_EDGE('',*,*,#6574,.F.);
#8779=ORIENTED_EDGE('',*,*,#6575,.F.);
#8780=ORIENTED_EDGE('',*,*,#6337,.T.);
#8781=ORIENTED_EDGE('',*,*,#6340,.T.);
#8782=ORIENTED_EDGE('',*,*,#6341,.T.);
#8783=ORIENTED_EDGE('',*,*,#6571,.T.);
#8784=ORIENTED_EDGE('',*,*,#6400,.T.);
#8785=ORIENTED_EDGE('',*,*,#6434,.F.);
#8786=ORIENTED_EDGE('',*,*,#6348,.F.);
#8787=ORIENTED_EDGE('',*,*,#6351,.F.);
#8788=ORIENTED_EDGE('',*,*,#6576,.T.);
#8789=ORIENTED_EDGE('',*,*,#6576,.F.);
#8790=ORIENTED_EDGE('',*,*,#6350,.T.);
#8791=ORIENTED_EDGE('',*,*,#6354,.F.);
#8792=ORIENTED_EDGE('',*,*,#6435,.F.);
#8793=ORIENTED_EDGE('',*,*,#6401,.T.);
#8794=ORIENTED_EDGE('',*,*,#6404,.T.);
#8795=ORIENTED_EDGE('',*,*,#6436,.F.);
#8796=ORIENTED_EDGE('',*,*,#6358,.F.);
#8797=ORIENTED_EDGE('',*,*,#6361,.F.);
#8798=ORIENTED_EDGE('',*,*,#6577,.T.);
#8799=ORIENTED_EDGE('',*,*,#6577,.F.);
#8800=ORIENTED_EDGE('',*,*,#6360,.T.);
#8801=ORIENTED_EDGE('',*,*,#6364,.F.);
#8802=ORIENTED_EDGE('',*,*,#6381,.F.);
#8803=ORIENTED_EDGE('',*,*,#6405,.T.);
#8804=ORIENTED_EDGE('',*,*,#6554,.T.);
#8805=ORIENTED_EDGE('',*,*,#6537,.F.);
#8806=ORIENTED_EDGE('',*,*,#6555,.T.);
#8807=ORIENTED_EDGE('',*,*,#6365,.F.);
#8808=ORIENTED_EDGE('',*,*,#6369,.T.);
#8809=ORIENTED_EDGE('',*,*,#6376,.T.);
#8810=ORIENTED_EDGE('',*,*,#6578,.F.);
#8811=ORIENTED_EDGE('',*,*,#6534,.F.);
#8812=ORIENTED_EDGE('',*,*,#6553,.T.);
#8813=ORIENTED_EDGE('',*,*,#6373,.T.);
#8814=ORIENTED_EDGE('',*,*,#6552,.T.);
#8815=ORIENTED_EDGE('',*,*,#6531,.F.);
#8816=ORIENTED_EDGE('',*,*,#6578,.T.);
#8817=ORIENTED_EDGE('',*,*,#6375,.F.);
#8818=ORIENTED_EDGE('',*,*,#6379,.T.);
#8819=ORIENTED_EDGE('',*,*,#6579,.T.);
#8820=ORIENTED_EDGE('',*,*,#6383,.T.);
#8821=ORIENTED_EDGE('',*,*,#6501,.T.);
#8822=ORIENTED_EDGE('',*,*,#6505,.F.);
#8823=ORIENTED_EDGE('',*,*,#6384,.T.);
#8824=ORIENTED_EDGE('',*,*,#6579,.F.);
#8825=ORIENTED_EDGE('',*,*,#6504,.F.);
#8826=ORIENTED_EDGE('',*,*,#6580,.T.);
#8827=ORIENTED_EDGE('',*,*,#6581,.T.);
#8828=ORIENTED_EDGE('',*,*,#6581,.F.);
#8829=ORIENTED_EDGE('',*,*,#6582,.T.);
#8830=ORIENTED_EDGE('',*,*,#6583,.T.);
#8831=ORIENTED_EDGE('',*,*,#6422,.F.);
#8832=ORIENTED_EDGE('',*,*,#6385,.T.);
#8833=ORIENTED_EDGE('',*,*,#6388,.T.);
#8834=ORIENTED_EDGE('',*,*,#6412,.F.);
#8835=ORIENTED_EDGE('',*,*,#6483,.F.);
#8836=ORIENTED_EDGE('',*,*,#6485,.F.);
#8837=ORIENTED_EDGE('',*,*,#6584,.T.);
#8838=ORIENTED_EDGE('',*,*,#6584,.F.);
#8839=ORIENTED_EDGE('',*,*,#6484,.F.);
#8840=ORIENTED_EDGE('',*,*,#6486,.F.);
#8841=ORIENTED_EDGE('',*,*,#6414,.F.);
#8842=ORIENTED_EDGE('',*,*,#6389,.T.);
#8843=ORIENTED_EDGE('',*,*,#6392,.T.);
#8844=ORIENTED_EDGE('',*,*,#6460,.F.);
#8845=ORIENTED_EDGE('',*,*,#6458,.F.);
#8846=ORIENTED_EDGE('',*,*,#6481,.F.);
#8847=ORIENTED_EDGE('',*,*,#6585,.T.);
#8848=ORIENTED_EDGE('',*,*,#6585,.F.);
#8849=ORIENTED_EDGE('',*,*,#6480,.F.);
#8850=ORIENTED_EDGE('',*,*,#6482,.F.);
#8851=ORIENTED_EDGE('',*,*,#6406,.F.);
#8852=ORIENTED_EDGE('',*,*,#6393,.T.);
#8853=ORIENTED_EDGE('',*,*,#6396,.T.);
#8854=ORIENTED_EDGE('',*,*,#6431,.F.);
#8855=ORIENTED_EDGE('',*,*,#6586,.T.);
#8856=ORIENTED_EDGE('',*,*,#6587,.T.);
#8857=ORIENTED_EDGE('',*,*,#6567,.F.);
#8858=ORIENTED_EDGE('',*,*,#6588,.T.);
#8859=ORIENTED_EDGE('',*,*,#6498,.F.);
#8860=ORIENTED_EDGE('',*,*,#6419,.F.);
#8861=ORIENTED_EDGE('',*,*,#6418,.T.);
#8862=ORIENTED_EDGE('',*,*,#6488,.F.);
#8863=ORIENTED_EDGE('',*,*,#6489,.F.);
#8864=ORIENTED_EDGE('',*,*,#6425,.T.);
#8865=ORIENTED_EDGE('',*,*,#6099,.T.);
#8866=ORIENTED_EDGE('',*,*,#6423,.F.);
#8867=ORIENTED_EDGE('',*,*,#6583,.F.);
#8868=ORIENTED_EDGE('',*,*,#6566,.F.);
#8869=ORIENTED_EDGE('',*,*,#6429,.T.);
#8870=ORIENTED_EDGE('',*,*,#6565,.F.);
#8871=ORIENTED_EDGE('',*,*,#6586,.F.);
#8872=ORIENTED_EDGE('',*,*,#6432,.F.);
#8873=ORIENTED_EDGE('',*,*,#6103,.T.);
#8874=ORIENTED_EDGE('',*,*,#6439,.F.);
#8875=ORIENTED_EDGE('',*,*,#6440,.F.);
#8876=ORIENTED_EDGE('',*,*,#6589,.T.);
#8877=ORIENTED_EDGE('',*,*,#6441,.F.);
#8878=ORIENTED_EDGE('',*,*,#6443,.F.);
#8879=ORIENTED_EDGE('',*,*,#6590,.T.);
#8880=ORIENTED_EDGE('',*,*,#6445,.F.);
#8881=ORIENTED_EDGE('',*,*,#6446,.F.);
#8882=ORIENTED_EDGE('',*,*,#6591,.T.);
#8883=ORIENTED_EDGE('',*,*,#6447,.F.);
#8884=ORIENTED_EDGE('',*,*,#6449,.F.);
#8885=ORIENTED_EDGE('',*,*,#6592,.T.);
#8886=ORIENTED_EDGE('',*,*,#6451,.F.);
#8887=ORIENTED_EDGE('',*,*,#6452,.F.);
#8888=ORIENTED_EDGE('',*,*,#6593,.T.);
#8889=ORIENTED_EDGE('',*,*,#6453,.F.);
#8890=ORIENTED_EDGE('',*,*,#6455,.F.);
#8891=ORIENTED_EDGE('',*,*,#6594,.T.);
#8892=ORIENTED_EDGE('',*,*,#5872,.T.);
#8893=ORIENTED_EDGE('',*,*,#5876,.F.);
#8894=ORIENTED_EDGE('',*,*,#6467,.T.);
#8895=ORIENTED_EDGE('',*,*,#6595,.F.);
#8896=ORIENTED_EDGE('',*,*,#6523,.F.);
#8897=ORIENTED_EDGE('',*,*,#6540,.T.);
#8898=ORIENTED_EDGE('',*,*,#6464,.T.);
#8899=ORIENTED_EDGE('',*,*,#6539,.T.);
#8900=ORIENTED_EDGE('',*,*,#6520,.F.);
#8901=ORIENTED_EDGE('',*,*,#6595,.T.);
#8902=ORIENTED_EDGE('',*,*,#6466,.F.);
#8903=ORIENTED_EDGE('',*,*,#6470,.T.);
#8904=ORIENTED_EDGE('',*,*,#6477,.T.);
#8905=ORIENTED_EDGE('',*,*,#6596,.F.);
#8906=ORIENTED_EDGE('',*,*,#6525,.F.);
#8907=ORIENTED_EDGE('',*,*,#6538,.T.);
#8908=ORIENTED_EDGE('',*,*,#6474,.T.);
#8909=ORIENTED_EDGE('',*,*,#6515,.T.);
#8910=ORIENTED_EDGE('',*,*,#6526,.F.);
#8911=ORIENTED_EDGE('',*,*,#6596,.T.);
#8912=ORIENTED_EDGE('',*,*,#6476,.F.);
#8913=ORIENTED_EDGE('',*,*,#6479,.T.);
#8914=ORIENTED_EDGE('',*,*,#6499,.F.);
#8915=ORIENTED_EDGE('',*,*,#6588,.F.);
#8916=ORIENTED_EDGE('',*,*,#6490,.F.);
#8917=ORIENTED_EDGE('',*,*,#6227,.F.);
#8918=ORIENTED_EDGE('',*,*,#6493,.T.);
#8919=ORIENTED_EDGE('',*,*,#6597,.F.);
#8920=ORIENTED_EDGE('',*,*,#6497,.T.);
#8921=ORIENTED_EDGE('',*,*,#6223,.F.);
#8922=ORIENTED_EDGE('',*,*,#6598,.F.);
#8923=ORIENTED_EDGE('',*,*,#6599,.F.);
#8924=ORIENTED_EDGE('',*,*,#6600,.F.);
#8925=ORIENTED_EDGE('',*,*,#6601,.F.);
#8926=ORIENTED_EDGE('',*,*,#6492,.T.);
#8927=ORIENTED_EDGE('',*,*,#6495,.T.);
#8928=ORIENTED_EDGE('',*,*,#6496,.T.);
#8929=ORIENTED_EDGE('',*,*,#6597,.T.);
#8930=ORIENTED_EDGE('',*,*,#6516,.F.);
#8931=ORIENTED_EDGE('',*,*,#6602,.F.);
#8932=ORIENTED_EDGE('',*,*,#6509,.T.);
#8933=ORIENTED_EDGE('',*,*,#6513,.F.);
#8934=ORIENTED_EDGE('',*,*,#6602,.T.);
#8935=ORIENTED_EDGE('',*,*,#6519,.F.);
#8936=ORIENTED_EDGE('',*,*,#6603,.F.);
#8937=ORIENTED_EDGE('',*,*,#6604,.F.);
#8938=ORIENTED_EDGE('',*,*,#6510,.T.);
#8939=ORIENTED_EDGE('',*,*,#6605,.F.);
#8940=ORIENTED_EDGE('',*,*,#6603,.T.);
#8941=ORIENTED_EDGE('',*,*,#6518,.F.);
#8942=ORIENTED_EDGE('',*,*,#6542,.T.);
#8943=ORIENTED_EDGE('',*,*,#6606,.F.);
#8944=ORIENTED_EDGE('',*,*,#6550,.T.);
#8945=ORIENTED_EDGE('',*,*,#6530,.F.);
#8946=ORIENTED_EDGE('',*,*,#6558,.T.);
#8947=ORIENTED_EDGE('',*,*,#6607,.F.);
#8948=ORIENTED_EDGE('',*,*,#6608,.F.);
#8949=ORIENTED_EDGE('',*,*,#6286,.F.);
#8950=ORIENTED_EDGE('',*,*,#6545,.F.);
#8951=ORIENTED_EDGE('',*,*,#6561,.F.);
#8952=ORIENTED_EDGE('',*,*,#6606,.T.);
#8953=ORIENTED_EDGE('',*,*,#6541,.T.);
#8954=ORIENTED_EDGE('',*,*,#6562,.F.);
#8955=ORIENTED_EDGE('',*,*,#6548,.F.);
#8956=ORIENTED_EDGE('',*,*,#6282,.F.);
#8957=ORIENTED_EDGE('',*,*,#6551,.T.);
#8958=ORIENTED_EDGE('',*,*,#6608,.T.);
#8959=ORIENTED_EDGE('',*,*,#6607,.T.);
#8960=ORIENTED_EDGE('',*,*,#6557,.T.);
#8961=ORIENTED_EDGE('',*,*,#6563,.F.);
#8962=ORIENTED_EDGE('',*,*,#6582,.F.);
#8963=ORIENTED_EDGE('',*,*,#6580,.F.);
#8964=ORIENTED_EDGE('',*,*,#6559,.F.);
#8965=ORIENTED_EDGE('',*,*,#6568,.F.);
#8966=ORIENTED_EDGE('',*,*,#6587,.F.);
#8967=ORIENTED_EDGE('',*,*,#6564,.F.);
#8968=ORIENTED_EDGE('',*,*,#6604,.T.);
#8969=ORIENTED_EDGE('',*,*,#6605,.T.);
#8970=ORIENTED_EDGE('',*,*,#6560,.F.);
#8971=ORIENTED_EDGE('',*,*,#6609,.T.);
#8972=ORIENTED_EDGE('',*,*,#6610,.T.);
#8973=ORIENTED_EDGE('',*,*,#6575,.T.);
#8974=ORIENTED_EDGE('',*,*,#6611,.T.);
#8975=ORIENTED_EDGE('',*,*,#6612,.T.);
#8976=ORIENTED_EDGE('',*,*,#6613,.T.);
#8977=ORIENTED_EDGE('',*,*,#6572,.T.);
#8978=ORIENTED_EDGE('',*,*,#6610,.F.);
#8979=ORIENTED_EDGE('',*,*,#6614,.T.);
#8980=ORIENTED_EDGE('',*,*,#6615,.T.);
#8981=ORIENTED_EDGE('',*,*,#6573,.T.);
#8982=ORIENTED_EDGE('',*,*,#6613,.F.);
#8983=ORIENTED_EDGE('',*,*,#6616,.T.);
#8984=ORIENTED_EDGE('',*,*,#6611,.F.);
#8985=ORIENTED_EDGE('',*,*,#6574,.T.);
#8986=ORIENTED_EDGE('',*,*,#6615,.F.);
#8987=ORIENTED_EDGE('',*,*,#6141,.T.);
#8988=ORIENTED_EDGE('',*,*,#6139,.T.);
#8989=ORIENTED_EDGE('',*,*,#6136,.T.);
#8990=ORIENTED_EDGE('',*,*,#6589,.F.);
#8991=ORIENTED_EDGE('',*,*,#6148,.T.);
#8992=ORIENTED_EDGE('',*,*,#6145,.T.);
#8993=ORIENTED_EDGE('',*,*,#6143,.T.);
#8994=ORIENTED_EDGE('',*,*,#6590,.F.);
#8995=ORIENTED_EDGE('',*,*,#6157,.T.);
#8996=ORIENTED_EDGE('',*,*,#6155,.T.);
#8997=ORIENTED_EDGE('',*,*,#6152,.T.);
#8998=ORIENTED_EDGE('',*,*,#6591,.F.);
#8999=ORIENTED_EDGE('',*,*,#6164,.T.);
#9000=ORIENTED_EDGE('',*,*,#6161,.T.);
#9001=ORIENTED_EDGE('',*,*,#6159,.T.);
#9002=ORIENTED_EDGE('',*,*,#6592,.F.);
#9003=ORIENTED_EDGE('',*,*,#6173,.T.);
#9004=ORIENTED_EDGE('',*,*,#6171,.T.);
#9005=ORIENTED_EDGE('',*,*,#6168,.T.);
#9006=ORIENTED_EDGE('',*,*,#6593,.F.);
#9007=ORIENTED_EDGE('',*,*,#6180,.T.);
#9008=ORIENTED_EDGE('',*,*,#6177,.T.);
#9009=ORIENTED_EDGE('',*,*,#6175,.T.);
#9010=ORIENTED_EDGE('',*,*,#6594,.F.);
#9011=ORIENTED_EDGE('',*,*,#6617,.T.);
#9012=ORIENTED_EDGE('',*,*,#6618,.T.);
#9013=ORIENTED_EDGE('',*,*,#6601,.T.);
#9014=ORIENTED_EDGE('',*,*,#6619,.T.);
#9015=ORIENTED_EDGE('',*,*,#6620,.T.);
#9016=ORIENTED_EDGE('',*,*,#6621,.T.);
#9017=ORIENTED_EDGE('',*,*,#6598,.T.);
#9018=ORIENTED_EDGE('',*,*,#6618,.F.);
#9019=ORIENTED_EDGE('',*,*,#6622,.T.);
#9020=ORIENTED_EDGE('',*,*,#6623,.T.);
#9021=ORIENTED_EDGE('',*,*,#6599,.T.);
#9022=ORIENTED_EDGE('',*,*,#6621,.F.);
#9023=ORIENTED_EDGE('',*,*,#6624,.T.);
#9024=ORIENTED_EDGE('',*,*,#6619,.F.);
#9025=ORIENTED_EDGE('',*,*,#6600,.T.);
#9026=ORIENTED_EDGE('',*,*,#6623,.F.);
#9027=ORIENTED_EDGE('',*,*,#5875,.F.);
#9028=ORIENTED_EDGE('',*,*,#6614,.F.);
#9029=ORIENTED_EDGE('',*,*,#6612,.F.);
#9030=ORIENTED_EDGE('',*,*,#6609,.F.);
#9031=ORIENTED_EDGE('',*,*,#6616,.F.);
#9032=ORIENTED_EDGE('',*,*,#5881,.F.);
#9033=ORIENTED_EDGE('',*,*,#5878,.F.);
#9034=ORIENTED_EDGE('',*,*,#6622,.F.);
#9035=ORIENTED_EDGE('',*,*,#6620,.F.);
#9036=ORIENTED_EDGE('',*,*,#6617,.F.);
#9037=ORIENTED_EDGE('',*,*,#6624,.F.);
#9038=ORIENTED_EDGE('',*,*,#5884,.F.);
#9039=ORIENTED_EDGE('',*,*,#5879,.F.);
#9040=ORIENTED_EDGE('',*,*,#5882,.F.);
#9041=ORIENTED_EDGE('',*,*,#5887,.T.);
#9042=ORIENTED_EDGE('',*,*,#5885,.F.);
#9043=ORIENTED_EDGE('',*,*,#5890,.T.);
#9044=ORIENTED_EDGE('',*,*,#5888,.F.);
#10174=CYLINDRICAL_SURFACE('',#11216,5.5);
#10175=CYLINDRICAL_SURFACE('',#11219,14.);
#10176=CYLINDRICAL_SURFACE('',#11222,1.35);
#10177=CYLINDRICAL_SURFACE('',#11225,1.35);
#10178=CYLINDRICAL_SURFACE('',#11228,1.35);
#10179=CYLINDRICAL_SURFACE('',#11231,1.35);
#10180=CYLINDRICAL_SURFACE('',#11234,1.35);
#10181=CYLINDRICAL_SURFACE('',#11237,1.35);
#10182=CYLINDRICAL_SURFACE('',#11240,1.35);
#10183=CYLINDRICAL_SURFACE('',#11243,1.35);
#10184=CYLINDRICAL_SURFACE('',#11246,1.35);
#10185=CYLINDRICAL_SURFACE('',#11249,1.35);
#10186=CYLINDRICAL_SURFACE('',#11252,1.35);
#10187=CYLINDRICAL_SURFACE('',#11255,1.35);
#10188=CYLINDRICAL_SURFACE('',#11258,5.);
#10189=CYLINDRICAL_SURFACE('',#11261,7.5);
#10190=CYLINDRICAL_SURFACE('',#11264,2.75);
#10191=CYLINDRICAL_SURFACE('',#11267,5.);
#10192=CYLINDRICAL_SURFACE('',#11270,7.25);
#10193=CYLINDRICAL_SURFACE('',#11273,14.);
#10194=CYLINDRICAL_SURFACE('',#11276,4.75);
#10195=CYLINDRICAL_SURFACE('',#11279,2.75);
#10196=CYLINDRICAL_SURFACE('',#11283,2.);
#10197=CYLINDRICAL_SURFACE('',#11286,1.5);
#10198=CYLINDRICAL_SURFACE('',#11289,1.5);
#10199=CYLINDRICAL_SURFACE('',#11292,1.5);
#10200=CYLINDRICAL_SURFACE('',#11306,2.);
#10201=CYLINDRICAL_SURFACE('',#11309,2.);
#10202=CYLINDRICAL_SURFACE('',#11312,2.);
#10203=CYLINDRICAL_SURFACE('',#11335,3.5);
#10204=CYLINDRICAL_SURFACE('',#11338,2.);
#10205=CYLINDRICAL_SURFACE('',#11340,2.);
#10206=CYLINDRICAL_SURFACE('',#11343,2.);
#10207=CYLINDRICAL_SURFACE('',#11346,1.5);
#10208=CYLINDRICAL_SURFACE('',#11348,1.5);
#10209=CYLINDRICAL_SURFACE('',#11359,0.999999999999999);
#10210=CYLINDRICAL_SURFACE('',#11361,0.999999999999999);
#10211=CYLINDRICAL_SURFACE('',#11369,3.);
#10212=CYLINDRICAL_SURFACE('',#11372,3.);
#10213=CYLINDRICAL_SURFACE('',#11375,3.);
#10214=CYLINDRICAL_SURFACE('',#11380,3.);
#10215=CYLINDRICAL_SURFACE('',#11385,3.);
#10216=CYLINDRICAL_SURFACE('',#11388,3.);
#10217=CYLINDRICAL_SURFACE('',#11394,2.35);
#10218=CYLINDRICAL_SURFACE('',#11397,0.999999999999999);
#10219=CYLINDRICAL_SURFACE('',#11400,0.999999999999999);
#10220=CYLINDRICAL_SURFACE('',#11403,2.35);
#10221=CYLINDRICAL_SURFACE('',#11406,1.);
#10222=CYLINDRICAL_SURFACE('',#11409,1.);
#10223=CYLINDRICAL_SURFACE('',#11412,2.35);
#10224=CYLINDRICAL_SURFACE('',#11415,0.999999999999999);
#10225=CYLINDRICAL_SURFACE('',#11418,0.999999999999999);
#10226=CYLINDRICAL_SURFACE('',#11421,2.35);
#10227=CYLINDRICAL_SURFACE('',#11438,3.);
#10228=CYLINDRICAL_SURFACE('',#11441,3.);
#10229=CYLINDRICAL_SURFACE('',#11446,3.);
#10230=CYLINDRICAL_SURFACE('',#11451,3.);
#10231=CYLINDRICAL_SURFACE('',#11454,3.);
#10232=CYLINDRICAL_SURFACE('',#11456,3.);
#10233=CYLINDRICAL_SURFACE('',#11464,2.);
#10234=CYLINDRICAL_SURFACE('',#11521,1.5);
#10235=CYLINDRICAL_SURFACE('',#11525,1.5);
#10236=CYLINDRICAL_SURFACE('',#11527,1.5);
#10237=CYLINDRICAL_SURFACE('',#11530,1.5);
#10238=CYLINDRICAL_SURFACE('',#11535,1.5);
#10239=CYLINDRICAL_SURFACE('',#11537,1.5);
#10240=CYLINDRICAL_SURFACE('',#11540,1.5);
#10241=CYLINDRICAL_SURFACE('',#11545,1.5);
#10242=CYLINDRICAL_SURFACE('',#11547,1.5);
#10243=CYLINDRICAL_SURFACE('',#11550,1.5);
#10244=CYLINDRICAL_SURFACE('',#11555,1.5);
#10245=CYLINDRICAL_SURFACE('',#11584,2.);
#10403=ADVANCED_FACE('',(#951),#10174,.T.);
#10404=ADVANCED_FACE('',(#952),#10175,.T.);
#10405=ADVANCED_FACE('',(#953),#10176,.F.);
#10406=ADVANCED_FACE('',(#954),#10177,.F.);
#10407=ADVANCED_FACE('',(#955),#10178,.F.);
#10408=ADVANCED_FACE('',(#956),#10179,.F.);
#10409=ADVANCED_FACE('',(#957),#10180,.F.);
#10410=ADVANCED_FACE('',(#958),#10181,.F.);
#10411=ADVANCED_FACE('',(#959),#10182,.F.);
#10412=ADVANCED_FACE('',(#960),#10183,.F.);
#10413=ADVANCED_FACE('',(#961),#10184,.F.);
#10414=ADVANCED_FACE('',(#962),#10185,.F.);
#10415=ADVANCED_FACE('',(#963),#10186,.F.);
#10416=ADVANCED_FACE('',(#964),#10187,.F.);
#10417=ADVANCED_FACE('',(#965),#10188,.T.);
#10418=ADVANCED_FACE('',(#966),#10189,.F.);
#10419=ADVANCED_FACE('',(#967),#10190,.T.);
#10420=ADVANCED_FACE('',(#968),#10191,.T.);
#10421=ADVANCED_FACE('',(#969),#10192,.T.);
#10422=ADVANCED_FACE('',(#970),#10193,.T.);
#10423=ADVANCED_FACE('',(#971),#10194,.T.);
#10424=ADVANCED_FACE('',(#972),#10195,.T.);
#10425=ADVANCED_FACE('',(#973,#414),#598,.T.);
#10426=ADVANCED_FACE('',(#974),#10196,.T.);
#10427=ADVANCED_FACE('',(#975),#10197,.T.);
#10428=ADVANCED_FACE('',(#976),#10198,.T.);
#10429=ADVANCED_FACE('',(#977),#10199,.T.);
#10430=ADVANCED_FACE('',(#978,#415),#599,.F.);
#10431=ADVANCED_FACE('',(#979),#600,.T.);
#10432=ADVANCED_FACE('',(#980),#292,.F.);
#10433=ADVANCED_FACE('',(#981),#293,.F.);
#10434=ADVANCED_FACE('',(#982),#601,.T.);
#10435=ADVANCED_FACE('',(#983),#244,.T.);
#10436=ADVANCED_FACE('',(#984),#602,.T.);
#10437=ADVANCED_FACE('',(#985),#245,.T.);
#10438=ADVANCED_FACE('',(#986),#603,.T.);
#10439=ADVANCED_FACE('',(#987),#10200,.T.);
#10440=ADVANCED_FACE('',(#988),#10201,.T.);
#10441=ADVANCED_FACE('',(#989),#10202,.T.);
#10442=ADVANCED_FACE('',(#990,#416,#417,#418,#419,#420,#421),#604,.F.);
#10443=ADVANCED_FACE('',(#991),#10203,.T.);
#10444=ADVANCED_FACE('',(#992),#10204,.T.);
#10445=ADVANCED_FACE('',(#993),#10205,.T.);
#10446=ADVANCED_FACE('',(#994),#10206,.T.);
#10447=ADVANCED_FACE('',(#995),#10207,.T.);
#10448=ADVANCED_FACE('',(#996),#10208,.T.);
#10449=ADVANCED_FACE('',(#997,#422,#423,#424,#425,#426,#427),#605,.T.);
#10450=ADVANCED_FACE('',(#998),#10209,.T.);
#10451=ADVANCED_FACE('',(#999),#232,.T.);
#10452=ADVANCED_FACE('',(#1000),#10210,.T.);
#10453=ADVANCED_FACE('',(#1001),#233,.T.);
#10454=ADVANCED_FACE('',(#1002,#428),#606,.F.);
#10455=ADVANCED_FACE('',(#1003),#607,.T.);
#10456=ADVANCED_FACE('',(#1004),#608,.F.);
#10457=ADVANCED_FACE('',(#1005),#609,.T.);
#10458=ADVANCED_FACE('',(#1006),#610,.T.);
#10459=ADVANCED_FACE('',(#1007),#611,.F.);
#10460=ADVANCED_FACE('',(#1008),#10211,.T.);
#10461=ADVANCED_FACE('',(#1009),#612,.F.);
#10462=ADVANCED_FACE('',(#1010),#10212,.T.);
#10463=ADVANCED_FACE('',(#1011),#613,.F.);
#10464=ADVANCED_FACE('',(#1012),#10213,.T.);
#10465=ADVANCED_FACE('',(#1013),#614,.F.);
#10466=ADVANCED_FACE('',(#1014),#10214,.T.);
#10467=ADVANCED_FACE('',(#1015),#615,.F.);
#10468=ADVANCED_FACE('',(#1016),#10215,.T.);
#10469=ADVANCED_FACE('',(#1017),#616,.F.);
#10470=ADVANCED_FACE('',(#1018),#10216,.T.);
#10471=ADVANCED_FACE('',(#1019),#223,.T.);
#10472=ADVANCED_FACE('',(#1020),#617,.F.);
#10473=ADVANCED_FACE('',(#1021),#10217,.F.);
#10474=ADVANCED_FACE('',(#1022),#618,.F.);
#10475=ADVANCED_FACE('',(#1023),#10218,.T.);
#10476=ADVANCED_FACE('',(#1024),#619,.T.);
#10477=ADVANCED_FACE('',(#1025),#10219,.T.);
#10478=ADVANCED_FACE('',(#1026),#620,.F.);
#10479=ADVANCED_FACE('',(#1027),#10220,.F.);
#10480=ADVANCED_FACE('',(#1028),#621,.F.);
#10481=ADVANCED_FACE('',(#1029),#10221,.T.);
#10482=ADVANCED_FACE('',(#1030),#622,.T.);
#10483=ADVANCED_FACE('',(#1031),#10222,.T.);
#10484=ADVANCED_FACE('',(#1032),#623,.F.);
#10485=ADVANCED_FACE('',(#1033),#10223,.F.);
#10486=ADVANCED_FACE('',(#1034),#624,.F.);
#10487=ADVANCED_FACE('',(#1035),#10224,.T.);
#10488=ADVANCED_FACE('',(#1036),#625,.T.);
#10489=ADVANCED_FACE('',(#1037),#10225,.T.);
#10490=ADVANCED_FACE('',(#1038),#626,.F.);
#10491=ADVANCED_FACE('',(#1039),#10226,.F.);
#10492=ADVANCED_FACE('',(#1040),#627,.F.);
#10493=ADVANCED_FACE('',(#1041),#224,.T.);
#10494=ADVANCED_FACE('',(#1042),#628,.F.);
#10495=ADVANCED_FACE('',(#1043,#429),#629,.F.);
#10496=ADVANCED_FACE('',(#1044),#630,.T.);
#10497=ADVANCED_FACE('',(#1045),#631,.F.);
#10498=ADVANCED_FACE('',(#1046),#632,.T.);
#10499=ADVANCED_FACE('',(#1047),#633,.T.);
#10500=ADVANCED_FACE('',(#1048),#634,.T.);
#10501=ADVANCED_FACE('',(#1049),#10227,.T.);
#10502=ADVANCED_FACE('',(#1050),#635,.T.);
#10503=ADVANCED_FACE('',(#1051),#10228,.T.);
#10504=ADVANCED_FACE('',(#1052),#636,.T.);
#10505=ADVANCED_FACE('',(#1053),#10229,.T.);
#10506=ADVANCED_FACE('',(#1054),#637,.T.);
#10507=ADVANCED_FACE('',(#1055),#10230,.T.);
#10508=ADVANCED_FACE('',(#1056),#638,.T.);
#10509=ADVANCED_FACE('',(#1057),#10231,.T.);
#10510=ADVANCED_FACE('',(#1058),#10232,.T.);
#10511=ADVANCED_FACE('',(#1059),#639,.F.);
#10512=ADVANCED_FACE('',(#1060),#640,.F.);
#10513=ADVANCED_FACE('',(#1061),#641,.T.);
#10514=ADVANCED_FACE('',(#1062),#642,.T.);
#10515=ADVANCED_FACE('',(#1063),#643,.F.);
#10516=ADVANCED_FACE('',(#1064),#10233,.T.);
#10517=ADVANCED_FACE('',(#1065),#644,.T.);
#10518=ADVANCED_FACE('',(#1066),#645,.F.);
#10519=ADVANCED_FACE('',(#1067),#646,.F.);
#10520=ADVANCED_FACE('',(#1068),#647,.T.);
#10521=ADVANCED_FACE('',(#1069),#648,.T.);
#10522=ADVANCED_FACE('',(#1070),#649,.F.);
#10523=ADVANCED_FACE('',(#1071),#650,.F.);
#10524=ADVANCED_FACE('',(#1072),#651,.F.);
#10525=ADVANCED_FACE('',(#1073),#652,.T.);
#10526=ADVANCED_FACE('',(#1074),#653,.T.);
#10527=ADVANCED_FACE('',(#1075),#654,.T.);
#10528=ADVANCED_FACE('',(#1076),#655,.T.);
#10529=ADVANCED_FACE('',(#1077),#656,.F.);
#10530=ADVANCED_FACE('',(#1078),#657,.T.);
#10531=ADVANCED_FACE('',(#1079),#658,.F.);
#10532=ADVANCED_FACE('',(#1080),#659,.T.);
#10533=ADVANCED_FACE('',(#1081),#660,.T.);
#10534=ADVANCED_FACE('',(#1082),#661,.T.);
#10535=ADVANCED_FACE('',(#1083),#662,.F.);
#10536=ADVANCED_FACE('',(#1084),#663,.F.);
#10537=ADVANCED_FACE('',(#1085),#664,.F.);
#10538=ADVANCED_FACE('',(#1086),#665,.T.);
#10539=ADVANCED_FACE('',(#1087),#666,.F.);
#10540=ADVANCED_FACE('',(#1088),#667,.T.);
#10541=ADVANCED_FACE('',(#1089),#668,.F.);
#10542=ADVANCED_FACE('',(#1090),#669,.F.);
#10543=ADVANCED_FACE('',(#1091),#670,.F.);
#10544=ADVANCED_FACE('',(#1092),#671,.T.);
#10545=ADVANCED_FACE('',(#1093),#672,.F.);
#10546=ADVANCED_FACE('',(#1094),#673,.T.);
#10547=ADVANCED_FACE('',(#1095),#674,.T.);
#10548=ADVANCED_FACE('',(#1096,#430),#675,.F.);
#10549=ADVANCED_FACE('',(#1097,#431),#676,.F.);
#10550=ADVANCED_FACE('',(#1098,#432),#677,.F.);
#10551=ADVANCED_FACE('',(#1099,#433),#678,.F.);
#10552=ADVANCED_FACE('',(#1100,#434),#679,.F.);
#10553=ADVANCED_FACE('',(#1101,#435),#680,.F.);
#10554=ADVANCED_FACE('',(#1102),#681,.T.);
#10555=ADVANCED_FACE('',(#1103),#682,.F.);
#10556=ADVANCED_FACE('',(#1104),#683,.T.);
#10557=ADVANCED_FACE('',(#1105),#684,.F.);
#10558=ADVANCED_FACE('',(#1106),#685,.T.);
#10559=ADVANCED_FACE('',(#1107),#686,.T.);
#10560=ADVANCED_FACE('',(#1108),#687,.F.);
#10561=ADVANCED_FACE('',(#1109),#688,.T.);
#10562=ADVANCED_FACE('',(#1110),#689,.F.);
#10563=ADVANCED_FACE('',(#1111),#690,.T.);
#10564=ADVANCED_FACE('',(#1112),#691,.F.);
#10565=ADVANCED_FACE('',(#1113),#692,.T.);
#10566=ADVANCED_FACE('',(#1114),#693,.F.);
#10567=ADVANCED_FACE('',(#1115),#694,.T.);
#10568=ADVANCED_FACE('',(#1116),#695,.F.);
#10569=ADVANCED_FACE('',(#1117),#696,.T.);
#10570=ADVANCED_FACE('',(#1118),#697,.T.);
#10571=ADVANCED_FACE('',(#1119),#698,.T.);
#10572=ADVANCED_FACE('',(#1120),#10234,.T.);
#10573=ADVANCED_FACE('',(#1121),#225,.T.);
#10574=ADVANCED_FACE('',(#1122),#10235,.T.);
#10575=ADVANCED_FACE('',(#1123),#10236,.T.);
#10576=ADVANCED_FACE('',(#1124),#10237,.T.);
#10577=ADVANCED_FACE('',(#1125),#226,.T.);
#10578=ADVANCED_FACE('',(#1126),#10238,.T.);
#10579=ADVANCED_FACE('',(#1127),#10239,.T.);
#10580=ADVANCED_FACE('',(#1128),#10240,.T.);
#10581=ADVANCED_FACE('',(#1129),#227,.T.);
#10582=ADVANCED_FACE('',(#1130),#10241,.T.);
#10583=ADVANCED_FACE('',(#1131),#10242,.T.);
#10584=ADVANCED_FACE('',(#1132),#10243,.T.);
#10585=ADVANCED_FACE('',(#1133),#228,.T.);
#10586=ADVANCED_FACE('',(#1134),#10244,.T.);
#10587=ADVANCED_FACE('',(#1135),#699,.F.);
#10588=ADVANCED_FACE('',(#1136),#700,.T.);
#10589=ADVANCED_FACE('',(#1137),#701,.T.);
#10590=ADVANCED_FACE('',(#1138),#702,.T.);
#10591=ADVANCED_FACE('',(#1139),#703,.F.);
#10592=ADVANCED_FACE('',(#1140),#704,.T.);
#10593=ADVANCED_FACE('',(#1141),#705,.F.);
#10594=ADVANCED_FACE('',(#1142),#706,.F.);
#10595=ADVANCED_FACE('',(#1143),#707,.F.);
#10596=ADVANCED_FACE('',(#1144),#708,.T.);
#10597=ADVANCED_FACE('',(#1145),#709,.F.);
#10598=ADVANCED_FACE('',(#1146),#710,.T.);
#10599=ADVANCED_FACE('',(#1147),#711,.F.);
#10600=ADVANCED_FACE('',(#1148),#712,.F.);
#10601=ADVANCED_FACE('',(#1149),#713,.F.);
#10602=ADVANCED_FACE('',(#1150),#714,.T.);
#10603=ADVANCED_FACE('',(#1151),#715,.T.);
#10604=ADVANCED_FACE('',(#1152),#716,.T.);
#10605=ADVANCED_FACE('',(#1153),#717,.T.);
#10606=ADVANCED_FACE('',(#1154),#718,.T.);
#10607=ADVANCED_FACE('',(#1155),#719,.T.);
#10608=ADVANCED_FACE('',(#1156),#720,.F.);
#10609=ADVANCED_FACE('',(#1157),#721,.F.);
#10610=ADVANCED_FACE('',(#1158),#722,.F.);
#10611=ADVANCED_FACE('',(#1159),#723,.T.);
#10612=ADVANCED_FACE('',(#1160),#724,.F.);
#10613=ADVANCED_FACE('',(#1161),#725,.T.);
#10614=ADVANCED_FACE('',(#1162),#10245,.T.);
#10615=ADVANCED_FACE('',(#1163),#726,.F.);
#10616=ADVANCED_FACE('',(#1164),#727,.T.);
#10617=ADVANCED_FACE('',(#1165),#728,.T.);
#10618=ADVANCED_FACE('',(#1166),#729,.F.);
#10619=ADVANCED_FACE('',(#1167,#436),#730,.T.);
#10620=ADVANCED_FACE('',(#1168,#437),#731,.T.);
#10621=ADVANCED_FACE('',(#1169,#438),#732,.T.);
#10622=ADVANCED_FACE('',(#1170,#439),#733,.T.);
#10623=ADVANCED_FACE('',(#1171,#440),#734,.T.);
#10624=ADVANCED_FACE('',(#1172,#441),#735,.T.);
#10625=ADVANCED_FACE('',(#1173),#736,.F.);
#10626=ADVANCED_FACE('',(#1174),#737,.F.);
#10627=ADVANCED_FACE('',(#1175),#738,.F.);
#10628=ADVANCED_FACE('',(#1176),#739,.F.);
#10629=ADVANCED_FACE('',(#1177),#740,.T.);
#10630=ADVANCED_FACE('',(#1178),#741,.F.);
#10631=ADVANCED_FACE('',(#1179),#742,.T.);
#10632=ADVANCED_FACE('',(#1180),#743,.F.);
#10633=ADVANCED_FACE('',(#1181),#744,.F.);
#10634=ADVANCED_FACE('',(#1182),#745,.F.);
#10635=ADVANCED_FACE('',(#1183),#746,.F.);
#10636=ADVANCED_FACE('',(#1184,#442),#747,.F.);
#10637=ADVANCED_FACE('',(#1185),#748,.F.);
#10638=ADVANCED_FACE('',(#1186),#749,.F.);
#10639=ADVANCED_FACE('',(#1187),#750,.F.);
#10640=ADVANCED_FACE('',(#1188),#751,.T.);
#10641=ADVANCED_FACE('',(#1189),#752,.T.);
#10642=ADVANCED_FACE('',(#1190),#753,.T.);
#10643=ADVANCED_FACE('',(#1191),#754,.T.);
#10644=ADVANCED_FACE('',(#1192,#443),#755,.F.);
#10645=ADVANCED_FACE('',(#1193),#756,.F.);
#10646=ADVANCED_FACE('',(#1194),#757,.T.);
#10647=ADVANCED_FACE('',(#1195),#758,.T.);
#10648=ADVANCED_FACE('',(#1196),#759,.T.);
#10649=ADVANCED_FACE('',(#1197),#760,.T.);
#10650=ADVANCED_FACE('',(#1198),#761,.F.);
#10651=ADVANCED_FACE('',(#1199),#762,.F.);
#10652=ADVANCED_FACE('',(#1200),#763,.F.);
#10653=ADVANCED_FACE('',(#1201),#764,.T.);
#10654=ADVANCED_FACE('',(#1202),#765,.T.);
#10655=ADVANCED_FACE('',(#1203),#766,.T.);
#10656=ADVANCED_FACE('',(#1204),#767,.T.);
#10657=ADVANCED_FACE('',(#1205),#768,.T.);
#10658=ADVANCED_FACE('',(#1206),#769,.T.);
#10659=ADVANCED_FACE('',(#1207),#770,.T.);
#10660=ADVANCED_FACE('',(#1208),#771,.T.);
#10661=ADVANCED_FACE('',(#1209),#772,.T.);
#10662=ADVANCED_FACE('',(#1210),#773,.T.);
#10663=ADVANCED_FACE('',(#1211),#774,.T.);
#10664=ADVANCED_FACE('',(#1212),#246,.T.);
#10665=ADVANCED_FACE('',(#1213),#247,.T.);
#10666=ADVANCED_FACE('',(#1214),#248,.T.);
#10667=ADVANCED_FACE('',(#1215),#249,.T.);
#10668=ADVANCED_FACE('',(#1216),#250,.T.);
#10669=ADVANCED_FACE('',(#1217),#251,.T.);
#10670=ADVANCED_FACE('',(#1218,#444),#775,.F.);
#10671=ADVANCED_FACE('',(#1219),#776,.F.);
#10672=ADVANCED_FACE('',(#1220),#777,.F.);
#10673=ADVANCED_FACE('',(#1221),#778,.F.);
#10674=ADVANCED_FACE('',(#1222),#779,.F.);
#10675=ADVANCED_FACE('',(#1223,#445),#780,.F.);
#10676=ADVANCED_FACE('',(#1224),#781,.F.);
#10677=ADVANCED_FACE('',(#1225),#782,.F.);
#10678=ADVANCED_FACE('',(#1226),#783,.F.);
#10679=ADVANCED_FACE('',(#1227),#784,.F.);
#10680=ADVANCED_FACE('',(#1228),#785,.F.);
#10681=ADVANCED_FACE('',(#1229),#786,.F.);
#10682=ADVANCED_FACE('',(#1230),#787,.F.);
#10683=ADVANCED_FACE('',(#1231),#788,.F.);
#10684=ADVANCED_FACE('',(#1232),#789,.T.);
#10685=ADVANCED_FACE('',(#1233),#790,.T.);
#10686=ADVANCED_FACE('',(#1234),#791,.F.);
#10687=ADVANCED_FACE('',(#1235),#792,.T.);
#10688=ADVANCED_FACE('',(#1236),#793,.T.);
#10689=ADVANCED_FACE('',(#1237),#794,.T.);
#10690=ADVANCED_FACE('',(#1238),#795,.T.);
#10691=ADVANCED_FACE('',(#1239),#234,.T.);
#10692=ADVANCED_FACE('',(#1240),#235,.T.);
#10693=ADVANCED_FACE('',(#1241),#236,.T.);
#10694=ADVANCED_FACE('',(#1242),#237,.T.);
#10695=ADVANCED_FACE('',(#1243),#238,.T.);
#10696=ADVANCED_FACE('',(#1244),#239,.T.);
#10697=ADVANCED_FACE('',(#1245),#796,.T.);
#10698=ADVANCED_FACE('',(#1246),#797,.T.);
#10699=ADVANCED_FACE('',(#1247),#798,.T.);
#10700=ADVANCED_FACE('',(#1248),#799,.T.);
#10701=ADVANCED_FACE('',(#1249),#800,.F.);
#10702=ADVANCED_FACE('',(#1250),#801,.T.);
#10703=ADVANCED_FACE('',(#1251,#446),#802,.F.);
#10704=ADVANCED_FACE('',(#1252),#803,.T.);
#10705=ADVANCED_FACE('',(#1253,#447),#804,.F.);
#10706=ADVANCED_FACE('',(#1254,#448),#805,.T.);
#10707=ADVANCED_FACE('',(#1255,#449),#806,.T.);
#10708=ADVANCED_FACE('',(#1256),#807,.T.);
#10945=CLOSED_SHELL('',(#10403,#10404,#10405,#10406,#10407,#10408,#10409,
#10410,#10411,#10412,#10413,#10414,#10415,#10416,#10417,#10418,#10419,#10420,
#10421,#10422,#10423,#10424,#10425,#10426,#10427,#10428,#10429,#10430,#10431,
#10432,#10433,#10434,#10435,#10436,#10437,#10438,#10439,#10440,#10441,#10442,
#10443,#10444,#10445,#10446,#10447,#10448,#10449,#10450,#10451,#10452,#10453,
#10454,#10455,#10456,#10457,#10458,#10459,#10460,#10461,#10462,#10463,#10464,
#10465,#10466,#10467,#10468,#10469,#10470,#10471,#10472,#10473,#10474,#10475,
#10476,#10477,#10478,#10479,#10480,#10481,#10482,#10483,#10484,#10485,#10486,
#10487,#10488,#10489,#10490,#10491,#10492,#10493,#10494,#10495,#10496,#10497,
#10498,#10499,#10500,#10501,#10502,#10503,#10504,#10505,#10506,#10507,#10508,
#10509,#10510,#10511,#10512,#10513,#10514,#10515,#10516,#10517,#10518,#10519,
#10520,#10521,#10522,#10523,#10524,#10525,#10526,#10527,#10528,#10529,#10530,
#10531,#10532,#10533,#10534,#10535,#10536,#10537,#10538,#10539,#10540,#10541,
#10542,#10543,#10544,#10545,#10546,#10547,#10548,#10549,#10550,#10551,#10552,
#10553,#10554,#10555,#10556,#10557,#10558,#10559,#10560,#10561,#10562,#10563,
#10564,#10565,#10566,#10567,#10568,#10569,#10570,#10571,#10572,#10573,#10574,
#10575,#10576,#10577,#10578,#10579,#10580,#10581,#10582,#10583,#10584,#10585,
#10586,#10587,#10588,#10589,#10590,#10591,#10592,#10593,#10594,#10595,#10596,
#10597,#10598,#10599,#10600,#10601,#10602,#10603,#10604,#10605,#10606,#10607,
#10608,#10609,#10610,#10611,#10612,#10613,#10614,#10615,#10616,#10617,#10618,
#10619,#10620,#10621,#10622,#10623,#10624,#10625,#10626,#10627,#10628,#10629,
#10630,#10631,#10632,#10633,#10634,#10635,#10636,#10637,#10638,#10639,#10640,
#10641,#10642,#10643,#10644,#10645,#10646,#10647,#10648,#10649,#10650,#10651,
#10652,#10653,#10654,#10655,#10656,#10657,#10658,#10659,#10660,#10661,#10662,
#10663,#10664,#10665,#10666,#10667,#10668,#10669,#10670,#10671,#10672,#10673,
#10674,#10675,#10676,#10677,#10678,#10679,#10680,#10681,#10682,#10683,#10684,
#10685,#10686,#10687,#10688,#10689,#10690,#10691,#10692,#10693,#10694,#10695,
#10696,#10697,#10698,#10699,#10700,#10701,#10702,#10703,#10704,#10705,#10706,
#10707,#10708));
#11215=AXIS2_PLACEMENT_3D('',#15688,#12509,#12510);
#11216=AXIS2_PLACEMENT_3D('',#15689,#12511,#12512);
#11217=AXIS2_PLACEMENT_3D('',#15691,#12513,#12514);
#11218=AXIS2_PLACEMENT_3D('',#15694,#12516,#12517);
#11219=AXIS2_PLACEMENT_3D('',#15695,#12518,#12519);
#11220=AXIS2_PLACEMENT_3D('',#15697,#12520,#12521);
#11221=AXIS2_PLACEMENT_3D('',#15700,#12523,#12524);
#11222=AXIS2_PLACEMENT_3D('',#15701,#12525,#12526);
#11223=AXIS2_PLACEMENT_3D('',#15703,#12527,#12528);
#11224=AXIS2_PLACEMENT_3D('',#15706,#12530,#12531);
#11225=AXIS2_PLACEMENT_3D('',#15707,#12532,#12533);
#11226=AXIS2_PLACEMENT_3D('',#15709,#12534,#12535);
#11227=AXIS2_PLACEMENT_3D('',#15712,#12537,#12538);
#11228=AXIS2_PLACEMENT_3D('',#15713,#12539,#12540);
#11229=AXIS2_PLACEMENT_3D('',#15715,#12541,#12542);
#11230=AXIS2_PLACEMENT_3D('',#15718,#12544,#12545);
#11231=AXIS2_PLACEMENT_3D('',#15719,#12546,#12547);
#11232=AXIS2_PLACEMENT_3D('',#15721,#12548,#12549);
#11233=AXIS2_PLACEMENT_3D('',#15724,#12551,#12552);
#11234=AXIS2_PLACEMENT_3D('',#15725,#12553,#12554);
#11235=AXIS2_PLACEMENT_3D('',#15727,#12555,#12556);
#11236=AXIS2_PLACEMENT_3D('',#15730,#12558,#12559);
#11237=AXIS2_PLACEMENT_3D('',#15731,#12560,#12561);
#11238=AXIS2_PLACEMENT_3D('',#15733,#12562,#12563);
#11239=AXIS2_PLACEMENT_3D('',#15736,#12565,#12566);
#11240=AXIS2_PLACEMENT_3D('',#15737,#12567,#12568);
#11241=AXIS2_PLACEMENT_3D('',#15739,#12569,#12570);
#11242=AXIS2_PLACEMENT_3D('',#15742,#12572,#12573);
#11243=AXIS2_PLACEMENT_3D('',#15743,#12574,#12575);
#11244=AXIS2_PLACEMENT_3D('',#15745,#12576,#12577);
#11245=AXIS2_PLACEMENT_3D('',#15748,#12579,#12580);
#11246=AXIS2_PLACEMENT_3D('',#15749,#12581,#12582);
#11247=AXIS2_PLACEMENT_3D('',#15751,#12583,#12584);
#11248=AXIS2_PLACEMENT_3D('',#15754,#12586,#12587);
#11249=AXIS2_PLACEMENT_3D('',#15755,#12588,#12589);
#11250=AXIS2_PLACEMENT_3D('',#15757,#12590,#12591);
#11251=AXIS2_PLACEMENT_3D('',#15760,#12593,#12594);
#11252=AXIS2_PLACEMENT_3D('',#15761,#12595,#12596);
#11253=AXIS2_PLACEMENT_3D('',#15763,#12597,#12598);
#11254=AXIS2_PLACEMENT_3D('',#15766,#12600,#12601);
#11255=AXIS2_PLACEMENT_3D('',#15767,#12602,#12603);
#11256=AXIS2_PLACEMENT_3D('',#15769,#12604,#12605);
#11257=AXIS2_PLACEMENT_3D('',#15772,#12607,#12608);
#11258=AXIS2_PLACEMENT_3D('',#15773,#12609,#12610);
#11259=AXIS2_PLACEMENT_3D('',#15775,#12611,#12612);
#11260=AXIS2_PLACEMENT_3D('',#15778,#12614,#12615);
#11261=AXIS2_PLACEMENT_3D('',#15779,#12616,#12617);
#11262=AXIS2_PLACEMENT_3D('',#15781,#12618,#12619);
#11263=AXIS2_PLACEMENT_3D('',#15784,#12621,#12622);
#11264=AXIS2_PLACEMENT_3D('',#15785,#12623,#12624);
#11265=AXIS2_PLACEMENT_3D('',#15787,#12625,#12626);
#11266=AXIS2_PLACEMENT_3D('',#15790,#12628,#12629);
#11267=AXIS2_PLACEMENT_3D('',#15791,#12630,#12631);
#11268=AXIS2_PLACEMENT_3D('',#15793,#12632,#12633);
#11269=AXIS2_PLACEMENT_3D('',#15796,#12635,#12636);
#11270=AXIS2_PLACEMENT_3D('',#15797,#12637,#12638);
#11271=AXIS2_PLACEMENT_3D('',#15799,#12639,#12640);
#11272=AXIS2_PLACEMENT_3D('',#15802,#12642,#12643);
#11273=AXIS2_PLACEMENT_3D('',#15803,#12644,#12645);
#11274=AXIS2_PLACEMENT_3D('',#15805,#12646,#12647);
#11275=AXIS2_PLACEMENT_3D('',#15808,#12649,#12650);
#11276=AXIS2_PLACEMENT_3D('',#15809,#12651,#12652);
#11277=AXIS2_PLACEMENT_3D('',#15811,#12653,#12654);
#11278=AXIS2_PLACEMENT_3D('',#15814,#12656,#12657);
#11279=AXIS2_PLACEMENT_3D('',#15815,#12658,#12659);
#11280=AXIS2_PLACEMENT_3D('',#15817,#12660,#12661);
#11281=AXIS2_PLACEMENT_3D('',#15820,#12663,#12664);
#11282=AXIS2_PLACEMENT_3D('',#15821,#12665,#12666);
#11283=AXIS2_PLACEMENT_3D('',#15830,#12671,#12672);
#11284=AXIS2_PLACEMENT_3D('',#15832,#12673,#12674);
#11285=AXIS2_PLACEMENT_3D('',#15835,#12676,#12677);
#11286=AXIS2_PLACEMENT_3D('',#15836,#12678,#12679);
#11287=AXIS2_PLACEMENT_3D('',#15840,#12681,#12682);
#11288=AXIS2_PLACEMENT_3D('',#15841,#12683,#12684);
#11289=AXIS2_PLACEMENT_3D('',#15842,#12685,#12686);
#11290=AXIS2_PLACEMENT_3D('',#15846,#12688,#12689);
#11291=AXIS2_PLACEMENT_3D('',#15847,#12690,#12691);
#11292=AXIS2_PLACEMENT_3D('',#15848,#12692,#12693);
#11293=AXIS2_PLACEMENT_3D('',#15850,#12694,#12695);
#11294=AXIS2_PLACEMENT_3D('',#15853,#12697,#12698);
#11295=AXIS2_PLACEMENT_3D('',#15854,#12699,#12700);
#11296=AXIS2_PLACEMENT_3D('',#15855,#12701,#12702);
#11297=AXIS2_PLACEMENT_3D('',#15905,#12720,#12721);
#11298=AXIS2_PLACEMENT_3D('',#15906,#12722,#12723);
#11299=AXIS2_PLACEMENT_3D('',#15923,#12724,#12725);
#11300=AXIS2_PLACEMENT_3D('',#15924,#12726,#12727);
#11301=AXIS2_PLACEMENT_3D('',#15925,#12728,#12729);
#11302=AXIS2_PLACEMENT_3D('',#15936,#12733,#12734);
#11303=AXIS2_PLACEMENT_3D('',#16118,#12735,#12736);
#11304=AXIS2_PLACEMENT_3D('',#16182,#12740,#12741);
#11305=AXIS2_PLACEMENT_3D('',#16237,#12742,#12743);
#11306=AXIS2_PLACEMENT_3D('',#16296,#12747,#12748);
#11307=AXIS2_PLACEMENT_3D('',#16300,#12750,#12751);
#11308=AXIS2_PLACEMENT_3D('',#16301,#12752,#12753);
#11309=AXIS2_PLACEMENT_3D('',#16302,#12754,#12755);
#11310=AXIS2_PLACEMENT_3D('',#16306,#12757,#12758);
#11311=AXIS2_PLACEMENT_3D('',#16307,#12759,#12760);
#11312=AXIS2_PLACEMENT_3D('',#16308,#12761,#12762);
#11313=AXIS2_PLACEMENT_3D('',#16312,#12764,#12765);
#11314=AXIS2_PLACEMENT_3D('',#16313,#12766,#12767);
#11315=AXIS2_PLACEMENT_3D('',#16314,#12768,#12769);
#11316=AXIS2_PLACEMENT_3D('',#16319,#12771,#12772);
#11317=AXIS2_PLACEMENT_3D('',#16323,#12774,#12775);
#11318=AXIS2_PLACEMENT_3D('',#16327,#12777,#12778);
#11319=AXIS2_PLACEMENT_3D('',#16331,#12780,#12781);
#11320=AXIS2_PLACEMENT_3D('',#16335,#12783,#12784);
#11321=AXIS2_PLACEMENT_3D('',#16338,#12786,#12787);
#11322=AXIS2_PLACEMENT_3D('',#16342,#12789,#12790);
#11323=AXIS2_PLACEMENT_3D('',#16346,#12792,#12793);
#11324=AXIS2_PLACEMENT_3D('',#16350,#12795,#12796);
#11325=AXIS2_PLACEMENT_3D('',#16354,#12798,#12799);
#11326=AXIS2_PLACEMENT_3D('',#16358,#12801,#12802);
#11327=AXIS2_PLACEMENT_3D('',#16362,#12804,#12805);
#11328=AXIS2_PLACEMENT_3D('',#16366,#12807,#12808);
#11329=AXIS2_PLACEMENT_3D('',#16370,#12810,#12811);
#11330=AXIS2_PLACEMENT_3D('',#16374,#12813,#12814);
#11331=AXIS2_PLACEMENT_3D('',#16378,#12816,#12817);
#11332=AXIS2_PLACEMENT_3D('',#16381,#12819,#12820);
#11333=AXIS2_PLACEMENT_3D('',#16383,#12821,#12822);
#11334=AXIS2_PLACEMENT_3D('',#16386,#12824,#12825);
#11335=AXIS2_PLACEMENT_3D('',#16387,#12826,#12827);
#11336=AXIS2_PLACEMENT_3D('',#16389,#12828,#12829);
#11337=AXIS2_PLACEMENT_3D('',#16391,#12830,#12831);
#11338=AXIS2_PLACEMENT_3D('',#16393,#12833,#12834);
#11339=AXIS2_PLACEMENT_3D('',#16395,#12835,#12836);
#11340=AXIS2_PLACEMENT_3D('',#16397,#12838,#12839);
#11341=AXIS2_PLACEMENT_3D('',#16399,#12840,#12841);
#11342=AXIS2_PLACEMENT_3D('',#16402,#12843,#12844);
#11343=AXIS2_PLACEMENT_3D('',#16403,#12845,#12846);
#11344=AXIS2_PLACEMENT_3D('',#16405,#12847,#12848);
#11345=AXIS2_PLACEMENT_3D('',#16408,#12850,#12851);
#11346=AXIS2_PLACEMENT_3D('',#16409,#12852,#12853);
#11347=AXIS2_PLACEMENT_3D('',#16410,#12854,#12855);
#11348=AXIS2_PLACEMENT_3D('',#16411,#12856,#12857);
#11349=AXIS2_PLACEMENT_3D('',#16412,#12858,#12859);
#11350=AXIS2_PLACEMENT_3D('',#16413,#12860,#12861);
#11351=AXIS2_PLACEMENT_3D('',#16416,#12862,#12863);
#11352=AXIS2_PLACEMENT_3D('',#16420,#12865,#12866);
#11353=AXIS2_PLACEMENT_3D('',#16422,#12868,#12869);
#11354=AXIS2_PLACEMENT_3D('',#16423,#12870,#12871);
#11355=AXIS2_PLACEMENT_3D('',#16427,#12873,#12874);
#11356=AXIS2_PLACEMENT_3D('',#16431,#12876,#12877);
#11357=AXIS2_PLACEMENT_3D('',#16435,#12879,#12880);
#11358=AXIS2_PLACEMENT_3D('',#16439,#12882,#12883);
#11359=AXIS2_PLACEMENT_3D('',#16441,#12885,#12886);
#11360=AXIS2_PLACEMENT_3D('',#16442,#12887,#12888);
#11361=AXIS2_PLACEMENT_3D('',#16487,#12889,#12890);
#11362=AXIS2_PLACEMENT_3D('',#16488,#12891,#12892);
#11363=AXIS2_PLACEMENT_3D('',#16533,#12893,#12894);
#11364=AXIS2_PLACEMENT_3D('',#16534,#12895,#12896);
#11365=AXIS2_PLACEMENT_3D('',#16546,#12903,#12904);
#11366=AXIS2_PLACEMENT_3D('',#16550,#12907,#12908);
#11367=AXIS2_PLACEMENT_3D('',#16626,#12947,#12948);
#11368=AXIS2_PLACEMENT_3D('',#16630,#12951,#12952);
#11369=AXIS2_PLACEMENT_3D('',#16640,#12958,#12959);
#11370=AXIS2_PLACEMENT_3D('',#16644,#12961,#12962);
#11371=AXIS2_PLACEMENT_3D('',#16646,#12964,#12965);
#11372=AXIS2_PLACEMENT_3D('',#16674,#12980,#12981);
#11373=AXIS2_PLACEMENT_3D('',#16676,#12982,#12983);
#11374=AXIS2_PLACEMENT_3D('',#16678,#12985,#12986);
#11375=AXIS2_PLACEMENT_3D('',#16682,#12989,#12990);
#11376=AXIS2_PLACEMENT_3D('',#16685,#12991,#12992);
#11377=AXIS2_PLACEMENT_3D('',#16687,#12993,#12994);
#11378=AXIS2_PLACEMENT_3D('',#16689,#12996,#12997);
#11379=AXIS2_PLACEMENT_3D('',#16690,#12998,#12999);
#11380=AXIS2_PLACEMENT_3D('',#16710,#13010,#13011);
#11381=AXIS2_PLACEMENT_3D('',#16712,#13012,#13013);
#11382=AXIS2_PLACEMENT_3D('',#16714,#13014,#13015);
#11383=AXIS2_PLACEMENT_3D('',#16716,#13017,#13018);
#11384=AXIS2_PLACEMENT_3D('',#16717,#13019,#13020);
#11385=AXIS2_PLACEMENT_3D('',#16721,#13023,#13024);
#11386=AXIS2_PLACEMENT_3D('',#16723,#13025,#13026);
#11387=AXIS2_PLACEMENT_3D('',#16725,#13028,#13029);
#11388=AXIS2_PLACEMENT_3D('',#16753,#13044,#13045);
#11389=AXIS2_PLACEMENT_3D('',#16754,#13046,#13047);
#11390=AXIS2_PLACEMENT_3D('',#16755,#13048,#13049);
#11391=AXIS2_PLACEMENT_3D('',#16757,#13050,#13051);
#11392=AXIS2_PLACEMENT_3D('',#16758,#13052,#13053);
#11393=AXIS2_PLACEMENT_3D('',#16759,#13054,#13055);
#11394=AXIS2_PLACEMENT_3D('',#16763,#13058,#13059);
#11395=AXIS2_PLACEMENT_3D('',#16766,#13061,#13062);
#11396=AXIS2_PLACEMENT_3D('',#16767,#13063,#13064);
#11397=AXIS2_PLACEMENT_3D('',#16776,#13067,#13068);
#11398=AXIS2_PLACEMENT_3D('',#16778,#13069,#13070);
#11399=AXIS2_PLACEMENT_3D('',#16780,#13072,#13073);
#11400=AXIS2_PLACEMENT_3D('',#16794,#13076,#13077);
#11401=AXIS2_PLACEMENT_3D('',#16796,#13078,#13079);
#11402=AXIS2_PLACEMENT_3D('',#16798,#13081,#13082);
#11403=AXIS2_PLACEMENT_3D('',#16807,#13085,#13086);
#11404=AXIS2_PLACEMENT_3D('',#16810,#13088,#13089);
#11405=AXIS2_PLACEMENT_3D('',#16811,#13090,#13091);
#11406=AXIS2_PLACEMENT_3D('',#16820,#13094,#13095);
#11407=AXIS2_PLACEMENT_3D('',#16822,#13096,#13097);
#11408=AXIS2_PLACEMENT_3D('',#16824,#13099,#13100);
#11409=AXIS2_PLACEMENT_3D('',#16838,#13103,#13104);
#11410=AXIS2_PLACEMENT_3D('',#16840,#13105,#13106);
#11411=AXIS2_PLACEMENT_3D('',#16842,#13108,#13109);
#11412=AXIS2_PLACEMENT_3D('',#16851,#13112,#13113);
#11413=AXIS2_PLACEMENT_3D('',#16854,#13115,#13116);
#11414=AXIS2_PLACEMENT_3D('',#16855,#13117,#13118);
#11415=AXIS2_PLACEMENT_3D('',#16864,#13121,#13122);
#11416=AXIS2_PLACEMENT_3D('',#16866,#13123,#13124);
#11417=AXIS2_PLACEMENT_3D('',#16868,#13126,#13127);
#11418=AXIS2_PLACEMENT_3D('',#16882,#13130,#13131);
#11419=AXIS2_PLACEMENT_3D('',#16884,#13132,#13133);
#11420=AXIS2_PLACEMENT_3D('',#16886,#13135,#13136);
#11421=AXIS2_PLACEMENT_3D('',#16895,#13139,#13140);
#11422=AXIS2_PLACEMENT_3D('',#16898,#13142,#13143);
#11423=AXIS2_PLACEMENT_3D('',#16899,#13144,#13145);
#11424=AXIS2_PLACEMENT_3D('',#16902,#13147,#13148);
#11425=AXIS2_PLACEMENT_3D('',#16903,#13149,#13150);
#11426=AXIS2_PLACEMENT_3D('',#16904,#13151,#13152);
#11427=AXIS2_PLACEMENT_3D('',#16905,#13153,#13154);
#11428=AXIS2_PLACEMENT_3D('',#16915,#13160,#13161);
#11429=AXIS2_PLACEMENT_3D('',#16918,#13162,#13163);
#11430=AXIS2_PLACEMENT_3D('',#16926,#13167,#13168);
#11431=AXIS2_PLACEMENT_3D('',#16934,#13172,#13173);
#11432=AXIS2_PLACEMENT_3D('',#16942,#13177,#13178);
#11433=AXIS2_PLACEMENT_3D('',#16945,#13181,#13182);
#11434=AXIS2_PLACEMENT_3D('',#16949,#13185,#13186);
#11435=AXIS2_PLACEMENT_3D('',#16955,#13190,#13191);
#11436=AXIS2_PLACEMENT_3D('',#17028,#13229,#13230);
#11437=AXIS2_PLACEMENT_3D('',#17038,#13236,#13237);
#11438=AXIS2_PLACEMENT_3D('',#17068,#13253,#13254);
#11439=AXIS2_PLACEMENT_3D('',#17071,#13256,#13257);
#11440=AXIS2_PLACEMENT_3D('',#17072,#13258,#13259);
#11441=AXIS2_PLACEMENT_3D('',#17076,#13262,#13263);
#11442=AXIS2_PLACEMENT_3D('',#17080,#13265,#13266);
#11443=AXIS2_PLACEMENT_3D('',#17081,#13267,#13268);
#11444=AXIS2_PLACEMENT_3D('',#17082,#13269,#13270);
#11445=AXIS2_PLACEMENT_3D('',#17083,#13271,#13272);
#11446=AXIS2_PLACEMENT_3D('',#17103,#13283,#13284);
#11447=AXIS2_PLACEMENT_3D('',#17106,#13286,#13287);
#11448=AXIS2_PLACEMENT_3D('',#17108,#13288,#13289);
#11449=AXIS2_PLACEMENT_3D('',#17109,#13290,#13291);
#11450=AXIS2_PLACEMENT_3D('',#17110,#13292,#13293);
#11451=AXIS2_PLACEMENT_3D('',#17114,#13296,#13297);
#11452=AXIS2_PLACEMENT_3D('',#17117,#13299,#13300);
#11453=AXIS2_PLACEMENT_3D('',#17118,#13301,#13302);
#11454=AXIS2_PLACEMENT_3D('',#17146,#13317,#13318);
#11455=AXIS2_PLACEMENT_3D('',#17147,#13319,#13320);
#11456=AXIS2_PLACEMENT_3D('',#17148,#13321,#13322);
#11457=AXIS2_PLACEMENT_3D('',#17149,#13323,#13324);
#11458=AXIS2_PLACEMENT_3D('',#17150,#13325,#13326);
#11459=AXIS2_PLACEMENT_3D('',#17156,#13330,#13331);
#11460=AXIS2_PLACEMENT_3D('',#17159,#13334,#13335);
#11461=AXIS2_PLACEMENT_3D('',#17160,#13336,#13337);
#11462=AXIS2_PLACEMENT_3D('',#17165,#13341,#13342);
#11463=AXIS2_PLACEMENT_3D('',#17171,#13345,#13346);
#11464=AXIS2_PLACEMENT_3D('',#17173,#13348,#13349);
#11465=AXIS2_PLACEMENT_3D('',#17176,#13351,#13352);
#11466=AXIS2_PLACEMENT_3D('',#17177,#13353,#13354);
#11467=AXIS2_PLACEMENT_3D('',#17185,#13359,#13360);
#11468=AXIS2_PLACEMENT_3D('',#17188,#13363,#13364);
#11469=AXIS2_PLACEMENT_3D('',#17189,#13365,#13366);
#11470=AXIS2_PLACEMENT_3D('',#17195,#13370,#13371);
#11471=AXIS2_PLACEMENT_3D('',#17199,#13374,#13375);
#11472=AXIS2_PLACEMENT_3D('',#17205,#13379,#13380);
#11473=AXIS2_PLACEMENT_3D('',#17209,#13383,#13384);
#11474=AXIS2_PLACEMENT_3D('',#17213,#13387,#13388);
#11475=AXIS2_PLACEMENT_3D('',#17219,#13392,#13393);
#11476=AXIS2_PLACEMENT_3D('',#17226,#13398,#13399);
#11477=AXIS2_PLACEMENT_3D('',#17230,#13402,#13403);
#11478=AXIS2_PLACEMENT_3D('',#17235,#13407,#13408);
#11479=AXIS2_PLACEMENT_3D('',#17237,#13410,#13411);
#11480=AXIS2_PLACEMENT_3D('',#17239,#13413,#13414);
#11481=AXIS2_PLACEMENT_3D('',#17241,#13416,#13417);
#11482=AXIS2_PLACEMENT_3D('',#17245,#13420,#13421);
#11483=AXIS2_PLACEMENT_3D('',#17249,#13424,#13425);
#11484=AXIS2_PLACEMENT_3D('',#17254,#13429,#13430);
#11485=AXIS2_PLACEMENT_3D('',#17255,#13431,#13432);
#11486=AXIS2_PLACEMENT_3D('',#17259,#13435,#13436);
#11487=AXIS2_PLACEMENT_3D('',#17264,#13440,#13441);
#11488=AXIS2_PLACEMENT_3D('',#17266,#13443,#13444);
#11489=AXIS2_PLACEMENT_3D('',#17268,#13446,#13447);
#11490=AXIS2_PLACEMENT_3D('',#17270,#13449,#13450);
#11491=AXIS2_PLACEMENT_3D('',#17274,#13453,#13454);
#11492=AXIS2_PLACEMENT_3D('',#17278,#13457,#13458);
#11493=AXIS2_PLACEMENT_3D('',#17283,#13462,#13463);
#11494=AXIS2_PLACEMENT_3D('',#17285,#13465,#13466);
#11495=AXIS2_PLACEMENT_3D('',#17286,#13467,#13468);
#11496=AXIS2_PLACEMENT_3D('',#17287,#13469,#13470);
#11497=AXIS2_PLACEMENT_3D('',#17291,#13473,#13474);
#11498=AXIS2_PLACEMENT_3D('',#17299,#13479,#13480);
#11499=AXIS2_PLACEMENT_3D('',#17307,#13485,#13486);
#11500=AXIS2_PLACEMENT_3D('',#17315,#13491,#13492);
#11501=AXIS2_PLACEMENT_3D('',#17323,#13497,#13498);
#11502=AXIS2_PLACEMENT_3D('',#17331,#13503,#13504);
#11503=AXIS2_PLACEMENT_3D('',#17337,#13508,#13509);
#11504=AXIS2_PLACEMENT_3D('',#17341,#13512,#13513);
#11505=AXIS2_PLACEMENT_3D('',#17344,#13516,#13517);
#11506=AXIS2_PLACEMENT_3D('',#17346,#13519,#13520);
#11507=AXIS2_PLACEMENT_3D('',#17348,#13522,#13523);
#11508=AXIS2_PLACEMENT_3D('',#17352,#13526,#13527);
#11509=AXIS2_PLACEMENT_3D('',#17356,#13530,#13531);
#11510=AXIS2_PLACEMENT_3D('',#17362,#13535,#13536);
#11511=AXIS2_PLACEMENT_3D('',#17366,#13539,#13540);
#11512=AXIS2_PLACEMENT_3D('',#17368,#13542,#13543);
#11513=AXIS2_PLACEMENT_3D('',#17372,#13546,#13547);
#11514=AXIS2_PLACEMENT_3D('',#17378,#13551,#13552);
#11515=AXIS2_PLACEMENT_3D('',#17382,#13555,#13556);
#11516=AXIS2_PLACEMENT_3D('',#17386,#13559,#13560);
#11517=AXIS2_PLACEMENT_3D('',#17390,#13563,#13564);
#11518=AXIS2_PLACEMENT_3D('',#17392,#13566,#13567);
#11519=AXIS2_PLACEMENT_3D('',#17394,#13569,#13570);
#11520=AXIS2_PLACEMENT_3D('',#17396,#13572,#13573);
#11521=AXIS2_PLACEMENT_3D('',#17398,#13575,#13576);
#11522=AXIS2_PLACEMENT_3D('',#17399,#13577,#13578);
#11523=AXIS2_PLACEMENT_3D('',#17400,#13579,#13580);
#11524=AXIS2_PLACEMENT_3D('',#17401,#13581,#13582);
#11525=AXIS2_PLACEMENT_3D('',#17402,#13583,#13584);
#11526=AXIS2_PLACEMENT_3D('',#17403,#13585,#13586);
#11527=AXIS2_PLACEMENT_3D('',#17404,#13587,#13588);
#11528=AXIS2_PLACEMENT_3D('',#17405,#13589,#13590);
#11529=AXIS2_PLACEMENT_3D('',#17406,#13591,#13592);
#11530=AXIS2_PLACEMENT_3D('',#17407,#13593,#13594);
#11531=AXIS2_PLACEMENT_3D('',#17408,#13595,#13596);
#11532=AXIS2_PLACEMENT_3D('',#17409,#13597,#13598);
#11533=AXIS2_PLACEMENT_3D('',#17410,#13599,#13600);
#11534=AXIS2_PLACEMENT_3D('',#17411,#13601,#13602);
#11535=AXIS2_PLACEMENT_3D('',#17412,#13603,#13604);
#11536=AXIS2_PLACEMENT_3D('',#17413,#13605,#13606);
#11537=AXIS2_PLACEMENT_3D('',#17414,#13607,#13608);
#11538=AXIS2_PLACEMENT_3D('',#17415,#13609,#13610);
#11539=AXIS2_PLACEMENT_3D('',#17416,#13611,#13612);
#11540=AXIS2_PLACEMENT_3D('',#17417,#13613,#13614);
#11541=AXIS2_PLACEMENT_3D('',#17418,#13615,#13616);
#11542=AXIS2_PLACEMENT_3D('',#17419,#13617,#13618);
#11543=AXIS2_PLACEMENT_3D('',#17420,#13619,#13620);
#11544=AXIS2_PLACEMENT_3D('',#17421,#13621,#13622);
#11545=AXIS2_PLACEMENT_3D('',#17422,#13623,#13624);
#11546=AXIS2_PLACEMENT_3D('',#17423,#13625,#13626);
#11547=AXIS2_PLACEMENT_3D('',#17424,#13627,#13628);
#11548=AXIS2_PLACEMENT_3D('',#17425,#13629,#13630);
#11549=AXIS2_PLACEMENT_3D('',#17426,#13631,#13632);
#11550=AXIS2_PLACEMENT_3D('',#17427,#13633,#13634);
#11551=AXIS2_PLACEMENT_3D('',#17428,#13635,#13636);
#11552=AXIS2_PLACEMENT_3D('',#17429,#13637,#13638);
#11553=AXIS2_PLACEMENT_3D('',#17430,#13639,#13640);
#11554=AXIS2_PLACEMENT_3D('',#17431,#13641,#13642);
#11555=AXIS2_PLACEMENT_3D('',#17432,#13643,#13644);
#11556=AXIS2_PLACEMENT_3D('',#17433,#13645,#13646);
#11557=AXIS2_PLACEMENT_3D('',#17435,#13648,#13649);
#11558=AXIS2_PLACEMENT_3D('',#17439,#13652,#13653);
#11559=AXIS2_PLACEMENT_3D('',#17441,#13655,#13656);
#11560=AXIS2_PLACEMENT_3D('',#17443,#13658,#13659);
#11561=AXIS2_PLACEMENT_3D('',#17445,#13661,#13662);
#11562=AXIS2_PLACEMENT_3D('',#17447,#13664,#13665);
#11563=AXIS2_PLACEMENT_3D('',#17451,#13668,#13669);
#11564=AXIS2_PLACEMENT_3D('',#17455,#13672,#13673);
#11565=AXIS2_PLACEMENT_3D('',#17460,#13677,#13678);
#11566=AXIS2_PLACEMENT_3D('',#17462,#13680,#13681);
#11567=AXIS2_PLACEMENT_3D('',#17464,#13683,#13684);
#11568=AXIS2_PLACEMENT_3D('',#17466,#13686,#13687);
#11569=AXIS2_PLACEMENT_3D('',#17470,#13690,#13691);
#11570=AXIS2_PLACEMENT_3D('',#17474,#13694,#13695);
#11571=AXIS2_PLACEMENT_3D('',#17478,#13698,#13699);
#11572=AXIS2_PLACEMENT_3D('',#17482,#13702,#13703);
#11573=AXIS2_PLACEMENT_3D('',#17484,#13705,#13706);
#11574=AXIS2_PLACEMENT_3D('',#17486,#13708,#13709);
#11575=AXIS2_PLACEMENT_3D('',#17490,#13712,#13713);
#11576=AXIS2_PLACEMENT_3D('',#17495,#13717,#13718);
#11577=AXIS2_PLACEMENT_3D('',#17499,#13721,#13722);
#11578=AXIS2_PLACEMENT_3D('',#17505,#13726,#13727);
#11579=AXIS2_PLACEMENT_3D('',#17509,#13730,#13731);
#11580=AXIS2_PLACEMENT_3D('',#17513,#13734,#13735);
#11581=AXIS2_PLACEMENT_3D('',#17517,#13738,#13739);
#11582=AXIS2_PLACEMENT_3D('',#17521,#13742,#13743);
#11583=AXIS2_PLACEMENT_3D('',#17523,#13744,#13745);
#11584=AXIS2_PLACEMENT_3D('',#17529,#13749,#13750);
#11585=AXIS2_PLACEMENT_3D('',#17531,#13751,#13752);
#11586=AXIS2_PLACEMENT_3D('',#17533,#13754,#13755);
#11587=AXIS2_PLACEMENT_3D('',#17541,#13760,#13761);
#11588=AXIS2_PLACEMENT_3D('',#17544,#13764,#13765);
#11589=AXIS2_PLACEMENT_3D('',#17545,#13766,#13767);
#11590=AXIS2_PLACEMENT_3D('',#17549,#13770,#13771);
#11591=AXIS2_PLACEMENT_3D('',#17557,#13776,#13777);
#11592=AXIS2_PLACEMENT_3D('',#17565,#13782,#13783);
#11593=AXIS2_PLACEMENT_3D('',#17571,#13787,#13788);
#11594=AXIS2_PLACEMENT_3D('',#17579,#13793,#13794);
#11595=AXIS2_PLACEMENT_3D('',#17587,#13799,#13800);
#11596=AXIS2_PLACEMENT_3D('',#17593,#13804,#13805);
#11597=AXIS2_PLACEMENT_3D('',#17595,#13807,#13808);
#11598=AXIS2_PLACEMENT_3D('',#17597,#13810,#13811);
#11599=AXIS2_PLACEMENT_3D('',#17599,#13813,#13814);
#11600=AXIS2_PLACEMENT_3D('',#17603,#13817,#13818);
#11601=AXIS2_PLACEMENT_3D('',#17609,#13822,#13823);
#11602=AXIS2_PLACEMENT_3D('',#17613,#13826,#13827);
#11603=AXIS2_PLACEMENT_3D('',#17617,#13830,#13831);
#11604=AXIS2_PLACEMENT_3D('',#17621,#13834,#13835);
#11605=AXIS2_PLACEMENT_3D('',#17623,#13837,#13838);
#11606=AXIS2_PLACEMENT_3D('',#17625,#13840,#13841);
#11607=AXIS2_PLACEMENT_3D('',#17627,#13843,#13844);
#11608=AXIS2_PLACEMENT_3D('',#17628,#13845,#13846);
#11609=AXIS2_PLACEMENT_3D('',#17630,#13848,#13849);
#11610=AXIS2_PLACEMENT_3D('',#17632,#13851,#13852);
#11611=AXIS2_PLACEMENT_3D('',#17636,#13855,#13856);
#11612=AXIS2_PLACEMENT_3D('',#17649,#13865,#13866);
#11613=AXIS2_PLACEMENT_3D('',#17654,#13870,#13871);
#11614=AXIS2_PLACEMENT_3D('',#17655,#13872,#13873);
#11615=AXIS2_PLACEMENT_3D('',#17657,#13875,#13876);
#11616=AXIS2_PLACEMENT_3D('',#17667,#13882,#13883);
#11617=AXIS2_PLACEMENT_3D('',#17668,#13884,#13885);
#11618=AXIS2_PLACEMENT_3D('',#17670,#13887,#13888);
#11619=AXIS2_PLACEMENT_3D('',#17671,#13889,#13890);
#11620=AXIS2_PLACEMENT_3D('',#17673,#13892,#13893);
#11621=AXIS2_PLACEMENT_3D('',#17674,#13894,#13895);
#11622=AXIS2_PLACEMENT_3D('',#17675,#13896,#13897);
#11623=AXIS2_PLACEMENT_3D('',#17677,#13899,#13900);
#11624=AXIS2_PLACEMENT_3D('',#17678,#13901,#13902);
#11625=AXIS2_PLACEMENT_3D('',#17680,#13904,#13905);
#11626=AXIS2_PLACEMENT_3D('',#17684,#13908,#13909);
#11627=AXIS2_PLACEMENT_3D('',#17687,#13912,#13913);
#11628=AXIS2_PLACEMENT_3D('',#17689,#13915,#13916);
#11629=AXIS2_PLACEMENT_3D('',#17690,#13917,#13918);
#11630=AXIS2_PLACEMENT_3D('',#17692,#13920,#13921);
#11631=AXIS2_PLACEMENT_3D('',#17693,#13922,#13923);
#11632=AXIS2_PLACEMENT_3D('',#17696,#13926,#13927);
#11633=AXIS2_PLACEMENT_3D('',#17698,#13929,#13930);
#11634=AXIS2_PLACEMENT_3D('',#17699,#13931,#13932);
#11635=AXIS2_PLACEMENT_3D('',#17700,#13933,#13934);
#11636=AXIS2_PLACEMENT_3D('',#17755,#13935,#13936);
#11637=AXIS2_PLACEMENT_3D('',#17937,#13937,#13938);
#11638=AXIS2_PLACEMENT_3D('',#18119,#13939,#13940);
#11639=AXIS2_PLACEMENT_3D('',#18174,#13941,#13942);
#11640=AXIS2_PLACEMENT_3D('',#18229,#13943,#13944);
#11641=AXIS2_PLACEMENT_3D('',#18411,#13945,#13946);
#11642=AXIS2_PLACEMENT_3D('',#18412,#13947,#13948);
#11643=AXIS2_PLACEMENT_3D('',#18414,#13950,#13951);
#11644=AXIS2_PLACEMENT_3D('',#18415,#13952,#13953);
#11645=AXIS2_PLACEMENT_3D('',#18417,#13955,#13956);
#11646=AXIS2_PLACEMENT_3D('',#18418,#13957,#13958);
#11647=AXIS2_PLACEMENT_3D('',#18428,#13964,#13965);
#11648=AXIS2_PLACEMENT_3D('',#18429,#13966,#13967);
#11649=AXIS2_PLACEMENT_3D('',#18431,#13969,#13970);
#11650=AXIS2_PLACEMENT_3D('',#18435,#13973,#13974);
#11651=AXIS2_PLACEMENT_3D('',#18438,#13977,#13978);
#11652=AXIS2_PLACEMENT_3D('',#18441,#13981,#13982);
#11653=AXIS2_PLACEMENT_3D('',#18442,#13983,#13984);
#11654=AXIS2_PLACEMENT_3D('',#18443,#13985,#13986);
#11655=AXIS2_PLACEMENT_3D('',#18444,#13987,#13988);
#11656=AXIS2_PLACEMENT_3D('',#18445,#13989,#13990);
#11657=AXIS2_PLACEMENT_3D('',#18446,#13991,#13992);
#11658=AXIS2_PLACEMENT_3D('',#18447,#13993,#13994);
#11659=AXIS2_PLACEMENT_3D('',#18453,#13998,#13999);
#11660=AXIS2_PLACEMENT_3D('',#18457,#14002,#14003);
#11661=AXIS2_PLACEMENT_3D('',#18461,#14006,#14007);
#11662=AXIS2_PLACEMENT_3D('',#18727,#14009,#14010);
#11663=AXIS2_PLACEMENT_3D('',#18733,#14014,#14015);
#11664=AXIS2_PLACEMENT_3D('',#18737,#14018,#14019);
#11665=AXIS2_PLACEMENT_3D('',#18741,#14022,#14023);
#11666=AXIS2_PLACEMENT_3D('',#18743,#14025,#14026);
#11667=AXIS2_PLACEMENT_3D('',#18744,#14027,#14028);
#11668=AXIS2_PLACEMENT_3D('',#18745,#14029,#14030);
#11669=AXIS2_PLACEMENT_3D('',#18746,#14031,#14032);
#11670=AXIS2_PLACEMENT_3D('',#18747,#14033,#14034);
#11671=AXIS2_PLACEMENT_3D('',#18748,#14035,#14036);
#11672=AXIS2_PLACEMENT_3D('',#18749,#14037,#14038);
#11673=AXIS2_PLACEMENT_3D('',#18750,#14039,#14040);
#12509=DIRECTION('axis',(0.,0.,1.));
#12510=DIRECTION('refdir',(1.,0.,0.));
#12511=DIRECTION('center_axis',(0.,0.,1.));
#12512=DIRECTION('ref_axis',(1.,0.,0.));
#12513=DIRECTION('center_axis',(0.,0.,-1.));
#12514=DIRECTION('ref_axis',(1.,0.,0.));
#12515=DIRECTION('',(0.,0.,-1.));
#12516=DIRECTION('center_axis',(0.,0.,-1.));
#12517=DIRECTION('ref_axis',(1.,0.,0.));
#12518=DIRECTION('center_axis',(0.,0.,-1.));
#12519=DIRECTION('ref_axis',(-1.,0.,0.));
#12520=DIRECTION('center_axis',(0.,0.,1.));
#12521=DIRECTION('ref_axis',(-1.,0.,0.));
#12522=DIRECTION('',(0.,0.,1.));
#12523=DIRECTION('center_axis',(0.,0.,-1.));
#12524=DIRECTION('ref_axis',(-1.,0.,0.));
#12525=DIRECTION('center_axis',(0.,0.,-1.));
#12526=DIRECTION('ref_axis',(-1.,0.,0.));
#12527=DIRECTION('center_axis',(0.,0.,-1.));
#12528=DIRECTION('ref_axis',(-1.,0.,0.));
#12529=DIRECTION('',(0.,0.,-1.));
#12530=DIRECTION('center_axis',(0.,0.,-1.));
#12531=DIRECTION('ref_axis',(-1.,0.,0.));
#12532=DIRECTION('center_axis',(0.,0.,-1.));
#12533=DIRECTION('ref_axis',(-1.,0.,0.));
#12534=DIRECTION('center_axis',(0.,0.,-1.));
#12535=DIRECTION('ref_axis',(-1.,0.,0.));
#12536=DIRECTION('',(0.,0.,-1.));
#12537=DIRECTION('center_axis',(0.,0.,-1.));
#12538=DIRECTION('ref_axis',(-1.,0.,0.));
#12539=DIRECTION('center_axis',(0.,0.,-1.));
#12540=DIRECTION('ref_axis',(-1.,0.,0.));
#12541=DIRECTION('center_axis',(0.,0.,-1.));
#12542=DIRECTION('ref_axis',(-1.,0.,0.));
#12543=DIRECTION('',(0.,0.,-1.));
#12544=DIRECTION('center_axis',(0.,0.,-1.));
#12545=DIRECTION('ref_axis',(-1.,0.,0.));
#12546=DIRECTION('center_axis',(0.,0.,-1.));
#12547=DIRECTION('ref_axis',(-1.,0.,0.));
#12548=DIRECTION('center_axis',(0.,0.,-1.));
#12549=DIRECTION('ref_axis',(-1.,0.,0.));
#12550=DIRECTION('',(0.,0.,-1.));
#12551=DIRECTION('center_axis',(0.,0.,-1.));
#12552=DIRECTION('ref_axis',(-1.,0.,0.));
#12553=DIRECTION('center_axis',(0.,0.,-1.));
#12554=DIRECTION('ref_axis',(-1.,0.,0.));
#12555=DIRECTION('center_axis',(0.,0.,-1.));
#12556=DIRECTION('ref_axis',(-1.,0.,0.));
#12557=DIRECTION('',(0.,0.,-1.));
#12558=DIRECTION('center_axis',(0.,0.,-1.));
#12559=DIRECTION('ref_axis',(-1.,0.,0.));
#12560=DIRECTION('center_axis',(0.,0.,-1.));
#12561=DIRECTION('ref_axis',(-1.,0.,0.));
#12562=DIRECTION('center_axis',(0.,0.,-1.));
#12563=DIRECTION('ref_axis',(-1.,0.,0.));
#12564=DIRECTION('',(0.,0.,-1.));
#12565=DIRECTION('center_axis',(0.,0.,-1.));
#12566=DIRECTION('ref_axis',(-1.,0.,0.));
#12567=DIRECTION('center_axis',(0.,0.,-1.));
#12568=DIRECTION('ref_axis',(-1.,0.,0.));
#12569=DIRECTION('center_axis',(0.,0.,-1.));
#12570=DIRECTION('ref_axis',(-1.,0.,0.));
#12571=DIRECTION('',(0.,0.,-1.));
#12572=DIRECTION('center_axis',(0.,0.,1.));
#12573=DIRECTION('ref_axis',(-1.,0.,0.));
#12574=DIRECTION('center_axis',(0.,0.,-1.));
#12575=DIRECTION('ref_axis',(-1.,0.,0.));
#12576=DIRECTION('center_axis',(0.,0.,-1.));
#12577=DIRECTION('ref_axis',(-1.,0.,0.));
#12578=DIRECTION('',(0.,0.,-1.));
#12579=DIRECTION('center_axis',(0.,0.,1.));
#12580=DIRECTION('ref_axis',(-1.,0.,0.));
#12581=DIRECTION('center_axis',(0.,0.,-1.));
#12582=DIRECTION('ref_axis',(-1.,0.,0.));
#12583=DIRECTION('center_axis',(0.,0.,-1.));
#12584=DIRECTION('ref_axis',(-1.,0.,0.));
#12585=DIRECTION('',(0.,0.,-1.));
#12586=DIRECTION('center_axis',(0.,0.,1.));
#12587=DIRECTION('ref_axis',(-1.,0.,0.));
#12588=DIRECTION('center_axis',(0.,0.,-1.));
#12589=DIRECTION('ref_axis',(-1.,0.,0.));
#12590=DIRECTION('center_axis',(0.,0.,-1.));
#12591=DIRECTION('ref_axis',(-1.,0.,0.));
#12592=DIRECTION('',(0.,0.,-1.));
#12593=DIRECTION('center_axis',(0.,0.,1.));
#12594=DIRECTION('ref_axis',(-1.,0.,0.));
#12595=DIRECTION('center_axis',(0.,0.,-1.));
#12596=DIRECTION('ref_axis',(-1.,0.,0.));
#12597=DIRECTION('center_axis',(0.,0.,-1.));
#12598=DIRECTION('ref_axis',(-1.,0.,0.));
#12599=DIRECTION('',(0.,0.,-1.));
#12600=DIRECTION('center_axis',(0.,0.,1.));
#12601=DIRECTION('ref_axis',(-1.,0.,0.));
#12602=DIRECTION('center_axis',(0.,0.,-1.));
#12603=DIRECTION('ref_axis',(-1.,0.,0.));
#12604=DIRECTION('center_axis',(0.,0.,-1.));
#12605=DIRECTION('ref_axis',(-1.,0.,0.));
#12606=DIRECTION('',(0.,0.,-1.));
#12607=DIRECTION('center_axis',(0.,0.,1.));
#12608=DIRECTION('ref_axis',(-1.,0.,0.));
#12609=DIRECTION('center_axis',(0.,0.,-1.));
#12610=DIRECTION('ref_axis',(-1.,0.,0.));
#12611=DIRECTION('center_axis',(0.,0.,1.));
#12612=DIRECTION('ref_axis',(-1.,0.,0.));
#12613=DIRECTION('',(0.,0.,1.));
#12614=DIRECTION('center_axis',(0.,0.,-1.));
#12615=DIRECTION('ref_axis',(-1.,0.,0.));
#12616=DIRECTION('center_axis',(0.,0.,1.));
#12617=DIRECTION('ref_axis',(1.,0.,0.));
#12618=DIRECTION('center_axis',(0.,0.,-1.));
#12619=DIRECTION('ref_axis',(1.,0.,0.));
#12620=DIRECTION('',(0.,0.,1.));
#12621=DIRECTION('center_axis',(0.,0.,-1.));
#12622=DIRECTION('ref_axis',(1.,0.,0.));
#12623=DIRECTION('center_axis',(0.,0.,-1.));
#12624=DIRECTION('ref_axis',(-1.,0.,0.));
#12625=DIRECTION('center_axis',(0.,0.,1.));
#12626=DIRECTION('ref_axis',(-1.,0.,0.));
#12627=DIRECTION('',(0.,0.,1.));
#12628=DIRECTION('center_axis',(0.,0.,-1.));
#12629=DIRECTION('ref_axis',(-1.,0.,0.));
#12630=DIRECTION('center_axis',(0.,0.,1.));
#12631=DIRECTION('ref_axis',(1.,0.,0.));
#12632=DIRECTION('center_axis',(0.,0.,-1.));
#12633=DIRECTION('ref_axis',(1.,0.,0.));
#12634=DIRECTION('',(0.,0.,-1.));
#12635=DIRECTION('center_axis',(0.,0.,1.));
#12636=DIRECTION('ref_axis',(1.,0.,0.));
#12637=DIRECTION('center_axis',(0.,0.,-1.));
#12638=DIRECTION('ref_axis',(-1.,0.,0.));
#12639=DIRECTION('center_axis',(0.,0.,1.));
#12640=DIRECTION('ref_axis',(-1.,0.,0.));
#12641=DIRECTION('',(0.,0.,1.));
#12642=DIRECTION('center_axis',(0.,0.,-1.));
#12643=DIRECTION('ref_axis',(-1.,0.,0.));
#12644=DIRECTION('center_axis',(0.,0.,-1.));
#12645=DIRECTION('ref_axis',(-1.,0.,0.));
#12646=DIRECTION('center_axis',(0.,0.,1.));
#12647=DIRECTION('ref_axis',(-1.,0.,0.));
#12648=DIRECTION('',(0.,0.,1.));
#12649=DIRECTION('center_axis',(0.,0.,-1.));
#12650=DIRECTION('ref_axis',(-1.,0.,0.));
#12651=DIRECTION('center_axis',(0.,0.,-1.));
#12652=DIRECTION('ref_axis',(-1.,0.,0.));
#12653=DIRECTION('center_axis',(0.,0.,1.));
#12654=DIRECTION('ref_axis',(-1.,0.,0.));
#12655=DIRECTION('',(0.,0.,1.));
#12656=DIRECTION('center_axis',(0.,0.,1.));
#12657=DIRECTION('ref_axis',(-1.,0.,0.));
#12658=DIRECTION('center_axis',(0.,0.,-1.));
#12659=DIRECTION('ref_axis',(-1.,0.,0.));
#12660=DIRECTION('center_axis',(0.,0.,1.));
#12661=DIRECTION('ref_axis',(-1.,0.,0.));
#12662=DIRECTION('',(0.,0.,1.));
#12663=DIRECTION('center_axis',(0.,0.,1.));
#12664=DIRECTION('ref_axis',(-1.,0.,0.));
#12665=DIRECTION('center_axis',(0.,0.,1.));
#12666=DIRECTION('ref_axis',(1.,0.,0.));
#12667=DIRECTION('',(0.,1.,0.));
#12668=DIRECTION('',(-1.,0.,0.));
#12669=DIRECTION('',(0.,-1.,0.));
#12670=DIRECTION('',(1.,0.,0.));
#12671=DIRECTION('center_axis',(-1.,0.,0.));
#12672=DIRECTION('ref_axis',(0.,0.,1.));
#12673=DIRECTION('center_axis',(-1.,0.,0.));
#12674=DIRECTION('ref_axis',(0.,0.,1.));
#12675=DIRECTION('',(-1.,0.,0.));
#12676=DIRECTION('center_axis',(1.,0.,0.));
#12677=DIRECTION('ref_axis',(0.,2.04046848861772E-11,1.));
#12678=DIRECTION('center_axis',(0.,1.,0.));
#12679=DIRECTION('ref_axis',(0.,0.,1.));
#12680=DIRECTION('',(0.,1.,0.));
#12681=DIRECTION('center_axis',(0.,-1.,0.));
#12682=DIRECTION('ref_axis',(-1.10629098474627E-11,0.,1.));
#12683=DIRECTION('center_axis',(0.,1.,0.));
#12684=DIRECTION('ref_axis',(0.,0.,1.));
#12685=DIRECTION('center_axis',(1.,0.,0.));
#12686=DIRECTION('ref_axis',(0.,0.,-1.));
#12687=DIRECTION('',(1.,0.,0.));
#12688=DIRECTION('center_axis',(-1.,0.,0.));
#12689=DIRECTION('ref_axis',(0.,0.,-1.));
#12690=DIRECTION('center_axis',(1.,0.,0.));
#12691=DIRECTION('ref_axis',(0.,0.,-1.));
#12692=DIRECTION('center_axis',(0.,-1.,0.));
#12693=DIRECTION('ref_axis',(0.,0.,-1.));
#12694=DIRECTION('center_axis',(0.,-1.,0.));
#12695=DIRECTION('ref_axis',(0.,0.,-1.));
#12696=DIRECTION('',(0.,-1.,0.));
#12697=DIRECTION('center_axis',(0.,1.,0.));
#12698=DIRECTION('ref_axis',(-1.15648231731787E-15,0.,-1.));
#12699=DIRECTION('center_axis',(0.,0.,1.));
#12700=DIRECTION('ref_axis',(1.,0.,0.));
#12701=DIRECTION('center_axis',(0.,1.,0.));
#12702=DIRECTION('ref_axis',(0.,0.,1.));
#12703=DIRECTION('',(0.,0.,1.));
#12704=DIRECTION('',(-1.,0.,0.));
#12705=DIRECTION('',(0.,0.,-1.));
#12706=DIRECTION('',(-1.,0.,0.));
#12707=DIRECTION('',(0.,0.,-1.));
#12708=DIRECTION('',(-1.,0.,0.));
#12709=DIRECTION('',(0.,0.,-1.));
#12710=DIRECTION('',(-1.,0.,0.));
#12711=DIRECTION('',(-1.,0.,0.));
#12712=DIRECTION('',(-1.,0.,0.));
#12713=DIRECTION('',(0.,0.,1.));
#12714=DIRECTION('',(-1.,0.,0.));
#12715=DIRECTION('',(0.,0.,1.));
#12716=DIRECTION('',(-1.,0.,0.));
#12717=DIRECTION('',(0.,0.,1.));
#12718=DIRECTION('',(-1.,0.,0.));
#12719=DIRECTION('',(0.,0.,-1.));
#12720=DIRECTION('center_axis',(-1.,7.30644979272993E-12,1.28397990694513E-11));
#12721=DIRECTION('ref_axis',(1.28397990694513E-11,4.61084724568329E-27,
1.));
#12722=DIRECTION('center_axis',(1.28419072818016E-11,-4.85794204139804E-12,
1.));
#12723=DIRECTION('ref_axis',(1.,1.59160909755483E-27,-1.28419072818016E-11));
#12724=DIRECTION('center_axis',(1.,-6.33047047191158E-12,6.77618385437683E-12));
#12725=DIRECTION('ref_axis',(-6.77618385426471E-12,1.77115266899322E-11,
1.));
#12726=DIRECTION('center_axis',(-6.77562190498519E-12,5.3501387359779E-10,
1.));
#12727=DIRECTION('ref_axis',(1.95819442432296E-27,-1.,5.3501387359779E-10));
#12728=DIRECTION('center_axis',(1.,0.,0.));
#12729=DIRECTION('ref_axis',(0.,0.,-1.));
#12730=DIRECTION('',(0.,0.,-1.));
#12731=DIRECTION('',(0.,1.,0.));
#12732=DIRECTION('',(0.,0.,1.));
#12733=DIRECTION('center_axis',(0.,0.,1.));
#12734=DIRECTION('ref_axis',(1.,0.,0.));
#12735=DIRECTION('center_axis',(0.,-1.,0.));
#12736=DIRECTION('ref_axis',(0.,0.,-1.));
#12737=DIRECTION('',(0.,0.,1.));
#12738=DIRECTION('',(0.,0.,-1.));
#12739=DIRECTION('',(1.,0.,0.));
#12740=DIRECTION('center_axis',(0.,0.,1.));
#12741=DIRECTION('ref_axis',(1.,0.,0.));
#12742=DIRECTION('center_axis',(-1.,0.,0.));
#12743=DIRECTION('ref_axis',(0.,0.,1.));
#12744=DIRECTION('',(0.,0.,-1.));
#12745=DIRECTION('',(0.,-1.,0.));
#12746=DIRECTION('',(0.,0.,1.));
#12747=DIRECTION('center_axis',(0.,0.,-1.));
#12748=DIRECTION('ref_axis',(-1.,0.,0.));
#12749=DIRECTION('',(0.,0.,1.));
#12750=DIRECTION('center_axis',(0.,0.,-1.));
#12751=DIRECTION('ref_axis',(-1.,0.,0.));
#12752=DIRECTION('center_axis',(0.,0.,1.));
#12753=DIRECTION('ref_axis',(-1.,-1.73472347597681E-15,0.));
#12754=DIRECTION('center_axis',(0.,0.,-1.));
#12755=DIRECTION('ref_axis',(-1.,0.,0.));
#12756=DIRECTION('',(0.,0.,1.));
#12757=DIRECTION('center_axis',(0.,0.,-1.));
#12758=DIRECTION('ref_axis',(-1.,0.,0.));
#12759=DIRECTION('center_axis',(0.,0.,1.));
#12760=DIRECTION('ref_axis',(-1.,0.,0.));
#12761=DIRECTION('center_axis',(0.,0.,-1.));
#12762=DIRECTION('ref_axis',(-1.,0.,0.));
#12763=DIRECTION('',(0.,0.,1.));
#12764=DIRECTION('center_axis',(0.,0.,-1.));
#12765=DIRECTION('ref_axis',(-1.,0.,0.));
#12766=DIRECTION('center_axis',(0.,0.,1.));
#12767=DIRECTION('ref_axis',(-1.,-5.20417042793042E-15,0.));
#12768=DIRECTION('center_axis',(0.,0.,1.));
#12769=DIRECTION('ref_axis',(1.,0.,0.));
#12770=DIRECTION('',(0.,1.,0.));
#12771=DIRECTION('center_axis',(0.,0.,1.));
#12772=DIRECTION('ref_axis',(-1.,0.,0.));
#12773=DIRECTION('',(0.562310021407237,0.826926502069557,0.));
#12774=DIRECTION('center_axis',(0.,0.,1.));
#12775=DIRECTION('ref_axis',(-1.,-2.31296463463574E-15,0.));
#12776=DIRECTION('',(1.,0.,0.));
#12777=DIRECTION('center_axis',(0.,0.,1.));
#12778=DIRECTION('ref_axis',(-1.,2.31296463463574E-15,0.));
#12779=DIRECTION('',(0.562310021407237,-0.826926502069557,0.));
#12780=DIRECTION('center_axis',(0.,0.,1.));
#12781=DIRECTION('ref_axis',(-1.,0.,0.));
#12782=DIRECTION('',(0.,-1.,0.));
#12783=DIRECTION('center_axis',(0.,0.,1.));
#12784=DIRECTION('ref_axis',(-1.,-3.46944695195362E-15,0.));
#12785=DIRECTION('',(-0.562310021407322,-0.826926502069499,0.));
#12786=DIRECTION('center_axis',(6.0998774063795E-15,-4.61958004021261E-15,
-1.));
#12787=DIRECTION('ref_axis',(0.,1.,-4.44089209850062E-15));
#12788=DIRECTION('',(0.,1.,0.));
#12789=DIRECTION('center_axis',(0.,0.,1.));
#12790=DIRECTION('ref_axis',(-1.,0.,0.));
#12791=DIRECTION('',(1.,0.,0.));
#12792=DIRECTION('center_axis',(0.,0.,-1.));
#12793=DIRECTION('ref_axis',(-1.,0.,0.));
#12794=DIRECTION('',(0.,1.,0.));
#12795=DIRECTION('center_axis',(0.,0.,-1.));
#12796=DIRECTION('ref_axis',(1.,0.,0.));
#12797=DIRECTION('',(-1.,0.,0.));
#12798=DIRECTION('center_axis',(0.,0.,1.));
#12799=DIRECTION('ref_axis',(-1.,0.,0.));
#12800=DIRECTION('',(0.,1.,0.));
#12801=DIRECTION('center_axis',(0.,0.,-1.));
#12802=DIRECTION('ref_axis',(-1.,0.,0.));
#12803=DIRECTION('',(-1.,0.,0.));
#12804=DIRECTION('center_axis',(0.,0.,-1.));
#12805=DIRECTION('ref_axis',(1.,0.,0.));
#12806=DIRECTION('',(0.,-1.,0.));
#12807=DIRECTION('center_axis',(0.,0.,1.));
#12808=DIRECTION('ref_axis',(-1.,0.,0.));
#12809=DIRECTION('',(-1.,0.,0.));
#12810=DIRECTION('center_axis',(0.,0.,-1.));
#12811=DIRECTION('ref_axis',(-1.,0.,0.));
#12812=DIRECTION('',(0.,-1.,0.));
#12813=DIRECTION('center_axis',(0.,0.,-1.));
#12814=DIRECTION('ref_axis',(1.,-2.60208521396521E-15,0.));
#12815=DIRECTION('',(1.,0.,0.));
#12816=DIRECTION('center_axis',(0.,0.,1.));
#12817=DIRECTION('ref_axis',(-1.,0.,0.));
#12818=DIRECTION('',(0.,-1.,0.));
#12819=DIRECTION('center_axis',(0.,0.,-1.));
#12820=DIRECTION('ref_axis',(1.,4.4408920985006E-15,0.));
#12821=DIRECTION('center_axis',(0.,0.,1.));
#12822=DIRECTION('ref_axis',(-1.,-4.33680868994202E-15,0.));
#12823=DIRECTION('',(-0.562310021407322,0.826926502069499,0.));
#12824=DIRECTION('center_axis',(0.,0.,1.));
#12825=DIRECTION('ref_axis',(-1.,0.,0.));
#12826=DIRECTION('center_axis',(1.,0.,0.));
#12827=DIRECTION('ref_axis',(0.,0.,-1.));
#12828=DIRECTION('center_axis',(1.,0.,0.));
#12829=DIRECTION('ref_axis',(0.,0.,-1.));
#12830=DIRECTION('center_axis',(-1.,0.,0.));
#12831=DIRECTION('ref_axis',(0.,0.,-1.));
#12832=DIRECTION('',(-1.,0.,0.));
#12833=DIRECTION('center_axis',(0.,0.,-1.));
#12834=DIRECTION('ref_axis',(-1.,0.,0.));
#12835=DIRECTION('center_axis',(0.,0.,-1.));
#12836=DIRECTION('ref_axis',(-1.,0.,0.));
#12837=DIRECTION('',(0.,0.,-1.));
#12838=DIRECTION('center_axis',(0.,0.,-1.));
#12839=DIRECTION('ref_axis',(-1.,0.,0.));
#12840=DIRECTION('center_axis',(0.,0.,-1.));
#12841=DIRECTION('ref_axis',(-1.,0.,0.));
#12842=DIRECTION('',(0.,0.,-1.));
#12843=DIRECTION('center_axis',(0.,0.,1.));
#12844=DIRECTION('ref_axis',(-1.,0.,0.));
#12845=DIRECTION('center_axis',(0.,0.,-1.));
#12846=DIRECTION('ref_axis',(-1.,0.,0.));
#12847=DIRECTION('center_axis',(0.,0.,-1.));
#12848=DIRECTION('ref_axis',(-1.,0.,0.));
#12849=DIRECTION('',(0.,0.,-1.));
#12850=DIRECTION('center_axis',(0.,0.,1.));
#12851=DIRECTION('ref_axis',(-1.,0.,0.));
#12852=DIRECTION('center_axis',(0.,0.,-1.));
#12853=DIRECTION('ref_axis',(0.707106813086204,0.70710674928689,0.));
#12854=DIRECTION('center_axis',(0.,0.,1.));
#12855=DIRECTION('ref_axis',(-1.,0.,0.));
#12856=DIRECTION('center_axis',(0.,0.,1.));
#12857=DIRECTION('ref_axis',(1.,0.,0.));
#12858=DIRECTION('center_axis',(0.,0.,1.));
#12859=DIRECTION('ref_axis',(1.,0.,0.));
#12860=DIRECTION('center_axis',(0.,0.,1.));
#12861=DIRECTION('ref_axis',(1.,0.,0.));
#12862=DIRECTION('center_axis',(0.,0.,1.));
#12863=DIRECTION('ref_axis',(-1.,2.31296463463574E-15,0.));
#12864=DIRECTION('',(0.,1.,0.));
#12865=DIRECTION('center_axis',(0.,0.,1.));
#12866=DIRECTION('ref_axis',(-1.,0.,0.));
#12867=DIRECTION('',(-0.562310021407322,0.826926502069499,0.));
#12868=DIRECTION('center_axis',(0.,0.,-1.));
#12869=DIRECTION('ref_axis',(-1.,0.,0.));
#12870=DIRECTION('center_axis',(0.,0.,-1.));
#12871=DIRECTION('ref_axis',(-1.,0.,0.));
#12872=DIRECTION('',(-0.562310021407322,-0.826926502069499,0.));
#12873=DIRECTION('center_axis',(0.,0.,1.));
#12874=DIRECTION('ref_axis',(-1.,-3.46944695195362E-15,0.));
#12875=DIRECTION('',(0.,-1.,0.));
#12876=DIRECTION('center_axis',(0.,0.,1.));
#12877=DIRECTION('ref_axis',(-1.,0.,0.));
#12878=DIRECTION('',(0.562310021407237,-0.826926502069557,0.));
#12879=DIRECTION('center_axis',(0.,0.,1.));
#12880=DIRECTION('ref_axis',(-1.,2.31296463463574E-15,0.));
#12881=DIRECTION('',(1.,0.,0.));
#12882=DIRECTION('center_axis',(0.,0.,1.));
#12883=DIRECTION('ref_axis',(-1.,-2.31296463463574E-15,0.));
#12884=DIRECTION('',(0.562310021407237,0.826926502069557,0.));
#12885=DIRECTION('center_axis',(0.,0.,-1.));
#12886=DIRECTION('ref_axis',(-1.,0.,0.));
#12887=DIRECTION('center_axis',(3.41948691584553E-13,3.41948691584525E-13,
-1.));
#12888=DIRECTION('ref_axis',(-6.88338275267599E-14,-1.,-3.41948691584549E-13));
#12889=DIRECTION('center_axis',(0.,0.,-1.));
#12890=DIRECTION('ref_axis',(-1.,0.,0.));
#12891=DIRECTION('center_axis',(3.55271367880032E-13,-3.55271367880047E-13,
-1.));
#12892=DIRECTION('ref_axis',(-1.,7.10542735760108E-14,-3.55271367880054E-13));
#12893=DIRECTION('center_axis',(0.,0.,-1.));
#12894=DIRECTION('ref_axis',(-1.,0.,0.));
#12895=DIRECTION('center_axis',(-0.826926502069509,0.562310021407307,0.));
#12896=DIRECTION('ref_axis',(-0.562310021407307,-0.826926502069509,0.));
#12897=DIRECTION('',(0.,0.,1.));
#12898=DIRECTION('',(0.562310021410592,0.826926502067275,0.));
#12899=DIRECTION('',(0.,0.,1.));
#12900=DIRECTION('',(-0.562310021407307,-0.826926502069509,0.));
#12901=DIRECTION('',(0.,0.,-1.));
#12902=DIRECTION('',(-0.562310021407307,-0.826926502069509,0.));
#12903=DIRECTION('center_axis',(0.,0.,1.));
#12904=DIRECTION('ref_axis',(1.,0.,0.));
#12905=DIRECTION('',(0.,1.,0.));
#12906=DIRECTION('',(1.,0.,0.));
#12907=DIRECTION('center_axis',(-1.,0.,0.));
#12908=DIRECTION('ref_axis',(0.,0.,1.));
#12909=DIRECTION('',(0.,-1.,0.));
#12910=DIRECTION('',(0.,0.,1.));
#12911=DIRECTION('',(0.,1.,0.));
#12912=DIRECTION('',(0.,1.,0.));
#12913=DIRECTION('',(0.,0.,-1.));
#12914=DIRECTION('',(0.,1.,0.));
#12915=DIRECTION('',(0.,1.,0.));
#12916=DIRECTION('',(0.,1.,0.));
#12917=DIRECTION('',(0.,0.,1.));
#12918=DIRECTION('',(0.,1.,0.));
#12919=DIRECTION('',(0.,0.,-1.));
#12920=DIRECTION('',(0.,1.,0.));
#12921=DIRECTION('',(0.,1.,0.));
#12922=DIRECTION('',(0.,1.,0.));
#12923=DIRECTION('',(0.,0.,1.));
#12924=DIRECTION('',(0.,-1.,0.));
#12925=DIRECTION('',(0.,0.,1.));
#12926=DIRECTION('',(0.,-1.,0.));
#12927=DIRECTION('',(0.,-1.,0.));
#12928=DIRECTION('',(0.,-1.,0.));
#12929=DIRECTION('',(0.,0.,-1.));
#12930=DIRECTION('',(0.,-1.,0.));
#12931=DIRECTION('',(0.,0.,1.));
#12932=DIRECTION('',(0.,-1.,0.));
#12933=DIRECTION('',(0.,-1.,0.));
#12934=DIRECTION('',(0.,-1.,0.));
#12935=DIRECTION('',(0.,0.,1.));
#12936=DIRECTION('',(0.,-1.,0.));
#12937=DIRECTION('',(0.,0.,1.));
#12938=DIRECTION('',(0.,-1.,0.));
#12939=DIRECTION('',(0.,0.,-1.));
#12940=DIRECTION('',(0.,-1.,0.));
#12941=DIRECTION('',(0.,0.,-1.));
#12942=DIRECTION('',(0.,-1.,0.));
#12943=DIRECTION('',(0.,-1.,0.));
#12944=DIRECTION('',(0.,0.,1.));
#12945=DIRECTION('',(0.,1.,0.));
#12946=DIRECTION('',(0.,0.,1.));
#12947=DIRECTION('center_axis',(0.,0.,1.));
#12948=DIRECTION('ref_axis',(1.,0.,0.));
#12949=DIRECTION('',(-0.562310021407171,-0.826926502069602,0.));
#12950=DIRECTION('',(1.,0.,0.));
#12951=DIRECTION('center_axis',(0.826926502069509,-0.562310021407307,0.));
#12952=DIRECTION('ref_axis',(0.562310021407307,0.826926502069509,0.));
#12953=DIRECTION('',(0.562310021410592,0.826926502067275,0.));
#12954=DIRECTION('',(0.,0.,-1.));
#12955=DIRECTION('',(-0.562310021407307,-0.826926502069509,0.));
#12956=DIRECTION('',(0.,0.,1.));
#12957=DIRECTION('',(0.,0.,-1.));
#12958=DIRECTION('center_axis',(0.,0.,-1.));
#12959=DIRECTION('ref_axis',(-1.,0.,0.));
#12960=DIRECTION('',(0.,0.,1.));
#12961=DIRECTION('center_axis',(0.,0.,-1.));
#12962=DIRECTION('ref_axis',(-1.,0.,0.));
#12963=DIRECTION('',(0.,0.,-1.));
#12964=DIRECTION('center_axis',(-1.,0.,0.));
#12965=DIRECTION('ref_axis',(0.,0.,1.));
#12966=DIRECTION('',(0.,1.,0.));
#12967=DIRECTION('',(0.,0.,-1.));
#12968=DIRECTION('',(0.,1.,0.));
#12969=DIRECTION('',(0.,0.,1.));
#12970=DIRECTION('',(0.,1.,0.));
#12971=DIRECTION('',(0.,0.,-1.));
#12972=DIRECTION('',(0.,1.,0.));
#12973=DIRECTION('',(0.,0.,1.));
#12974=DIRECTION('',(0.,1.,0.));
#12975=DIRECTION('',(0.,0.,-1.));
#12976=DIRECTION('',(0.,1.,0.));
#12977=DIRECTION('',(0.,0.,1.));
#12978=DIRECTION('',(0.,1.,0.));
#12979=DIRECTION('',(0.,0.,1.));
#12980=DIRECTION('center_axis',(0.,0.,-1.));
#12981=DIRECTION('ref_axis',(-1.,0.,0.));
#12982=DIRECTION('center_axis',(0.,0.,-1.));
#12983=DIRECTION('ref_axis',(-1.,0.,0.));
#12984=DIRECTION('',(0.,0.,-1.));
#12985=DIRECTION('center_axis',(-0.826926502069509,0.562310021407307,0.));
#12986=DIRECTION('ref_axis',(-0.562310021407307,-0.826926502069509,0.));
#12987=DIRECTION('',(0.562310021407307,0.826926502069509,0.));
#12988=DIRECTION('',(0.,0.,1.));
#12989=DIRECTION('center_axis',(0.,0.,-1.));
#12990=DIRECTION('ref_axis',(-1.,0.,0.));
#12991=DIRECTION('center_axis',(0.,0.,-1.));
#12992=DIRECTION('ref_axis',(-1.,0.,0.));
#12993=DIRECTION('center_axis',(0.,0.,-1.));
#12994=DIRECTION('ref_axis',(-1.,0.,0.));
#12995=DIRECTION('',(0.,0.,-1.));
#12996=DIRECTION('center_axis',(0.,0.,-1.));
#12997=DIRECTION('ref_axis',(-1.,0.,0.));
#12998=DIRECTION('center_axis',(0.,1.,0.));
#12999=DIRECTION('ref_axis',(0.,0.,1.));
#13000=DIRECTION('',(1.,0.,0.));
#13001=DIRECTION('',(0.,0.,-1.));
#13002=DIRECTION('',(1.,0.,0.));
#13003=DIRECTION('',(0.,0.,1.));
#13004=DIRECTION('',(1.,0.,0.));
#13005=DIRECTION('',(0.,0.,-1.));
#13006=DIRECTION('',(1.,0.,0.));
#13007=DIRECTION('',(0.,0.,1.));
#13008=DIRECTION('',(1.,0.,0.));
#13009=DIRECTION('',(0.,0.,1.));
#13010=DIRECTION('center_axis',(0.,0.,-1.));
#13011=DIRECTION('ref_axis',(-1.,0.,0.));
#13012=DIRECTION('center_axis',(0.,0.,-1.));
#13013=DIRECTION('ref_axis',(-1.,0.,0.));
#13014=DIRECTION('center_axis',(0.,0.,-1.));
#13015=DIRECTION('ref_axis',(-1.,0.,0.));
#13016=DIRECTION('',(0.,0.,-1.));
#13017=DIRECTION('center_axis',(0.,0.,-1.));
#13018=DIRECTION('ref_axis',(-1.,0.,0.));
#13019=DIRECTION('center_axis',(0.826926502069509,0.562310021407307,0.));
#13020=DIRECTION('ref_axis',(-0.562310021407307,0.826926502069509,0.));
#13021=DIRECTION('',(0.562310021407307,-0.826926502069509,0.));
#13022=DIRECTION('',(0.,0.,1.));
#13023=DIRECTION('center_axis',(0.,0.,-1.));
#13024=DIRECTION('ref_axis',(-1.,0.,0.));
#13025=DIRECTION('center_axis',(0.,0.,-1.));
#13026=DIRECTION('ref_axis',(-1.,0.,0.));
#13027=DIRECTION('',(0.,0.,-1.));
#13028=DIRECTION('center_axis',(1.,0.,0.));
#13029=DIRECTION('ref_axis',(0.,0.,-1.));
#13030=DIRECTION('',(0.,-1.,0.));
#13031=DIRECTION('',(0.,0.,-1.));
#13032=DIRECTION('',(0.,-1.,0.));
#13033=DIRECTION('',(0.,0.,1.));
#13034=DIRECTION('',(0.,-1.,0.));
#13035=DIRECTION('',(0.,0.,-1.));
#13036=DIRECTION('',(0.,-1.,0.));
#13037=DIRECTION('',(0.,0.,1.));
#13038=DIRECTION('',(0.,-1.,0.));
#13039=DIRECTION('',(0.,0.,-1.));
#13040=DIRECTION('',(0.,-1.,0.));
#13041=DIRECTION('',(0.,0.,1.));
#13042=DIRECTION('',(0.,-1.,0.));
#13043=DIRECTION('',(0.,0.,1.));
#13044=DIRECTION('center_axis',(0.,0.,-1.));
#13045=DIRECTION('ref_axis',(-1.,0.,0.));
#13046=DIRECTION('center_axis',(0.,0.,-1.));
#13047=DIRECTION('ref_axis',(-1.,0.,0.));
#13048=DIRECTION('center_axis',(1.,9.94839377593602E-15,-1.10487024155554E-14));
#13049=DIRECTION('ref_axis',(-1.11656715619443E-14,0.,-1.));
#13050=DIRECTION('center_axis',(0.,1.,0.));
#13051=DIRECTION('ref_axis',(0.,0.,-1.));
#13052=DIRECTION('center_axis',(1.,-7.850462293419E-16,1.89526925396706E-15));
#13053=DIRECTION('ref_axis',(5.55111512312575E-16,1.,-6.6613381477509E-15));
#13054=DIRECTION('center_axis',(1.,0.,0.));
#13055=DIRECTION('ref_axis',(0.,0.,-1.));
#13056=DIRECTION('',(0.,1.,0.));
#13057=DIRECTION('',(0.,0.,-1.));
#13058=DIRECTION('center_axis',(0.,0.,-1.));
#13059=DIRECTION('ref_axis',(0.707106781233148,-0.707106781139947,0.));
#13060=DIRECTION('',(0.,0.,-1.));
#13061=DIRECTION('center_axis',(0.,0.,1.));
#13062=DIRECTION('ref_axis',(-1.,0.,0.));
#13063=DIRECTION('center_axis',(0.,-1.,0.));
#13064=DIRECTION('ref_axis',(0.,0.,-1.));
#13065=DIRECTION('',(0.,0.,-1.));
#13066=DIRECTION('',(1.,0.,0.));
#13067=DIRECTION('center_axis',(0.,0.,-1.));
#13068=DIRECTION('ref_axis',(-1.,0.,0.));
#13069=DIRECTION('center_axis',(-6.35468797035731E-9,6.35397964806342E-9,
-1.));
#13070=DIRECTION('ref_axis',(3.84137166520666E-13,1.,6.3539795647276E-9));
#13071=DIRECTION('',(0.,0.,1.));
#13072=DIRECTION('center_axis',(-1.,0.,0.));
#13073=DIRECTION('ref_axis',(0.,0.,1.));
#13074=DIRECTION('',(0.,-1.,0.));
#13075=DIRECTION('',(0.,0.,1.));
#13076=DIRECTION('center_axis',(0.,0.,1.));
#13077=DIRECTION('ref_axis',(1.,0.,0.));
#13078=DIRECTION('center_axis',(-6.36151393603232E-9,-6.36219561297833E-9,
-1.));
#13079=DIRECTION('ref_axis',(-1.,-5.67546010185474E-12,6.36151353813414E-9));
#13080=DIRECTION('',(0.,0.,1.));
#13081=DIRECTION('center_axis',(0.,1.,0.));
#13082=DIRECTION('ref_axis',(0.,0.,1.));
#13083=DIRECTION('',(0.,0.,-1.));
#13084=DIRECTION('',(-1.,0.,0.));
#13085=DIRECTION('center_axis',(0.,0.,-1.));
#13086=DIRECTION('ref_axis',(0.707106781233548,0.707106781139547,0.));
#13087=DIRECTION('',(0.,0.,-1.));
#13088=DIRECTION('center_axis',(0.,0.,1.));
#13089=DIRECTION('ref_axis',(-1.,0.,0.));
#13090=DIRECTION('center_axis',(1.,0.,0.));
#13091=DIRECTION('ref_axis',(0.,0.,-1.));
#13092=DIRECTION('',(0.,0.,-1.));
#13093=DIRECTION('',(0.,1.,0.));
#13094=DIRECTION('center_axis',(0.,0.,-1.));
#13095=DIRECTION('ref_axis',(-1.,0.,0.));
#13096=DIRECTION('center_axis',(-6.36152086670943E-9,-6.36220476409676E-9,
-1.));
#13097=DIRECTION('ref_axis',(-1.,3.73034936274398E-13,6.36152019951075E-9));
#13098=DIRECTION('',(0.,0.,1.));
#13099=DIRECTION('center_axis',(0.,-1.,0.));
#13100=DIRECTION('ref_axis',(0.,0.,-1.));
#13101=DIRECTION('',(1.,0.,0.));
#13102=DIRECTION('',(0.,0.,1.));
#13103=DIRECTION('center_axis',(0.,0.,1.));
#13104=DIRECTION('ref_axis',(1.,0.,0.));
#13105=DIRECTION('center_axis',(6.35475386807431E-9,-6.35404776622543E-9,
-1.));
#13106=DIRECTION('ref_axis',(5.99964522503824E-12,-1.,6.3540483985109E-9));
#13107=DIRECTION('',(0.,0.,1.));
#13108=DIRECTION('center_axis',(-1.,0.,0.));
#13109=DIRECTION('ref_axis',(0.,0.,1.));
#13110=DIRECTION('',(0.,0.,-1.));
#13111=DIRECTION('',(0.,-1.,0.));
#13112=DIRECTION('center_axis',(0.,0.,-1.));
#13113=DIRECTION('ref_axis',(-1.,0.,0.));
#13114=DIRECTION('',(0.,0.,-1.));
#13115=DIRECTION('center_axis',(0.,0.,1.));
#13116=DIRECTION('ref_axis',(-1.,0.,0.));
#13117=DIRECTION('center_axis',(0.,1.,0.));
#13118=DIRECTION('ref_axis',(0.,0.,1.));
#13119=DIRECTION('',(0.,0.,-1.));
#13120=DIRECTION('',(-1.,0.,0.));
#13121=DIRECTION('center_axis',(0.,0.,-1.));
#13122=DIRECTION('ref_axis',(-1.,0.,0.));
#13123=DIRECTION('center_axis',(6.35468797040853E-9,-6.35397964810999E-9,
-1.));
#13124=DIRECTION('ref_axis',(5.68434188605167E-12,-1.,6.35397956468904E-9));
#13125=DIRECTION('',(0.,0.,1.));
#13126=DIRECTION('center_axis',(1.,0.,0.));
#13127=DIRECTION('ref_axis',(0.,0.,-1.));
#13128=DIRECTION('',(0.,1.,0.));
#13129=DIRECTION('',(0.,0.,1.));
#13130=DIRECTION('center_axis',(0.,0.,1.));
#13131=DIRECTION('ref_axis',(1.,0.,0.));
#13132=DIRECTION('center_axis',(6.36153916910018E-9,6.36221862559652E-9,
-1.));
#13133=DIRECTION('ref_axis',(1.,6.00075544806287E-12,6.36154018348104E-9));
#13134=DIRECTION('',(0.,0.,1.));
#13135=DIRECTION('center_axis',(0.,-1.,0.));
#13136=DIRECTION('ref_axis',(0.,0.,-1.));
#13137=DIRECTION('',(0.,0.,-1.));
#13138=DIRECTION('',(1.,0.,0.));
#13139=DIRECTION('center_axis',(0.,0.,-1.));
#13140=DIRECTION('ref_axis',(-1.,0.,0.));
#13141=DIRECTION('',(0.,0.,-1.));
#13142=DIRECTION('center_axis',(0.,0.,1.));
#13143=DIRECTION('ref_axis',(-1.,0.,0.));
#13144=DIRECTION('center_axis',(-1.,0.,0.));
#13145=DIRECTION('ref_axis',(0.,0.,1.));
#13146=DIRECTION('',(0.,-1.,0.));
#13147=DIRECTION('center_axis',(-1.,-7.85046229341902E-16,1.89526925396706E-15));
#13148=DIRECTION('ref_axis',(-1.66533453693772E-15,6.66133814775089E-15,
-1.));
#13149=DIRECTION('center_axis',(1.,0.,0.));
#13150=DIRECTION('ref_axis',(0.,0.,-1.));
#13151=DIRECTION('center_axis',(0.,1.,0.));
#13152=DIRECTION('ref_axis',(0.,0.,-1.));
#13153=DIRECTION('center_axis',(-0.826926502069509,-0.562310021407307,0.));
#13154=DIRECTION('ref_axis',(0.562310021407307,-0.826926502069509,0.));
#13155=DIRECTION('',(-0.562310021407307,0.826926502069509,0.));
#13156=DIRECTION('',(0.,0.,-1.));
#13157=DIRECTION('',(-0.562310021407307,0.826926502069509,0.));
#13158=DIRECTION('',(0.,0.,1.));
#13159=DIRECTION('',(-0.562310021407307,0.826926502069509,0.));
#13160=DIRECTION('center_axis',(0.,0.,1.));
#13161=DIRECTION('ref_axis',(1.,0.,0.));
#13162=DIRECTION('center_axis',(-4.37239035198399E-13,-3.70337308189936E-13,
-1.));
#13163=DIRECTION('ref_axis',(-0.999999999999855,-5.39048211617437E-7,4.37168237134799E-13));
#13164=DIRECTION('',(-1.,0.,0.));
#13165=DIRECTION('',(0.,1.,0.));
#13166=DIRECTION('',(1.,0.,0.));
#13167=DIRECTION('center_axis',(-3.24372003830014E-13,4.24724639577507E-13,
-1.));
#13168=DIRECTION('ref_axis',(-4.6464532774625E-7,0.999999999999892,4.24480008512514E-13));
#13169=DIRECTION('',(0.,1.,0.));
#13170=DIRECTION('',(1.,0.,0.));
#13171=DIRECTION('',(0.,-1.,0.));
#13172=DIRECTION('center_axis',(3.95187814714554E-13,3.12137463243106E-13,
-1.));
#13173=DIRECTION('ref_axis',(0.999999999999951,3.13109078086861E-7,3.95643242527955E-13));
#13174=DIRECTION('',(1.,0.,0.));
#13175=DIRECTION('',(0.,-1.,0.));
#13176=DIRECTION('',(-1.,0.,0.));
#13177=DIRECTION('center_axis',(2.78474182098387E-15,-2.78474295664464E-15,
-1.));
#13178=DIRECTION('ref_axis',(-5.9452945013776E-7,-0.999999999999823,2.30695830588665E-15));
#13179=DIRECTION('',(0.,-1.,0.));
#13180=DIRECTION('',(0.,1.,0.));
#13181=DIRECTION('center_axis',(0.,0.,1.));
#13182=DIRECTION('ref_axis',(1.,0.,0.));
#13183=DIRECTION('',(1.,0.,0.));
#13184=DIRECTION('',(0.,-1.,0.));
#13185=DIRECTION('center_axis',(0.,0.,1.));
#13186=DIRECTION('ref_axis',(1.,0.,0.));
#13187=DIRECTION('',(-0.562310021407171,0.826926502069602,0.));
#13188=DIRECTION('',(1.,0.,0.));
#13189=DIRECTION('',(0.,-1.,0.));
#13190=DIRECTION('center_axis',(1.,0.,0.));
#13191=DIRECTION('ref_axis',(0.,0.,-1.));
#13192=DIRECTION('',(0.,0.,1.));
#13193=DIRECTION('',(0.,-1.,0.));
#13194=DIRECTION('',(0.,-1.,0.));
#13195=DIRECTION('',(0.,0.,-1.));
#13196=DIRECTION('',(0.,1.,0.));
#13197=DIRECTION('',(0.,0.,-1.));
#13198=DIRECTION('',(0.,-1.,0.));
#13199=DIRECTION('',(0.,0.,-1.));
#13200=DIRECTION('',(0.,1.,0.));
#13201=DIRECTION('',(0.,1.,0.));
#13202=DIRECTION('',(0.,0.,1.));
#13203=DIRECTION('',(0.,1.,0.));
#13204=DIRECTION('',(0.,0.,1.));
#13205=DIRECTION('',(0.,1.,0.));
#13206=DIRECTION('',(0.,0.,-1.));
#13207=DIRECTION('',(0.,1.,0.));
#13208=DIRECTION('',(0.,0.,-1.));
#13209=DIRECTION('',(0.,1.,0.));
#13210=DIRECTION('',(0.,1.,0.));
#13211=DIRECTION('',(0.,1.,0.));
#13212=DIRECTION('',(0.,0.,-1.));
#13213=DIRECTION('',(0.,1.,0.));
#13214=DIRECTION('',(0.,0.,1.));
#13215=DIRECTION('',(0.,1.,0.));
#13216=DIRECTION('',(0.,1.,0.));
#13217=DIRECTION('',(0.,1.,0.));
#13218=DIRECTION('',(0.,0.,-1.));
#13219=DIRECTION('',(0.,0.,-1.));
#13220=DIRECTION('',(0.,-1.,0.));
#13221=DIRECTION('',(0.,-1.,0.));
#13222=DIRECTION('',(0.,-1.,0.));
#13223=DIRECTION('',(0.,0.,1.));
#13224=DIRECTION('',(0.,-1.,0.));
#13225=DIRECTION('',(0.,0.,-1.));
#13226=DIRECTION('',(0.,-1.,0.));
#13227=DIRECTION('',(0.,-1.,0.));
#13228=DIRECTION('',(0.,-1.,0.));
#13229=DIRECTION('center_axis',(0.826926502069509,0.562310021407307,0.));
#13230=DIRECTION('ref_axis',(-0.562310021407307,0.826926502069509,0.));
#13231=DIRECTION('',(0.,0.,-1.));
#13232=DIRECTION('',(0.562310021410592,-0.826926502067275,0.));
#13233=DIRECTION('',(0.,0.,-1.));
#13234=DIRECTION('',(-0.562310021407307,0.826926502069509,0.));
#13235=DIRECTION('',(0.,0.,1.));
#13236=DIRECTION('center_axis',(1.,0.,0.));
#13237=DIRECTION('ref_axis',(0.,0.,-1.));
#13238=DIRECTION('',(0.,0.,1.));
#13239=DIRECTION('',(0.,1.,0.));
#13240=DIRECTION('',(0.,0.,1.));
#13241=DIRECTION('',(0.,0.,-1.));
#13242=DIRECTION('',(0.,1.,0.));
#13243=DIRECTION('',(0.,0.,-1.));
#13244=DIRECTION('',(0.,1.,0.));
#13245=DIRECTION('',(0.,0.,1.));
#13246=DIRECTION('',(0.,1.,0.));
#13247=DIRECTION('',(0.,0.,-1.));
#13248=DIRECTION('',(0.,1.,0.));
#13249=DIRECTION('',(0.,0.,1.));
#13250=DIRECTION('',(0.,1.,0.));
#13251=DIRECTION('',(0.,0.,-1.));
#13252=DIRECTION('',(0.,1.,0.));
#13253=DIRECTION('center_axis',(0.,0.,-1.));
#13254=DIRECTION('ref_axis',(-1.,0.,0.));
#13255=DIRECTION('',(0.,0.,-1.));
#13256=DIRECTION('center_axis',(0.,0.,1.));
#13257=DIRECTION('ref_axis',(-1.,4.62592926927149E-15,0.));
#13258=DIRECTION('center_axis',(0.826926502069509,-0.562310021407307,0.));
#13259=DIRECTION('ref_axis',(0.562310021407307,0.826926502069509,0.));
#13260=DIRECTION('',(0.,0.,-1.));
#13261=DIRECTION('',(0.562310021407307,0.826926502069509,0.));
#13262=DIRECTION('center_axis',(0.,0.,-1.));
#13263=DIRECTION('ref_axis',(-1.,0.,0.));
#13264=DIRECTION('',(0.,0.,-1.));
#13265=DIRECTION('center_axis',(0.,0.,1.));
#13266=DIRECTION('ref_axis',(-1.,0.,0.));
#13267=DIRECTION('center_axis',(0.,0.,1.));
#13268=DIRECTION('ref_axis',(-1.,-2.31296463463574E-15,0.));
#13269=DIRECTION('center_axis',(0.,0.,1.));
#13270=DIRECTION('ref_axis',(-1.,4.62592926927148E-15,0.));
#13271=DIRECTION('center_axis',(0.,-1.,0.));
#13272=DIRECTION('ref_axis',(0.,0.,-1.));
#13273=DIRECTION('',(0.,0.,1.));
#13274=DIRECTION('',(1.,0.,0.));
#13275=DIRECTION('',(0.,0.,-1.));
#13276=DIRECTION('',(1.,0.,0.));
#13277=DIRECTION('',(0.,0.,-1.));
#13278=DIRECTION('',(1.,0.,0.));
#13279=DIRECTION('',(0.,0.,1.));
#13280=DIRECTION('',(1.,0.,0.));
#13281=DIRECTION('',(0.,0.,-1.));
#13282=DIRECTION('',(1.,0.,0.));
#13283=DIRECTION('center_axis',(0.,0.,-1.));
#13284=DIRECTION('ref_axis',(-1.,0.,0.));
#13285=DIRECTION('',(0.,0.,-1.));
#13286=DIRECTION('center_axis',(0.,0.,1.));
#13287=DIRECTION('ref_axis',(-1.,0.,0.));
#13288=DIRECTION('center_axis',(0.,0.,1.));
#13289=DIRECTION('ref_axis',(-1.,0.,0.));
#13290=DIRECTION('center_axis',(0.,0.,1.));
#13291=DIRECTION('ref_axis',(-1.,0.,0.));
#13292=DIRECTION('center_axis',(-0.826926502069509,-0.562310021407307,0.));
#13293=DIRECTION('ref_axis',(0.562310021407307,-0.826926502069509,0.));
#13294=DIRECTION('',(0.,0.,-1.));
#13295=DIRECTION('',(0.562310021407307,-0.826926502069509,0.));
#13296=DIRECTION('center_axis',(0.,0.,-1.));
#13297=DIRECTION('ref_axis',(-1.,0.,0.));
#13298=DIRECTION('',(0.,0.,-1.));
#13299=DIRECTION('center_axis',(0.,0.,1.));
#13300=DIRECTION('ref_axis',(-1.,0.,0.));
#13301=DIRECTION('center_axis',(-1.,0.,0.));
#13302=DIRECTION('ref_axis',(0.,0.,1.));
#13303=DIRECTION('',(0.,0.,1.));
#13304=DIRECTION('',(0.,-1.,0.));
#13305=DIRECTION('',(0.,0.,-1.));
#13306=DIRECTION('',(0.,-1.,0.));
#13307=DIRECTION('',(0.,0.,-1.));
#13308=DIRECTION('',(0.,-1.,0.));
#13309=DIRECTION('',(0.,0.,1.));
#13310=DIRECTION('',(0.,-1.,0.));
#13311=DIRECTION('',(0.,0.,-1.));
#13312=DIRECTION('',(0.,-1.,0.));
#13313=DIRECTION('',(0.,0.,1.));
#13314=DIRECTION('',(0.,-1.,0.));
#13315=DIRECTION('',(0.,0.,-1.));
#13316=DIRECTION('',(0.,-1.,0.));
#13317=DIRECTION('center_axis',(0.,0.,-1.));
#13318=DIRECTION('ref_axis',(-1.,0.,0.));
#13319=DIRECTION('center_axis',(0.,0.,1.));
#13320=DIRECTION('ref_axis',(-1.,5.20417042793042E-15,0.));
#13321=DIRECTION('center_axis',(0.,0.,-1.));
#13322=DIRECTION('ref_axis',(-1.,0.,0.));
#13323=DIRECTION('center_axis',(0.,0.,1.));
#13324=DIRECTION('ref_axis',(-1.,1.73472347597681E-15,0.));
#13325=DIRECTION('center_axis',(0.,1.,0.));
#13326=DIRECTION('ref_axis',(0.,0.,1.));
#13327=DIRECTION('',(-1.,0.,0.));
#13328=DIRECTION('',(0.,0.,-1.));
#13329=DIRECTION('',(1.,0.,0.));
#13330=DIRECTION('center_axis',(0.,0.,1.));
#13331=DIRECTION('ref_axis',(1.,0.,0.));
#13332=DIRECTION('',(-1.,0.,0.));
#13333=DIRECTION('',(0.50000000000116,-0.866025403783769,0.));
#13334=DIRECTION('center_axis',(0.,1.,0.));
#13335=DIRECTION('ref_axis',(0.,0.,1.));
#13336=DIRECTION('center_axis',(0.,-1.,0.));
#13337=DIRECTION('ref_axis',(0.,0.,-1.));
#13338=DIRECTION('',(1.,0.,0.));
#13339=DIRECTION('',(0.,0.,1.));
#13340=DIRECTION('',(-1.,0.,0.));
#13341=DIRECTION('center_axis',(0.,0.,1.));
#13342=DIRECTION('ref_axis',(1.,0.,0.));
#13343=DIRECTION('',(0.866025403783496,0.500000000001632,0.));
#13344=DIRECTION('',(0.,1.,0.));
#13345=DIRECTION('center_axis',(0.,0.,-1.));
#13346=DIRECTION('ref_axis',(-1.,0.,0.));
#13347=DIRECTION('',(-1.,0.,0.));
#13348=DIRECTION('center_axis',(0.,0.,-1.));
#13349=DIRECTION('ref_axis',(-1.,0.,0.));
#13350=DIRECTION('',(0.,0.,1.));
#13351=DIRECTION('center_axis',(0.,0.,1.));
#13352=DIRECTION('ref_axis',(-1.,-3.46944695195361E-15,0.));
#13353=DIRECTION('center_axis',(0.,0.,1.));
#13354=DIRECTION('ref_axis',(1.,0.,0.));
#13355=DIRECTION('',(-1.,0.,0.));
#13356=DIRECTION('',(1.,0.,0.));
#13357=DIRECTION('',(0.,1.,0.));
#13358=DIRECTION('',(0.866025403783496,0.500000000001632,0.));
#13359=DIRECTION('center_axis',(0.,1.,0.));
#13360=DIRECTION('ref_axis',(0.,0.,1.));
#13361=DIRECTION('',(0.,0.,-1.));
#13362=DIRECTION('',(-1.,0.,0.));
#13363=DIRECTION('center_axis',(0.,0.,1.));
#13364=DIRECTION('ref_axis',(1.,0.,0.));
#13365=DIRECTION('center_axis',(0.,0.,1.));
#13366=DIRECTION('ref_axis',(1.,0.,0.));
#13367=DIRECTION('',(-1.,0.,0.));
#13368=DIRECTION('',(0.,1.,0.));
#13369=DIRECTION('',(-1.,0.,0.));
#13370=DIRECTION('center_axis',(0.,-1.,0.));
#13371=DIRECTION('ref_axis',(0.,0.,-1.));
#13372=DIRECTION('',(0.,0.,-1.));
#13373=DIRECTION('',(-1.,0.,0.));
#13374=DIRECTION('center_axis',(0.,-1.,0.));
#13375=DIRECTION('ref_axis',(0.,0.,-1.));
#13376=DIRECTION('',(-1.,0.,0.));
#13377=DIRECTION('',(0.,0.,1.));
#13378=DIRECTION('',(1.,0.,0.));
#13379=DIRECTION('center_axis',(0.,0.,1.));
#13380=DIRECTION('ref_axis',(1.,0.,0.));
#13381=DIRECTION('',(-1.,0.,0.));
#13382=DIRECTION('',(0.,1.,0.));
#13383=DIRECTION('center_axis',(0.,1.,0.));
#13384=DIRECTION('ref_axis',(0.,0.,1.));
#13385=DIRECTION('',(0.,0.,-1.));
#13386=DIRECTION('',(-1.,0.,0.));
#13387=DIRECTION('center_axis',(0.,1.,0.));
#13388=DIRECTION('ref_axis',(0.,0.,1.));
#13389=DIRECTION('',(0.,0.,1.));
#13390=DIRECTION('',(1.,0.,0.));
#13391=DIRECTION('',(-1.,0.,0.));
#13392=DIRECTION('center_axis',(0.,0.,1.));
#13393=DIRECTION('ref_axis',(1.,0.,0.));
#13394=DIRECTION('',(1.,0.,0.));
#13395=DIRECTION('',(0.,1.,0.));
#13396=DIRECTION('',(-0.500000000001634,-0.866025403783495,0.));
#13397=DIRECTION('',(-1.,0.,0.));
#13398=DIRECTION('center_axis',(0.,0.,-1.));
#13399=DIRECTION('ref_axis',(-1.,0.,0.));
#13400=DIRECTION('',(-0.500000000000017,0.866025403784429,0.));
#13401=DIRECTION('',(-0.499999999998097,-0.866025403785537,0.));
#13402=DIRECTION('center_axis',(0.,0.,1.));
#13403=DIRECTION('ref_axis',(1.,0.,0.));
#13404=DIRECTION('',(-1.,0.,0.));
#13405=DIRECTION('',(1.,0.,0.));
#13406=DIRECTION('',(0.500000000001634,-0.866025403783495,0.));
#13407=DIRECTION('center_axis',(0.,-1.,0.));
#13408=DIRECTION('ref_axis',(0.,0.,-1.));
#13409=DIRECTION('',(1.,0.,0.));
#13410=DIRECTION('center_axis',(0.,0.,1.));
#13411=DIRECTION('ref_axis',(1.,0.,0.));
#13412=DIRECTION('',(-1.,0.,0.));
#13413=DIRECTION('center_axis',(0.,1.,0.));
#13414=DIRECTION('ref_axis',(0.,0.,1.));
#13415=DIRECTION('',(1.,0.,0.));
#13416=DIRECTION('center_axis',(0.,0.,1.));
#13417=DIRECTION('ref_axis',(1.,0.,0.));
#13418=DIRECTION('',(-0.50000000000116,-0.866025403783769,0.));
#13419=DIRECTION('',(-1.,0.,0.));
#13420=DIRECTION('center_axis',(0.,0.,-1.));
#13421=DIRECTION('ref_axis',(-1.,0.,0.));
#13422=DIRECTION('',(-0.500000000000017,0.866025403784429,0.));
#13423=DIRECTION('',(-0.500000000009312,-0.866025403779062,0.));
#13424=DIRECTION('center_axis',(0.,0.,1.));
#13425=DIRECTION('ref_axis',(1.,0.,0.));
#13426=DIRECTION('',(-1.,0.,0.));
#13427=DIRECTION('',(1.,0.,0.));
#13428=DIRECTION('',(0.50000000000116,-0.866025403783769,0.));
#13429=DIRECTION('center_axis',(0.,-1.,0.));
#13430=DIRECTION('ref_axis',(0.,0.,-1.));
#13431=DIRECTION('center_axis',(0.,0.,-1.));
#13432=DIRECTION('ref_axis',(-1.,0.,0.));
#13433=DIRECTION('',(0.500000000000017,0.866025403784429,0.));
#13434=DIRECTION('',(0.500000000009309,-0.866025403779064,0.));
#13435=DIRECTION('center_axis',(0.,0.,1.));
#13436=DIRECTION('ref_axis',(1.,0.,0.));
#13437=DIRECTION('',(1.,0.,0.));
#13438=DIRECTION('',(-1.,0.,0.));
#13439=DIRECTION('',(-0.50000000000116,-0.866025403783769,0.));
#13440=DIRECTION('center_axis',(0.,-1.,0.));
#13441=DIRECTION('ref_axis',(0.,0.,-1.));
#13442=DIRECTION('',(-1.,0.,0.));
#13443=DIRECTION('center_axis',(0.,0.,1.));
#13444=DIRECTION('ref_axis',(1.,0.,0.));
#13445=DIRECTION('',(1.,0.,0.));
#13446=DIRECTION('center_axis',(0.,1.,0.));
#13447=DIRECTION('ref_axis',(0.,0.,1.));
#13448=DIRECTION('',(-1.,0.,0.));
#13449=DIRECTION('center_axis',(0.,0.,1.));
#13450=DIRECTION('ref_axis',(1.,0.,0.));
#13451=DIRECTION('',(0.500000000001634,-0.866025403783495,0.));
#13452=DIRECTION('',(1.,0.,0.));
#13453=DIRECTION('center_axis',(0.,0.,-1.));
#13454=DIRECTION('ref_axis',(-1.,0.,0.));
#13455=DIRECTION('',(0.500000000000017,0.866025403784429,0.));
#13456=DIRECTION('',(0.499999999998084,-0.866025403785545,0.));
#13457=DIRECTION('center_axis',(0.,0.,1.));
#13458=DIRECTION('ref_axis',(1.,0.,0.));
#13459=DIRECTION('',(1.,0.,0.));
#13460=DIRECTION('',(-1.,0.,0.));
#13461=DIRECTION('',(-0.500000000001634,-0.866025403783495,0.));
#13462=DIRECTION('center_axis',(0.,-1.,0.));
#13463=DIRECTION('ref_axis',(0.,0.,-1.));
#13464=DIRECTION('',(-1.,0.,0.));
#13465=DIRECTION('center_axis',(0.,0.,1.));
#13466=DIRECTION('ref_axis',(1.,0.,0.));
#13467=DIRECTION('center_axis',(0.,0.,1.));
#13468=DIRECTION('ref_axis',(1.,0.,0.));
#13469=DIRECTION('center_axis',(0.,-1.,0.));
#13470=DIRECTION('ref_axis',(0.,0.,-1.));
#13471=DIRECTION('',(0.,0.,1.));
#13472=DIRECTION('',(1.,0.,0.));
#13473=DIRECTION('center_axis',(0.,0.,-1.));
#13474=DIRECTION('ref_axis',(-1.,0.,0.));
#13475=DIRECTION('',(0.,-1.,0.));
#13476=DIRECTION('',(0.866025403783581,-0.500000000001486,0.));
#13477=DIRECTION('',(0.86602540378358,0.500000000001487,0.));
#13478=DIRECTION('',(0.,1.,0.));
#13479=DIRECTION('center_axis',(0.,0.,-1.));
#13480=DIRECTION('ref_axis',(-1.,0.,0.));
#13481=DIRECTION('',(1.,0.,0.));
#13482=DIRECTION('',(0.50000000000149,0.866025403783578,0.));
#13483=DIRECTION('',(-0.500000000001491,0.866025403783578,0.));
#13484=DIRECTION('',(-1.,0.,0.));
#13485=DIRECTION('center_axis',(0.,0.,-1.));
#13486=DIRECTION('ref_axis',(-1.,0.,0.));
#13487=DIRECTION('',(1.,0.,0.));
#13488=DIRECTION('',(0.50000000000149,0.866025403783578,0.));
#13489=DIRECTION('',(-0.50000000000149,0.866025403783578,0.));
#13490=DIRECTION('',(-1.,0.,0.));
#13491=DIRECTION('center_axis',(0.,0.,-1.));
#13492=DIRECTION('ref_axis',(-1.,0.,0.));
#13493=DIRECTION('',(0.,-1.,0.));
#13494=DIRECTION('',(0.86602540378358,-0.500000000001487,0.));
#13495=DIRECTION('',(0.866025403783581,0.500000000001486,0.));
#13496=DIRECTION('',(0.,1.,0.));
#13497=DIRECTION('center_axis',(0.,0.,-1.));
#13498=DIRECTION('ref_axis',(-1.,0.,0.));
#13499=DIRECTION('',(-1.,0.,0.));
#13500=DIRECTION('',(-0.500000000001491,-0.866025403783578,0.));
#13501=DIRECTION('',(0.50000000000149,-0.866025403783578,0.));
#13502=DIRECTION('',(1.,0.,0.));
#13503=DIRECTION('center_axis',(0.,0.,-1.));
#13504=DIRECTION('ref_axis',(-1.,0.,0.));
#13505=DIRECTION('',(-1.,0.,0.));
#13506=DIRECTION('',(-0.50000000000149,-0.866025403783578,0.));
#13507=DIRECTION('',(0.50000000000149,-0.866025403783578,0.));
#13508=DIRECTION('center_axis',(0.,1.,0.));
#13509=DIRECTION('ref_axis',(0.,0.,1.));
#13510=DIRECTION('',(0.,0.,1.));
#13511=DIRECTION('',(1.,0.,0.));
#13512=DIRECTION('center_axis',(0.,1.,0.));
#13513=DIRECTION('ref_axis',(0.,0.,1.));
#13514=DIRECTION('',(-1.,0.,0.));
#13515=DIRECTION('',(1.,0.,0.));
#13516=DIRECTION('center_axis',(0.,0.,1.));
#13517=DIRECTION('ref_axis',(1.,0.,0.));
#13518=DIRECTION('',(1.,0.,0.));
#13519=DIRECTION('center_axis',(0.,-1.,0.));
#13520=DIRECTION('ref_axis',(0.,0.,-1.));
#13521=DIRECTION('',(-1.,0.,0.));
#13522=DIRECTION('center_axis',(0.,-1.,0.));
#13523=DIRECTION('ref_axis',(0.,0.,-1.));
#13524=DIRECTION('',(0.,0.,-1.));
#13525=DIRECTION('',(-1.,0.,0.));
#13526=DIRECTION('center_axis',(0.,1.,0.));
#13527=DIRECTION('ref_axis',(0.,0.,1.));
#13528=DIRECTION('',(0.,0.,1.));
#13529=DIRECTION('',(1.,0.,0.));
#13530=DIRECTION('center_axis',(0.,1.,0.));
#13531=DIRECTION('ref_axis',(0.,0.,1.));
#13532=DIRECTION('',(-1.,0.,0.));
#13533=DIRECTION('',(1.,0.,0.));
#13534=DIRECTION('',(0.,0.,1.));
#13535=DIRECTION('center_axis',(0.,0.,1.));
#13536=DIRECTION('ref_axis',(1.,0.,0.));
#13537=DIRECTION('',(0.,-1.,0.));
#13538=DIRECTION('',(-1.,0.,0.));
#13539=DIRECTION('center_axis',(0.,0.,1.));
#13540=DIRECTION('ref_axis',(1.,0.,0.));
#13541=DIRECTION('',(1.,0.,0.));
#13542=DIRECTION('center_axis',(1.,0.,0.));
#13543=DIRECTION('ref_axis',(0.,0.,-1.));
#13544=DIRECTION('',(0.,0.,1.));
#13545=DIRECTION('',(0.,-1.,0.));
#13546=DIRECTION('center_axis',(1.,0.,0.));
#13547=DIRECTION('ref_axis',(0.,0.,-1.));
#13548=DIRECTION('',(0.,1.,0.));
#13549=DIRECTION('',(0.,-1.,0.));
#13550=DIRECTION('',(0.,0.,1.));
#13551=DIRECTION('center_axis',(0.,0.,1.));
#13552=DIRECTION('ref_axis',(1.,0.,0.));
#13553=DIRECTION('',(0.,-1.,0.));
#13554=DIRECTION('',(-1.,0.,0.));
#13555=DIRECTION('center_axis',(-1.,0.,0.));
#13556=DIRECTION('ref_axis',(0.,0.,1.));
#13557=DIRECTION('',(0.,1.,0.));
#13558=DIRECTION('',(0.,0.,-1.));
#13559=DIRECTION('center_axis',(-1.,0.,0.));
#13560=DIRECTION('ref_axis',(0.,0.,1.));
#13561=DIRECTION('',(0.,0.,-1.));
#13562=DIRECTION('',(0.,1.,0.));
#13563=DIRECTION('center_axis',(0.,1.,0.));
#13564=DIRECTION('ref_axis',(0.,0.,1.));
#13565=DIRECTION('',(0.,0.,-1.));
#13566=DIRECTION('center_axis',(0.,1.,0.));
#13567=DIRECTION('ref_axis',(0.,0.,1.));
#13568=DIRECTION('',(0.,0.,-1.));
#13569=DIRECTION('center_axis',(0.,-1.,0.));
#13570=DIRECTION('ref_axis',(0.,0.,-1.));
#13571=DIRECTION('',(0.,0.,1.));
#13572=DIRECTION('center_axis',(0.,1.,0.));
#13573=DIRECTION('ref_axis',(0.,0.,1.));
#13574=DIRECTION('',(0.,0.,-1.));
#13575=DIRECTION('center_axis',(0.,1.,0.));
#13576=DIRECTION('ref_axis',(0.,0.,1.));
#13577=DIRECTION('center_axis',(0.,1.,0.));
#13578=DIRECTION('ref_axis',(0.,0.,1.));
#13579=DIRECTION('center_axis',(1.63914506158791E-15,-4.24321088898506E-15,
-1.));
#13580=DIRECTION('ref_axis',(0.707106781281055,-0.70710678109204,4.64841042086043E-15));
#13581=DIRECTION('center_axis',(1.,1.83697019872103E-16,0.));
#13582=DIRECTION('ref_axis',(1.83697019872103E-16,-1.,0.));
#13583=DIRECTION('center_axis',(1.,0.,0.));
#13584=DIRECTION('ref_axis',(0.,0.,-1.));
#13585=DIRECTION('center_axis',(1.,0.,0.));
#13586=DIRECTION('ref_axis',(0.,0.,-1.));
#13587=DIRECTION('center_axis',(0.,1.,0.));
#13588=DIRECTION('ref_axis',(0.,0.,1.));
#13589=DIRECTION('center_axis',(0.,-1.,0.));
#13590=DIRECTION('ref_axis',(0.,0.,1.));
#13591=DIRECTION('center_axis',(0.,1.,0.));
#13592=DIRECTION('ref_axis',(0.,0.,1.));
#13593=DIRECTION('center_axis',(-1.,0.,0.));
#13594=DIRECTION('ref_axis',(0.,0.,1.));
#13595=DIRECTION('center_axis',(-1.,0.,0.));
#13596=DIRECTION('ref_axis',(0.,0.,1.));
#13597=DIRECTION('center_axis',(1.,0.,0.));
#13598=DIRECTION('ref_axis',(0.,0.,1.));
#13599=DIRECTION('center_axis',(1.48434289583302E-14,1.42898708586572E-14,
-1.));
#13600=DIRECTION('ref_axis',(0.707106781236163,0.707106781136932,2.0585817578096E-14));
#13601=DIRECTION('center_axis',(1.40259237217524E-10,1.,0.));
#13602=DIRECTION('ref_axis',(1.,-1.40259237217524E-10,0.));
#13603=DIRECTION('center_axis',(0.,1.,0.));
#13604=DIRECTION('ref_axis',(0.,0.,1.));
#13605=DIRECTION('center_axis',(0.,1.,0.));
#13606=DIRECTION('ref_axis',(0.,0.,1.));
#13607=DIRECTION('center_axis',(-1.,0.,0.));
#13608=DIRECTION('ref_axis',(0.,0.,1.));
#13609=DIRECTION('center_axis',(1.,0.,0.));
#13610=DIRECTION('ref_axis',(0.,0.,1.));
#13611=DIRECTION('center_axis',(-1.,0.,0.));
#13612=DIRECTION('ref_axis',(0.,0.,1.));
#13613=DIRECTION('center_axis',(0.,-1.,0.));
#13614=DIRECTION('ref_axis',(0.,0.,-1.));
#13615=DIRECTION('center_axis',(0.,-1.,0.));
#13616=DIRECTION('ref_axis',(0.,0.,-1.));
#13617=DIRECTION('center_axis',(0.,1.,0.));
#13618=DIRECTION('ref_axis',(0.,0.,-1.));
#13619=DIRECTION('center_axis',(1.17155445946046E-15,-2.64224536130632E-16,
-1.));
#13620=DIRECTION('ref_axis',(-1.,0.,-6.64058631551495E-16));
#13621=DIRECTION('center_axis',(-1.,1.40259742539074E-10,0.));
#13622=DIRECTION('ref_axis',(1.40259742539074E-10,1.,0.));
#13623=DIRECTION('center_axis',(-1.,0.,0.));
#13624=DIRECTION('ref_axis',(0.,0.,1.));
#13625=DIRECTION('center_axis',(-1.,0.,0.));
#13626=DIRECTION('ref_axis',(0.,0.,1.));
#13627=DIRECTION('center_axis',(0.,-1.,0.));
#13628=DIRECTION('ref_axis',(0.,0.,-1.));
#13629=DIRECTION('center_axis',(0.,1.,0.));
#13630=DIRECTION('ref_axis',(0.,0.,-1.));
#13631=DIRECTION('center_axis',(0.,-1.,0.));
#13632=DIRECTION('ref_axis',(0.,0.,-1.));
#13633=DIRECTION('center_axis',(1.,0.,0.));
#13634=DIRECTION('ref_axis',(0.,0.,-1.));
#13635=DIRECTION('center_axis',(1.,0.,0.));
#13636=DIRECTION('ref_axis',(0.,0.,-1.));
#13637=DIRECTION('center_axis',(-1.,0.,0.));
#13638=DIRECTION('ref_axis',(0.,0.,-1.));
#13639=DIRECTION('center_axis',(0.,0.,-1.));
#13640=DIRECTION('ref_axis',(-1.,0.,0.));
#13641=DIRECTION('center_axis',(0.,-1.,0.));
#13642=DIRECTION('ref_axis',(-1.,0.,0.));
#13643=DIRECTION('center_axis',(0.,-1.,0.));
#13644=DIRECTION('ref_axis',(0.,0.,-1.));
#13645=DIRECTION('center_axis',(0.,-1.,0.));
#13646=DIRECTION('ref_axis',(0.,0.,-1.));
#13647=DIRECTION('',(-1.,0.,0.));
#13648=DIRECTION('center_axis',(0.,0.,1.));
#13649=DIRECTION('ref_axis',(1.,0.,0.));
#13650=DIRECTION('',(0.50000000000116,0.866025403783769,0.));
#13651=DIRECTION('',(1.,0.,0.));
#13652=DIRECTION('center_axis',(0.,-1.,0.));
#13653=DIRECTION('ref_axis',(0.,0.,-1.));
#13654=DIRECTION('',(0.,0.,-1.));
#13655=DIRECTION('center_axis',(0.,1.,0.));
#13656=DIRECTION('ref_axis',(0.,0.,1.));
#13657=DIRECTION('',(-1.,0.,0.));
#13658=DIRECTION('center_axis',(0.,0.,1.));
#13659=DIRECTION('ref_axis',(1.,0.,0.));
#13660=DIRECTION('',(-1.,0.,0.));
#13661=DIRECTION('center_axis',(0.,-1.,0.));
#13662=DIRECTION('ref_axis',(0.,0.,-1.));
#13663=DIRECTION('',(1.,0.,0.));
#13664=DIRECTION('center_axis',(0.,0.,1.));
#13665=DIRECTION('ref_axis',(1.,0.,0.));
#13666=DIRECTION('',(-0.500000000001634,0.866025403783495,0.));
#13667=DIRECTION('',(-1.,0.,0.));
#13668=DIRECTION('center_axis',(0.,0.,-1.));
#13669=DIRECTION('ref_axis',(-1.,0.,0.));
#13670=DIRECTION('',(-0.500000000000017,-0.866025403784429,0.));
#13671=DIRECTION('',(-0.499999999998097,0.866025403785537,0.));
#13672=DIRECTION('center_axis',(0.,0.,1.));
#13673=DIRECTION('ref_axis',(1.,0.,0.));
#13674=DIRECTION('',(-1.,0.,0.));
#13675=DIRECTION('',(1.,0.,0.));
#13676=DIRECTION('',(0.500000000001634,0.866025403783495,0.));
#13677=DIRECTION('center_axis',(0.,1.,0.));
#13678=DIRECTION('ref_axis',(0.,0.,1.));
#13679=DIRECTION('',(1.,0.,0.));
#13680=DIRECTION('center_axis',(0.,0.,1.));
#13681=DIRECTION('ref_axis',(1.,0.,0.));
#13682=DIRECTION('',(-1.,0.,0.));
#13683=DIRECTION('center_axis',(0.,-1.,0.));
#13684=DIRECTION('ref_axis',(0.,0.,-1.));
#13685=DIRECTION('',(1.,0.,0.));
#13686=DIRECTION('center_axis',(0.,0.,1.));
#13687=DIRECTION('ref_axis',(1.,0.,0.));
#13688=DIRECTION('',(-0.50000000000116,0.866025403783769,0.));
#13689=DIRECTION('',(-1.,0.,0.));
#13690=DIRECTION('center_axis',(0.,0.,-1.));
#13691=DIRECTION('ref_axis',(-1.,0.,0.));
#13692=DIRECTION('',(-0.500000000000017,-0.866025403784429,0.));
#13693=DIRECTION('',(-0.500000000009312,0.866025403779062,0.));
#13694=DIRECTION('center_axis',(0.,0.,1.));
#13695=DIRECTION('ref_axis',(1.,0.,0.));
#13696=DIRECTION('',(1.,0.,0.));
#13697=DIRECTION('',(0.50000000000116,0.866025403783769,0.));
#13698=DIRECTION('center_axis',(0.,0.,-1.));
#13699=DIRECTION('ref_axis',(-1.,0.,0.));
#13700=DIRECTION('',(-0.500000000009312,0.866025403779062,0.));
#13701=DIRECTION('',(0.500000000009309,0.866025403779064,0.));
#13702=DIRECTION('center_axis',(0.,0.,1.));
#13703=DIRECTION('ref_axis',(1.,0.,0.));
#13704=DIRECTION('',(-0.50000000000116,0.866025403783769,0.));
#13705=DIRECTION('center_axis',(0.,0.,1.));
#13706=DIRECTION('ref_axis',(1.,0.,0.));
#13707=DIRECTION('',(0.500000000001634,0.866025403783495,0.));
#13708=DIRECTION('center_axis',(0.,0.,-1.));
#13709=DIRECTION('ref_axis',(-1.,0.,0.));
#13710=DIRECTION('',(-0.499999999998097,0.866025403785537,0.));
#13711=DIRECTION('',(0.499999999998084,0.866025403785545,0.));
#13712=DIRECTION('center_axis',(0.,0.,1.));
#13713=DIRECTION('ref_axis',(1.,0.,0.));
#13714=DIRECTION('',(-0.500000000001634,0.866025403783495,0.));
#13715=DIRECTION('',(1.,0.,0.));
#13716=DIRECTION('',(0.,-1.,0.));
#13717=DIRECTION('center_axis',(0.,1.,0.));
#13718=DIRECTION('ref_axis',(0.,0.,1.));
#13719=DIRECTION('',(0.,0.,-1.));
#13720=DIRECTION('',(1.,0.,0.));
#13721=DIRECTION('center_axis',(0.,1.,0.));
#13722=DIRECTION('ref_axis',(0.,0.,1.));
#13723=DIRECTION('',(1.,0.,0.));
#13724=DIRECTION('',(0.,0.,1.));
#13725=DIRECTION('',(-1.,0.,0.));
#13726=DIRECTION('center_axis',(0.,0.,1.));
#13727=DIRECTION('ref_axis',(1.,0.,0.));
#13728=DIRECTION('',(1.,0.,0.));
#13729=DIRECTION('',(0.,-1.,0.));
#13730=DIRECTION('center_axis',(0.,-1.,0.));
#13731=DIRECTION('ref_axis',(0.,0.,-1.));
#13732=DIRECTION('',(0.,0.,-1.));
#13733=DIRECTION('',(1.,0.,0.));
#13734=DIRECTION('center_axis',(0.,-1.,0.));
#13735=DIRECTION('ref_axis',(0.,0.,-1.));
#13736=DIRECTION('',(0.,0.,1.));
#13737=DIRECTION('',(-1.,0.,0.));
#13738=DIRECTION('center_axis',(0.,1.,0.));
#13739=DIRECTION('ref_axis',(0.,0.,1.));
#13740=DIRECTION('',(1.,0.,0.));
#13741=DIRECTION('',(0.,0.,1.));
#13742=DIRECTION('center_axis',(0.,0.,1.));
#13743=DIRECTION('ref_axis',(1.,0.,0.));
#13744=DIRECTION('center_axis',(0.,0.,-1.));
#13745=DIRECTION('ref_axis',(-1.,0.,0.));
#13746=DIRECTION('',(-1.,0.,0.));
#13747=DIRECTION('',(0.866025403783496,-0.500000000001632,0.));
#13748=DIRECTION('',(0.,-1.,0.));
#13749=DIRECTION('center_axis',(0.,0.,-1.));
#13750=DIRECTION('ref_axis',(-1.,0.,0.));
#13751=DIRECTION('center_axis',(0.,0.,-1.));
#13752=DIRECTION('ref_axis',(-1.,0.,0.));
#13753=DIRECTION('',(0.,0.,-1.));
#13754=DIRECTION('center_axis',(0.,0.,1.));
#13755=DIRECTION('ref_axis',(1.,0.,0.));
#13756=DIRECTION('',(1.,0.,0.));
#13757=DIRECTION('',(0.,-1.,0.));
#13758=DIRECTION('',(0.866025403783496,-0.500000000001632,0.));
#13759=DIRECTION('',(-1.,0.,0.));
#13760=DIRECTION('center_axis',(0.,-1.,0.));
#13761=DIRECTION('ref_axis',(0.,0.,-1.));
#13762=DIRECTION('',(-1.,0.,0.));
#13763=DIRECTION('',(0.,0.,-1.));
#13764=DIRECTION('center_axis',(0.,0.,1.));
#13765=DIRECTION('ref_axis',(1.,0.,0.));
#13766=DIRECTION('center_axis',(0.,1.,0.));
#13767=DIRECTION('ref_axis',(0.,0.,1.));
#13768=DIRECTION('',(1.,0.,0.));
#13769=DIRECTION('',(0.,0.,1.));
#13770=DIRECTION('center_axis',(0.,0.,-1.));
#13771=DIRECTION('ref_axis',(-1.,0.,0.));
#13772=DIRECTION('',(0.,-1.,0.));
#13773=DIRECTION('',(0.,1.,0.));
#13774=DIRECTION('',(0.86602540378358,0.500000000001487,0.));
#13775=DIRECTION('',(0.866025403783581,-0.500000000001486,0.));
#13776=DIRECTION('center_axis',(0.,0.,-1.));
#13777=DIRECTION('ref_axis',(-1.,0.,0.));
#13778=DIRECTION('',(0.50000000000149,0.866025403783578,0.));
#13779=DIRECTION('',(1.,0.,0.));
#13780=DIRECTION('',(-1.,0.,0.));
#13781=DIRECTION('',(-0.500000000001491,0.866025403783578,0.));
#13782=DIRECTION('center_axis',(0.,0.,-1.));
#13783=DIRECTION('ref_axis',(-1.,0.,0.));
#13784=DIRECTION('',(-1.,0.,0.));
#13785=DIRECTION('',(-0.50000000000149,0.866025403783578,0.));
#13786=DIRECTION('',(0.50000000000149,0.866025403783578,0.));
#13787=DIRECTION('center_axis',(0.,0.,-1.));
#13788=DIRECTION('ref_axis',(-1.,0.,0.));
#13789=DIRECTION('',(0.,-1.,0.));
#13790=DIRECTION('',(0.,1.,0.));
#13791=DIRECTION('',(0.866025403783581,0.500000000001486,0.));
#13792=DIRECTION('',(0.86602540378358,-0.500000000001487,0.));
#13793=DIRECTION('center_axis',(0.,0.,-1.));
#13794=DIRECTION('ref_axis',(-1.,0.,0.));
#13795=DIRECTION('',(-0.500000000001491,-0.866025403783578,0.));
#13796=DIRECTION('',(-1.,0.,0.));
#13797=DIRECTION('',(1.,0.,0.));
#13798=DIRECTION('',(0.50000000000149,-0.866025403783578,0.));
#13799=DIRECTION('center_axis',(0.,0.,-1.));
#13800=DIRECTION('ref_axis',(-1.,0.,0.));
#13801=DIRECTION('',(-1.,0.,0.));
#13802=DIRECTION('',(0.50000000000149,-0.866025403783578,0.));
#13803=DIRECTION('',(-0.50000000000149,-0.866025403783578,0.));
#13804=DIRECTION('center_axis',(0.,-1.,0.));
#13805=DIRECTION('ref_axis',(0.,0.,-1.));
#13806=DIRECTION('',(0.,0.,-1.));
#13807=DIRECTION('center_axis',(0.,1.,0.));
#13808=DIRECTION('ref_axis',(0.,0.,1.));
#13809=DIRECTION('',(0.,0.,1.));
#13810=DIRECTION('center_axis',(0.,-1.,0.));
#13811=DIRECTION('ref_axis',(0.,0.,-1.));
#13812=DIRECTION('',(0.,0.,-1.));
#13813=DIRECTION('center_axis',(-1.,0.,0.));
#13814=DIRECTION('ref_axis',(0.,0.,1.));
#13815=DIRECTION('',(0.,-1.,0.));
#13816=DIRECTION('',(0.,0.,-1.));
#13817=DIRECTION('center_axis',(-1.,0.,0.));
#13818=DIRECTION('ref_axis',(0.,0.,1.));
#13819=DIRECTION('',(0.,1.,0.));
#13820=DIRECTION('',(0.,0.,-1.));
#13821=DIRECTION('',(0.,-1.,0.));
#13822=DIRECTION('center_axis',(0.,0.,1.));
#13823=DIRECTION('ref_axis',(1.,0.,0.));
#13824=DIRECTION('',(0.,-1.,0.));
#13825=DIRECTION('',(-1.,0.,0.));
#13826=DIRECTION('center_axis',(1.,0.,0.));
#13827=DIRECTION('ref_axis',(0.,0.,-1.));
#13828=DIRECTION('',(0.,1.,0.));
#13829=DIRECTION('',(0.,0.,1.));
#13830=DIRECTION('center_axis',(1.,0.,0.));
#13831=DIRECTION('ref_axis',(0.,0.,-1.));
#13832=DIRECTION('',(0.,0.,1.));
#13833=DIRECTION('',(0.,1.,0.));
#13834=DIRECTION('center_axis',(0.,-1.,0.));
#13835=DIRECTION('ref_axis',(0.,0.,-1.));
#13836=DIRECTION('',(0.,0.,1.));
#13837=DIRECTION('center_axis',(0.,1.,0.));
#13838=DIRECTION('ref_axis',(0.,0.,1.));
#13839=DIRECTION('',(0.,0.,-1.));
#13840=DIRECTION('center_axis',(0.,-1.,0.));
#13841=DIRECTION('ref_axis',(0.,0.,-1.));
#13842=DIRECTION('',(0.,0.,1.));
#13843=DIRECTION('center_axis',(0.,0.,-1.));
#13844=DIRECTION('ref_axis',(-1.,0.,0.));
#13845=DIRECTION('center_axis',(0.866025403784429,0.500000000000017,0.));
#13846=DIRECTION('ref_axis',(-0.500000000000017,0.866025403784429,0.));
#13847=DIRECTION('',(0.,0.,-1.));
#13848=DIRECTION('center_axis',(-1.,0.,0.));
#13849=DIRECTION('ref_axis',(0.,0.,1.));
#13850=DIRECTION('',(0.,0.,-1.));
#13851=DIRECTION('center_axis',(-0.500000000000017,0.866025403784429,0.));
#13852=DIRECTION('ref_axis',(-0.866025403784429,-0.500000000000017,0.));
#13853=DIRECTION('',(-0.866025403784429,-0.500000000000017,0.));
#13854=DIRECTION('',(0.,0.,-1.));
#13855=DIRECTION('center_axis',(0.,-1.,0.));
#13856=DIRECTION('ref_axis',(0.,0.,-1.));
#13857=DIRECTION('',(1.,0.,0.));
#13858=DIRECTION('',(-1.,0.,0.));
#13859=DIRECTION('',(-1.,0.,0.));
#13860=DIRECTION('',(-1.,0.,0.));
#13861=DIRECTION('',(-1.,0.,0.));
#13862=DIRECTION('',(1.,0.,0.));
#13863=DIRECTION('',(1.,0.,0.));
#13864=DIRECTION('',(1.,0.,0.));
#13865=DIRECTION('center_axis',(0.500000000000017,-0.866025403784429,0.));
#13866=DIRECTION('ref_axis',(0.866025403784429,0.500000000000017,0.));
#13867=DIRECTION('',(0.,0.,1.));
#13868=DIRECTION('',(-0.866025403784429,-0.500000000000017,0.));
#13869=DIRECTION('',(0.,0.,-1.));
#13870=DIRECTION('center_axis',(1.,0.,0.));
#13871=DIRECTION('ref_axis',(0.,0.,-1.));
#13872=DIRECTION('center_axis',(-1.,0.,0.));
#13873=DIRECTION('ref_axis',(0.,0.,1.));
#13874=DIRECTION('',(0.,1.,0.));
#13875=DIRECTION('center_axis',(0.,0.,-1.));
#13876=DIRECTION('ref_axis',(-1.,0.,0.));
#13877=DIRECTION('',(0.,-1.,0.));
#13878=DIRECTION('',(0.,1.,0.));
#13879=DIRECTION('',(1.,0.,0.));
#13880=DIRECTION('',(0.,-1.,0.));
#13881=DIRECTION('',(-1.,0.,0.));
#13882=DIRECTION('center_axis',(1.,0.,0.));
#13883=DIRECTION('ref_axis',(0.,0.,-1.));
#13884=DIRECTION('center_axis',(-0.866025403784429,0.500000000000017,0.));
#13885=DIRECTION('ref_axis',(-0.500000000000017,-0.866025403784429,0.));
#13886=DIRECTION('',(0.,0.,-1.));
#13887=DIRECTION('center_axis',(-0.866025403784429,-0.500000000000017,0.));
#13888=DIRECTION('ref_axis',(0.500000000000017,-0.866025403784429,0.));
#13889=DIRECTION('center_axis',(-0.866025403784429,0.500000000000017,0.));
#13890=DIRECTION('ref_axis',(-0.500000000000017,-0.866025403784429,0.));
#13891=DIRECTION('',(0.,0.,-1.));
#13892=DIRECTION('center_axis',(-0.866025403784429,-0.500000000000017,0.));
#13893=DIRECTION('ref_axis',(0.500000000000017,-0.866025403784429,0.));
#13894=DIRECTION('center_axis',(0.866025403784429,-0.500000000000017,0.));
#13895=DIRECTION('ref_axis',(0.500000000000017,0.866025403784429,0.));
#13896=DIRECTION('center_axis',(0.866025403784429,0.500000000000017,0.));
#13897=DIRECTION('ref_axis',(-0.500000000000017,0.866025403784429,0.));
#13898=DIRECTION('',(0.,0.,-1.));
#13899=DIRECTION('center_axis',(0.866025403784429,-0.500000000000017,0.));
#13900=DIRECTION('ref_axis',(0.500000000000017,0.866025403784429,0.));
#13901=DIRECTION('center_axis',(-1.,0.,0.));
#13902=DIRECTION('ref_axis',(0.,0.,1.));
#13903=DIRECTION('',(0.,0.,-1.));
#13904=DIRECTION('center_axis',(-0.500000000000017,-0.866025403784429,0.));
#13905=DIRECTION('ref_axis',(0.866025403784429,-0.500000000000017,0.));
#13906=DIRECTION('',(-0.866025403784429,0.500000000000017,0.));
#13907=DIRECTION('',(0.,0.,-1.));
#13908=DIRECTION('center_axis',(0.500000000000017,-0.866025403784429,0.));
#13909=DIRECTION('ref_axis',(0.866025403784429,0.500000000000017,0.));
#13910=DIRECTION('',(-0.866025403784429,-0.500000000000017,0.));
#13911=DIRECTION('',(-0.866025403784429,-0.500000000000017,0.));
#13912=DIRECTION('center_axis',(0.866025403784429,-0.500000000000017,0.));
#13913=DIRECTION('ref_axis',(0.500000000000017,0.866025403784429,0.));
#13914=DIRECTION('',(0.,0.,-1.));
#13915=DIRECTION('center_axis',(0.866025403784429,0.500000000000017,0.));
#13916=DIRECTION('ref_axis',(-0.500000000000017,0.866025403784429,0.));
#13917=DIRECTION('center_axis',(0.866025403784429,-0.500000000000017,0.));
#13918=DIRECTION('ref_axis',(0.500000000000017,0.866025403784429,0.));
#13919=DIRECTION('',(0.,0.,-1.));
#13920=DIRECTION('center_axis',(0.866025403784429,0.500000000000017,0.));
#13921=DIRECTION('ref_axis',(-0.500000000000017,0.866025403784429,0.));
#13922=DIRECTION('center_axis',(-0.500000000000017,-0.866025403784429,0.));
#13923=DIRECTION('ref_axis',(0.866025403784429,-0.500000000000017,0.));
#13924=DIRECTION('',(-0.866025403784429,0.500000000000017,0.));
#13925=DIRECTION('',(-0.866025403784429,0.500000000000017,0.));
#13926=DIRECTION('center_axis',(1.,0.,0.));
#13927=DIRECTION('ref_axis',(0.,0.,-1.));
#13928=DIRECTION('',(0.,-1.,0.));
#13929=DIRECTION('center_axis',(0.,0.,1.));
#13930=DIRECTION('ref_axis',(1.,0.,0.));
#13931=DIRECTION('center_axis',(0.,0.,1.));
#13932=DIRECTION('ref_axis',(1.,0.,0.));
#13933=DIRECTION('center_axis',(0.,0.,1.));
#13934=DIRECTION('ref_axis',(1.,0.,0.));
#13935=DIRECTION('center_axis',(0.,0.,1.));
#13936=DIRECTION('ref_axis',(1.,0.,0.));
#13937=DIRECTION('center_axis',(0.,0.,1.));
#13938=DIRECTION('ref_axis',(1.,0.,0.));
#13939=DIRECTION('center_axis',(0.,0.,1.));
#13940=DIRECTION('ref_axis',(1.,0.,0.));
#13941=DIRECTION('center_axis',(0.,0.,1.));
#13942=DIRECTION('ref_axis',(1.,0.,0.));
#13943=DIRECTION('center_axis',(0.,0.,1.));
#13944=DIRECTION('ref_axis',(1.,0.,0.));
#13945=DIRECTION('center_axis',(0.,0.,1.));
#13946=DIRECTION('ref_axis',(1.,0.,0.));
#13947=DIRECTION('center_axis',(-0.866025403784429,-0.500000000000017,0.));
#13948=DIRECTION('ref_axis',(0.500000000000017,-0.866025403784429,0.));
#13949=DIRECTION('',(0.,0.,-1.));
#13950=DIRECTION('center_axis',(-0.866025403784429,0.500000000000017,0.));
#13951=DIRECTION('ref_axis',(-0.500000000000017,-0.866025403784429,0.));
#13952=DIRECTION('center_axis',(-0.866025403784429,-0.500000000000017,0.));
#13953=DIRECTION('ref_axis',(0.500000000000017,-0.866025403784429,0.));
#13954=DIRECTION('',(0.,0.,-1.));
#13955=DIRECTION('center_axis',(-0.866025403784429,0.500000000000017,0.));
#13956=DIRECTION('ref_axis',(-0.500000000000017,-0.866025403784429,0.));
#13957=DIRECTION('center_axis',(0.,0.,-1.));
#13958=DIRECTION('ref_axis',(-1.,0.,0.));
#13959=DIRECTION('',(0.,1.,0.));
#13960=DIRECTION('',(-1.,0.,0.));
#13961=DIRECTION('',(0.,1.,0.));
#13962=DIRECTION('',(1.,0.,0.));
#13963=DIRECTION('',(0.,-1.,0.));
#13964=DIRECTION('center_axis',(-1.,0.,0.));
#13965=DIRECTION('ref_axis',(0.,0.,1.));
#13966=DIRECTION('center_axis',(1.,0.,0.));
#13967=DIRECTION('ref_axis',(0.,0.,-1.));
#13968=DIRECTION('',(0.,0.,1.));
#13969=DIRECTION('center_axis',(0.500000000000017,0.866025403784429,0.));
#13970=DIRECTION('ref_axis',(-0.866025403784429,0.500000000000017,0.));
#13971=DIRECTION('',(0.,0.,1.));
#13972=DIRECTION('',(-0.866025403784429,0.500000000000017,0.));
#13973=DIRECTION('center_axis',(-0.500000000000017,0.866025403784429,0.));
#13974=DIRECTION('ref_axis',(-0.866025403784429,-0.500000000000017,0.));
#13975=DIRECTION('',(-0.866025403784429,-0.500000000000017,0.));
#13976=DIRECTION('',(-0.866025403784429,-0.500000000000017,0.));
#13977=DIRECTION('center_axis',(0.500000000000017,0.866025403784429,0.));
#13978=DIRECTION('ref_axis',(-0.866025403784429,0.500000000000017,0.));
#13979=DIRECTION('',(-0.866025403784429,0.500000000000017,0.));
#13980=DIRECTION('',(-0.866025403784429,0.500000000000017,0.));
#13981=DIRECTION('center_axis',(0.,0.,1.));
#13982=DIRECTION('ref_axis',(1.,0.,0.));
#13983=DIRECTION('center_axis',(0.,0.,1.));
#13984=DIRECTION('ref_axis',(1.,0.,0.));
#13985=DIRECTION('center_axis',(0.,0.,-1.));
#13986=DIRECTION('ref_axis',(-1.,0.,0.));
#13987=DIRECTION('center_axis',(0.,0.,-1.));
#13988=DIRECTION('ref_axis',(-1.,0.,0.));
#13989=DIRECTION('center_axis',(0.,0.,-1.));
#13990=DIRECTION('ref_axis',(-1.,0.,0.));
#13991=DIRECTION('center_axis',(0.,0.,-1.));
#13992=DIRECTION('ref_axis',(-1.,0.,0.));
#13993=DIRECTION('center_axis',(0.,1.,0.));
#13994=DIRECTION('ref_axis',(0.,0.,1.));
#13995=DIRECTION('',(1.,0.,0.));
#13996=DIRECTION('',(0.,0.,-1.));
#13997=DIRECTION('',(0.,0.,1.));
#13998=DIRECTION('center_axis',(1.,0.,0.));
#13999=DIRECTION('ref_axis',(0.,0.,-1.));
#14000=DIRECTION('',(0.,-1.,0.));
#14001=DIRECTION('',(0.,0.,-1.));
#14002=DIRECTION('center_axis',(0.,-1.,0.));
#14003=DIRECTION('ref_axis',(0.,0.,-1.));
#14004=DIRECTION('',(-1.,0.,0.));
#14005=DIRECTION('',(0.,0.,-1.));
#14006=DIRECTION('center_axis',(-1.,0.,0.));
#14007=DIRECTION('ref_axis',(0.,0.,1.));
#14008=DIRECTION('',(0.,1.,0.));
#14009=DIRECTION('center_axis',(-1.,0.,0.));
#14010=DIRECTION('ref_axis',(0.,0.,1.));
#14011=DIRECTION('',(0.,1.,0.));
#14012=DIRECTION('',(0.,0.,-1.));
#14013=DIRECTION('',(0.,0.,1.));
#14014=DIRECTION('center_axis',(0.,1.,0.));
#14015=DIRECTION('ref_axis',(0.,0.,1.));
#14016=DIRECTION('',(1.,0.,0.));
#14017=DIRECTION('',(0.,0.,-1.));
#14018=DIRECTION('center_axis',(1.,0.,0.));
#14019=DIRECTION('ref_axis',(0.,0.,-1.));
#14020=DIRECTION('',(0.,-1.,0.));
#14021=DIRECTION('',(0.,0.,-1.));
#14022=DIRECTION('center_axis',(0.,-1.,0.));
#14023=DIRECTION('ref_axis',(0.,0.,-1.));
#14024=DIRECTION('',(-1.,0.,0.));
#14025=DIRECTION('center_axis',(0.,0.,-1.));
#14026=DIRECTION('ref_axis',(-1.,0.,0.));
#14027=DIRECTION('center_axis',(0.,0.,1.));
#14028=DIRECTION('ref_axis',(1.,0.,0.));
#14029=DIRECTION('center_axis',(0.,0.,-1.));
#14030=DIRECTION('ref_axis',(-1.,0.,0.));
#14031=DIRECTION('center_axis',(0.,0.,1.));
#14032=DIRECTION('ref_axis',(1.,0.,0.));
#14033=DIRECTION('center_axis',(0.,0.,-1.));
#14034=DIRECTION('ref_axis',(-1.,0.,0.));
#14035=DIRECTION('center_axis',(0.,0.,-1.));
#14036=DIRECTION('ref_axis',(-1.,0.,0.));
#14037=DIRECTION('center_axis',(0.,0.,-1.));
#14038=DIRECTION('ref_axis',(-1.,0.,0.));
#14039=DIRECTION('center_axis',(0.,0.,-1.));
#14040=DIRECTION('ref_axis',(-1.,0.,0.));
#15688=CARTESIAN_POINT('',(0.,0.,0.));
#15689=CARTESIAN_POINT('Origin',(0.,0.,-1.05));
#15690=CARTESIAN_POINT('',(-5.5,-6.73555739531044E-16,21.));
#15691=CARTESIAN_POINT('Origin',(0.,0.,21.));
#15692=CARTESIAN_POINT('',(-5.5,-6.73555739531044E-16,20.5));
#15693=CARTESIAN_POINT('',(-5.5,-6.73555739531044E-16,-1.05));
#15694=CARTESIAN_POINT('Origin',(0.,0.,20.5));
#15695=CARTESIAN_POINT('Origin',(0.,0.,28.375));
#15696=CARTESIAN_POINT('',(14.,-1.71450551880629E-15,21.));
#15697=CARTESIAN_POINT('Origin',(0.,0.,21.));
#15698=CARTESIAN_POINT('',(14.,-1.71450551880629E-15,23.5));
#15699=CARTESIAN_POINT('',(14.,-1.71450551880629E-15,28.375));
#15700=CARTESIAN_POINT('Origin',(0.,0.,23.5));
#15701=CARTESIAN_POINT('Origin',(11.,-45.3,0.));
#15702=CARTESIAN_POINT('',(12.35,-45.3,-14.5));
#15703=CARTESIAN_POINT('Origin',(11.,-45.3,-14.5));
#15704=CARTESIAN_POINT('',(12.35,-45.3,-17.));
#15705=CARTESIAN_POINT('',(12.35,-45.3,0.));
#15706=CARTESIAN_POINT('Origin',(11.,-45.3,-17.));
#15707=CARTESIAN_POINT('Origin',(17.3,-18.,0.));
#15708=CARTESIAN_POINT('',(18.65,-18.,-14.5));
#15709=CARTESIAN_POINT('Origin',(17.3,-18.,-14.5));
#15710=CARTESIAN_POINT('',(18.65,-18.,-17.));
#15711=CARTESIAN_POINT('',(18.65,-18.,0.));
#15712=CARTESIAN_POINT('Origin',(17.3,-18.,-17.));
#15713=CARTESIAN_POINT('Origin',(17.3,4.,0.));
#15714=CARTESIAN_POINT('',(18.65,4.,-14.5));
#15715=CARTESIAN_POINT('Origin',(17.3,4.,-14.5));
#15716=CARTESIAN_POINT('',(18.65,4.,-17.));
#15717=CARTESIAN_POINT('',(18.65,4.,0.));
#15718=CARTESIAN_POINT('Origin',(17.3,4.,-17.));
#15719=CARTESIAN_POINT('Origin',(-11.,-45.3,0.));
#15720=CARTESIAN_POINT('',(-9.65,-45.3,-14.5));
#15721=CARTESIAN_POINT('Origin',(-11.,-45.3,-14.5));
#15722=CARTESIAN_POINT('',(-9.65,-45.3,-17.));
#15723=CARTESIAN_POINT('',(-9.65,-45.3,0.));
#15724=CARTESIAN_POINT('Origin',(-11.,-45.3,-17.));
#15725=CARTESIAN_POINT('Origin',(-17.3,-18.,0.));
#15726=CARTESIAN_POINT('',(-15.95,-18.,-14.5));
#15727=CARTESIAN_POINT('Origin',(-17.3,-18.,-14.5));
#15728=CARTESIAN_POINT('',(-15.95,-18.,-17.));
#15729=CARTESIAN_POINT('',(-15.95,-18.,0.));
#15730=CARTESIAN_POINT('Origin',(-17.3,-18.,-17.));
#15731=CARTESIAN_POINT('Origin',(-17.3,4.,0.));
#15732=CARTESIAN_POINT('',(-15.95,4.,-14.5));
#15733=CARTESIAN_POINT('Origin',(-17.3,4.,-14.5));
#15734=CARTESIAN_POINT('',(-15.95,4.,-17.));
#15735=CARTESIAN_POINT('',(-15.95,4.,0.));
#15736=CARTESIAN_POINT('Origin',(-17.3,4.,-17.));
#15737=CARTESIAN_POINT('Origin',(11.,-45.3,0.));
#15738=CARTESIAN_POINT('',(12.35,-45.3,17.));
#15739=CARTESIAN_POINT('Origin',(11.,-45.3,17.));
#15740=CARTESIAN_POINT('',(12.35,-45.3,14.5));
#15741=CARTESIAN_POINT('',(12.35,-45.3,0.));
#15742=CARTESIAN_POINT('Origin',(11.,-45.3,14.5));
#15743=CARTESIAN_POINT('Origin',(17.3,-18.,0.));
#15744=CARTESIAN_POINT('',(18.65,-18.,17.));
#15745=CARTESIAN_POINT('Origin',(17.3,-18.,17.));
#15746=CARTESIAN_POINT('',(18.65,-18.,14.5));
#15747=CARTESIAN_POINT('',(18.65,-18.,0.));
#15748=CARTESIAN_POINT('Origin',(17.3,-18.,14.5));
#15749=CARTESIAN_POINT('Origin',(17.3,4.,0.));
#15750=CARTESIAN_POINT('',(18.65,4.,17.));
#15751=CARTESIAN_POINT('Origin',(17.3,4.,17.));
#15752=CARTESIAN_POINT('',(18.65,4.,14.5));
#15753=CARTESIAN_POINT('',(18.65,4.,0.));
#15754=CARTESIAN_POINT('Origin',(17.3,4.,14.5));
#15755=CARTESIAN_POINT('Origin',(-11.,-45.3,0.));
#15756=CARTESIAN_POINT('',(-9.65,-45.3,17.));
#15757=CARTESIAN_POINT('Origin',(-11.,-45.3,17.));
#15758=CARTESIAN_POINT('',(-9.65,-45.3,14.5));
#15759=CARTESIAN_POINT('',(-9.65,-45.3,0.));
#15760=CARTESIAN_POINT('Origin',(-11.,-45.3,14.5));
#15761=CARTESIAN_POINT('Origin',(-17.3,-18.,0.));
#15762=CARTESIAN_POINT('',(-15.95,-18.,17.));
#15763=CARTESIAN_POINT('Origin',(-17.3,-18.,17.));
#15764=CARTESIAN_POINT('',(-15.95,-18.,14.5));
#15765=CARTESIAN_POINT('',(-15.95,-18.,0.));
#15766=CARTESIAN_POINT('Origin',(-17.3,-18.,14.5));
#15767=CARTESIAN_POINT('Origin',(-17.3,4.,0.));
#15768=CARTESIAN_POINT('',(-15.95,4.,17.));
#15769=CARTESIAN_POINT('Origin',(-17.3,4.,17.));
#15770=CARTESIAN_POINT('',(-15.95,4.,14.5));
#15771=CARTESIAN_POINT('',(-15.95,4.,0.));
#15772=CARTESIAN_POINT('Origin',(-17.3,4.,14.5));
#15773=CARTESIAN_POINT('Origin',(0.,0.,28.375));
#15774=CARTESIAN_POINT('',(5.,-6.12323399573677E-16,23.5));
#15775=CARTESIAN_POINT('Origin',(0.,0.,23.5));
#15776=CARTESIAN_POINT('',(5.,-6.12323399573677E-16,25.));
#15777=CARTESIAN_POINT('',(5.,-6.12323399573677E-16,28.375));
#15778=CARTESIAN_POINT('Origin',(0.,0.,25.));
#15779=CARTESIAN_POINT('Origin',(0.,0.,-23.1));
#15780=CARTESIAN_POINT('',(-7.5,-9.18485099360515E-16,-20.5));
#15781=CARTESIAN_POINT('Origin',(0.,0.,-20.5));
#15782=CARTESIAN_POINT('',(-7.5,-9.18485099360515E-16,-19.5));
#15783=CARTESIAN_POINT('',(-7.5,-9.18485099360515E-16,-23.1));
#15784=CARTESIAN_POINT('Origin',(0.,0.,-19.5));
#15785=CARTESIAN_POINT('Origin',(0.,0.,28.375));
#15786=CARTESIAN_POINT('',(2.75,-3.36777869765522E-16,25.));
#15787=CARTESIAN_POINT('Origin',(0.,0.,25.));
#15788=CARTESIAN_POINT('',(2.75,-3.36777869765522E-16,28.));
#15789=CARTESIAN_POINT('',(2.75,-3.36777869765522E-16,28.375));
#15790=CARTESIAN_POINT('Origin',(0.,0.,28.));
#15791=CARTESIAN_POINT('Origin',(0.,0.,-23.1));
#15792=CARTESIAN_POINT('',(-5.,-6.12323399573677E-16,-19.5));
#15793=CARTESIAN_POINT('Origin',(0.,0.,-19.5));
#15794=CARTESIAN_POINT('',(-5.,-6.12323399573677E-16,-19.8));
#15795=CARTESIAN_POINT('',(-5.,-6.12323399573677E-16,-23.1));
#15796=CARTESIAN_POINT('Origin',(0.,0.,-19.8));
#15797=CARTESIAN_POINT('Origin',(0.,0.,1.305));
#15798=CARTESIAN_POINT('',(7.25,-8.87868929381831E-16,-21.));
#15799=CARTESIAN_POINT('Origin',(0.,0.,-21.));
#15800=CARTESIAN_POINT('',(7.25,-8.87868929381831E-16,-19.8));
#15801=CARTESIAN_POINT('',(7.25,-8.87868929381831E-16,1.305));
#15802=CARTESIAN_POINT('Origin',(0.,0.,-19.8));
#15803=CARTESIAN_POINT('Origin',(0.,0.,1.305));
#15804=CARTESIAN_POINT('',(14.,-1.71450551880629E-15,-23.5));
#15805=CARTESIAN_POINT('Origin',(0.,0.,-23.5));
#15806=CARTESIAN_POINT('',(14.,-1.71450551880629E-15,-21.));
#15807=CARTESIAN_POINT('',(14.,-1.71450551880629E-15,1.305));
#15808=CARTESIAN_POINT('Origin',(0.,0.,-21.));
#15809=CARTESIAN_POINT('Origin',(0.,0.,1.305));
#15810=CARTESIAN_POINT('',(4.75,-5.81707229594993E-16,-24.3));
#15811=CARTESIAN_POINT('Origin',(0.,0.,-24.3));
#15812=CARTESIAN_POINT('',(4.75,-5.81707229594993E-16,-23.5));
#15813=CARTESIAN_POINT('',(4.75,-5.81707229594993E-16,1.305));
#15814=CARTESIAN_POINT('Origin',(0.,0.,-23.5));
#15815=CARTESIAN_POINT('Origin',(0.,0.,1.305));
#15816=CARTESIAN_POINT('',(2.75,-3.36777869765522E-16,-26.1));
#15817=CARTESIAN_POINT('Origin',(0.,0.,-26.1));
#15818=CARTESIAN_POINT('',(2.75,-3.36777869765522E-16,-24.3));
#15819=CARTESIAN_POINT('',(2.75,-3.36777869765522E-16,1.305));
#15820=CARTESIAN_POINT('Origin',(0.,0.,-24.3));
#15821=CARTESIAN_POINT('Origin',(0.,0.,20.5));
#15822=CARTESIAN_POINT('',(13.,-41.,20.5));
#15823=CARTESIAN_POINT('',(13.0000000000055,11.,20.4999999999987));
#15824=CARTESIAN_POINT('',(13.,0.,20.5));
#15825=CARTESIAN_POINT('',(-13.,10.9999999999864,20.4999999999983));
#15826=CARTESIAN_POINT('',(0.,11.,20.5));
#15827=CARTESIAN_POINT('',(-13.,-41.,20.5));
#15828=CARTESIAN_POINT('',(-13.,0.,20.5));
#15829=CARTESIAN_POINT('',(0.,-41.,20.5));
#15830=CARTESIAN_POINT('Origin',(14.63200966641,11.,18.5));
#15831=CARTESIAN_POINT('',(13.,12.9999999999984,18.4999999991966));
#15832=CARTESIAN_POINT('Origin',(13.,11.,18.5));
#15833=CARTESIAN_POINT('',(-12.9999999999935,13.0000000000008,18.49999999892));
#15834=CARTESIAN_POINT('',(14.63200966641,13.,18.49999999892));
#15835=CARTESIAN_POINT('Origin',(-13.,11.,18.5));
#15836=CARTESIAN_POINT('Origin',(13.,-42.63464535978,19.));
#15837=CARTESIAN_POINT('',(14.5000000000004,-41.,18.9999999999984));
#15838=CARTESIAN_POINT('',(14.5000000000014,11.0000000000001,18.999999864659));
#15839=CARTESIAN_POINT('',(14.5,-42.63464535978,19.));
#15840=CARTESIAN_POINT('Origin',(13.,11.,19.));
#15841=CARTESIAN_POINT('Origin',(13.,-41.,19.));
#15842=CARTESIAN_POINT('Origin',(-14.67485779376,-41.,19.));
#15843=CARTESIAN_POINT('',(-13.,-42.5000000000004,18.9999999999985));
#15844=CARTESIAN_POINT('',(13.,-42.5000000000002,19.));
#15845=CARTESIAN_POINT('',(-14.67485779376,-42.5,19.));
#15846=CARTESIAN_POINT('Origin',(13.,-41.,19.));
#15847=CARTESIAN_POINT('Origin',(-13.,-41.,19.));
#15848=CARTESIAN_POINT('Origin',(-13.,11.13971317669,19.));
#15849=CARTESIAN_POINT('',(-14.5000000000014,11.000000000002,18.9999998643683));
#15850=CARTESIAN_POINT('Origin',(-13.,11.,19.));
#15851=CARTESIAN_POINT('',(-14.5000000000002,-41.0000000021332,18.9999998796623));
#15852=CARTESIAN_POINT('',(-14.5,11.13971317669,18.99999972876));
#15853=CARTESIAN_POINT('Origin',(-13.,-41.,19.));
#15854=CARTESIAN_POINT('Origin',(0.,0.,21.));
#15855=CARTESIAN_POINT('Origin',(14.5,13.,-20.5));
#15856=CARTESIAN_POINT('',(13.,13.,17.));
#15857=CARTESIAN_POINT('',(13.,13.,18.63971317669));
#15858=CARTESIAN_POINT('',(13.94140536675,13.,17.));
#15859=CARTESIAN_POINT('',(0.,13.,17.));
#15860=CARTESIAN_POINT('',(13.94140536675,13.,14.5));
#15861=CARTESIAN_POINT('',(13.94140536675,13.,-20.5));
#15862=CARTESIAN_POINT('',(12.5,13.,14.5));
#15863=CARTESIAN_POINT('',(0.,13.,14.5));
#15864=CARTESIAN_POINT('',(12.5,13.,-14.5));
#15865=CARTESIAN_POINT('',(12.5,13.,-20.5));
#15866=CARTESIAN_POINT('',(13.94140536675,13.,-14.5));
#15867=CARTESIAN_POINT('',(0.,13.,-14.5));
#15868=CARTESIAN_POINT('',(13.94140536675,13.,-17.));
#15869=CARTESIAN_POINT('',(13.94140536675,13.,-20.5));
#15870=CARTESIAN_POINT('',(6.65,13.,-17.));
#15871=CARTESIAN_POINT('',(14.5,13.,-17.));
#15872=CARTESIAN_POINT('',(-6.65,13.,-17.));
#15873=CARTESIAN_POINT('',(14.5,13.,-17.));
#15874=CARTESIAN_POINT('',(-13.94140536675,13.,-17.));
#15875=CARTESIAN_POINT('',(14.5,13.,-17.));
#15876=CARTESIAN_POINT('',(-13.94140536675,13.,-14.5));
#15877=CARTESIAN_POINT('',(-13.94140536675,13.,-20.5));
#15878=CARTESIAN_POINT('',(-12.5,13.,-14.5));
#15879=CARTESIAN_POINT('',(0.,13.,-14.5));
#15880=CARTESIAN_POINT('',(-12.5,13.,14.5));
#15881=CARTESIAN_POINT('',(-12.5,13.,-20.5));
#15882=CARTESIAN_POINT('',(-13.94140536675,13.,14.5));
#15883=CARTESIAN_POINT('',(0.,13.,14.5));
#15884=CARTESIAN_POINT('',(-13.94140536675,13.,17.));
#15885=CARTESIAN_POINT('',(-13.94140536675,13.,-20.5));
#15886=CARTESIAN_POINT('',(-13.,13.,17.));
#15887=CARTESIAN_POINT('',(0.,13.,17.));
#15888=CARTESIAN_POINT('',(-13.,13.,-17.13464535978));
#15889=CARTESIAN_POINT('Ctrl Pts',(14.5000000000041,11.0000000000019,18.99999972876));
#15890=CARTESIAN_POINT('Ctrl Pts',(14.5000000000077,11.499999728971,18.9999997287616));
#15891=CARTESIAN_POINT('Ctrl Pts',(14.5000000000013,11.4999997287644,18.4999999997925));
#15892=CARTESIAN_POINT('Ctrl Pts',(14.5000001123536,11.0000000000019,19.6213201517653));
#15893=CARTESIAN_POINT('Ctrl Pts',(14.5000001123618,12.1213201522332,19.621320151769));
#15894=CARTESIAN_POINT('Ctrl Pts',(14.5000001123474,12.1213201517697,18.4999999995377));
#15895=CARTESIAN_POINT('Ctrl Pts',(14.0606602676774,11.0000000000052,20.0606600758827));
#15896=CARTESIAN_POINT('Ctrl Pts',(14.0606602676888,12.5606600765297,20.0606600758878));
#15897=CARTESIAN_POINT('Ctrl Pts',(14.0606602676688,12.5606600758847,18.4999999993632));
#15898=CARTESIAN_POINT('Ctrl Pts',(13.6213204230012,11.0000000000084,20.5000000000001));
#15899=CARTESIAN_POINT('Ctrl Pts',(13.6213204230159,13.0000000008263,20.5000000000066));
#15900=CARTESIAN_POINT('Ctrl Pts',(13.6213204229902,12.9999999999996,18.4999999991887));
#15901=CARTESIAN_POINT('Ctrl Pts',(12.9999999999959,11.0000000000129,20.4999999999974));
#15902=CARTESIAN_POINT('Ctrl Pts',(13.0000000000105,13.0000000008201,20.5000000000039));
#15903=CARTESIAN_POINT('Ctrl Pts',(12.9999999999848,12.9999999999935,18.4999999991966));
#15904=CARTESIAN_POINT('',(14.5000000000009,11.4999998646612,18.4999999999998));
#15905=CARTESIAN_POINT('Origin',(14.4999999999976,11.0000000000019,18.4999999999976));
#15906=CARTESIAN_POINT('Origin',(12.9999999999996,11.4999999999918,18.5000000000193));
#15907=CARTESIAN_POINT('Ctrl Pts',(-13.,10.9999999999728,20.4999999999966));
#15908=CARTESIAN_POINT('Ctrl Pts',(-12.9999999999873,13.000000001073,20.5000000000202));
#15909=CARTESIAN_POINT('Ctrl Pts',(-12.9999999999738,13.000000000003,18.49999999892));
#15910=CARTESIAN_POINT('Ctrl Pts',(-13.6213203832862,10.9999999999767,20.5));
#15911=CARTESIAN_POINT('Ctrl Pts',(-13.6213203832735,13.0000000010845,20.5000000000236));
#15912=CARTESIAN_POINT('Ctrl Pts',(-13.6213203832599,13.0000000000145,18.4999999989158));
#15913=CARTESIAN_POINT('Ctrl Pts',(-14.0606602197355,10.9999999999847,20.0606601238272));
#15914=CARTESIAN_POINT('Ctrl Pts',(-14.0606602197256,12.5606601246825,20.0606601238456));
#15915=CARTESIAN_POINT('Ctrl Pts',(-14.0606602197151,12.5606601238475,18.4999999991479));
#15916=CARTESIAN_POINT('Ctrl Pts',(-14.5000000561849,10.9999999999927,19.6213202476545));
#15917=CARTESIAN_POINT('Ctrl Pts',(-14.5000000561778,12.1213202482804,19.6213202476677));
#15918=CARTESIAN_POINT('Ctrl Pts',(-14.5000000561702,12.1213202476805,18.4999999993799));
#15919=CARTESIAN_POINT('Ctrl Pts',(-14.5000000000041,11.,18.9999998643683));
#15920=CARTESIAN_POINT('Ctrl Pts',(-14.500000000001,11.4999998646618,18.9999998643742));
#15921=CARTESIAN_POINT('Ctrl Pts',(-14.4999999999976,11.4999998643943,18.4999999997124));
#15922=CARTESIAN_POINT('',(-14.4999999999976,11.5000000000041,18.4999999998461));
#15923=CARTESIAN_POINT('Origin',(-14.5000000000007,11.0000000000059,18.4999999999799));
#15924=CARTESIAN_POINT('Origin',(-13.0000000000016,11.500000000007,18.4999999997225));
#15925=CARTESIAN_POINT('Origin',(14.5,-42.5,-20.5));
#15926=CARTESIAN_POINT('',(14.5000000000008,-41.5,18.4999999994855));
#15927=CARTESIAN_POINT('',(14.5,-41.5,17.));
#15928=CARTESIAN_POINT('',(14.5,-41.5,-20.5));
#15929=CARTESIAN_POINT('',(14.5,11.5,17.));
#15930=CARTESIAN_POINT('',(14.5,-42.5,17.));
#15931=CARTESIAN_POINT('',(14.5,11.5,-20.5));
#15932=CARTESIAN_POINT('Ctrl Pts',(14.5000000000019,-41.5,18.4999999994855));
#15933=CARTESIAN_POINT('Ctrl Pts',(14.5000000000027,-41.5000000003692,18.7411872045814));
#15934=CARTESIAN_POINT('Ctrl Pts',(14.5000000000008,-41.241175036448,18.9975772517615));
#15935=CARTESIAN_POINT('Ctrl Pts',(14.5000000000013,-41.,18.9999999999984));
#15936=CARTESIAN_POINT('Origin',(13.,-41.,19.));
#15937=CARTESIAN_POINT('Ctrl Pts',(13.,-42.5,19.));
#15938=CARTESIAN_POINT('Ctrl Pts',(13.0022600019965,-42.5,19.0595135681432));
#15939=CARTESIAN_POINT('Ctrl Pts',(13.0073620228215,-42.4964573811086,19.1183481172834));
#15940=CARTESIAN_POINT('Ctrl Pts',(13.0153053530606,-42.4895493826963,19.1760919722096));
#15941=CARTESIAN_POINT('Ctrl Pts',(13.0166707573604,-42.4883619448773,19.186017747096));
#15942=CARTESIAN_POINT('Ctrl Pts',(13.0181201082026,-42.4870749459193,19.1959113155762));
#15943=CARTESIAN_POINT('Ctrl Pts',(13.0196533909879,-42.4856891362025,19.2057705877734));
#15944=CARTESIAN_POINT('Ctrl Pts',(13.0232674597544,-42.4824226731195,19.2290096719467));
#15945=CARTESIAN_POINT('Ctrl Pts',(13.0272781780523,-42.4786470144108,19.2518093521003));
#15946=CARTESIAN_POINT('Ctrl Pts',(13.0317575007208,-42.4743454279988,19.2744030249233));
#15947=CARTESIAN_POINT('Ctrl Pts',(13.0362018078404,-42.4700774677444,19.2968200795573));
#15948=CARTESIAN_POINT('Ctrl Pts',(13.0411074346211,-42.4652916250984,19.319034767169));
#15949=CARTESIAN_POINT('Ctrl Pts',(13.0465443279543,-42.4599219905355,19.3412644239973));
#15950=CARTESIAN_POINT('Ctrl Pts',(13.0514771601157,-42.4550501814998,19.3614331415751));
#15951=CARTESIAN_POINT('Ctrl Pts',(13.0568473243571,-42.4496972429146,19.381614336539));
#15952=CARTESIAN_POINT('Ctrl Pts',(13.0627066489669,-42.4437789851613,19.4019578562263));
#15953=CARTESIAN_POINT('Ctrl Pts',(13.0781595750634,-42.4281706333847,19.4556102696368));
#15954=CARTESIAN_POINT('Ctrl Pts',(13.096287694905,-42.4096294661813,19.5068516934207));
#15955=CARTESIAN_POINT('Ctrl Pts',(13.1170615404762,-42.3885021085325,19.5553003604737));
#15956=CARTESIAN_POINT('Ctrl Pts',(13.121596504369,-42.3838899723846,19.5658767823976));
#15957=CARTESIAN_POINT('Ctrl Pts',(13.1262574478728,-42.3791544387863,19.576320041403));
#15958=CARTESIAN_POINT('Ctrl Pts',(13.1310438701017,-42.3742988849167,19.5866260129124));
#15959=CARTESIAN_POINT('Ctrl Pts',(13.1443999464751,-42.3607499029811,19.61538389009));
#15960=CARTESIAN_POINT('Ctrl Pts',(13.1587334900202,-42.3462665987258,19.6430731920815));
#15961=CARTESIAN_POINT('Ctrl Pts',(13.1740297517328,-42.3309201189407,19.6696008381944));
#15962=CARTESIAN_POINT('Ctrl Pts',(13.1816778825891,-42.3232468790482,19.6828646612509));
#15963=CARTESIAN_POINT('Ctrl Pts',(13.1895666820893,-42.3153577656199,19.6958380292812));
#15964=CARTESIAN_POINT('Ctrl Pts',(13.1976935757618,-42.3072615166738,19.7085086994005));
#15965=CARTESIAN_POINT('Ctrl Pts',(13.201757022598,-42.3032133922008,19.7148440344601));
#15966=CARTESIAN_POINT('Ctrl Pts',(13.2058799925008,-42.2991134795606,19.7211036930466));
#15967=CARTESIAN_POINT('Ctrl Pts',(13.2100621289868,-42.2949628612153,19.7272861129147));
#15968=CARTESIAN_POINT('Ctrl Pts',(13.2129317585393,-42.2921148582616,19.7315282639825));
#15969=CARTESIAN_POINT('Ctrl Pts',(13.2161072666261,-42.2889722558305,19.7361264257699));
#15970=CARTESIAN_POINT('Ctrl Pts',(13.2190161563155,-42.2860911505925,19.7402712176225));
#15971=CARTESIAN_POINT('Ctrl Pts',(13.2203466199925,-42.284773394927,19.7421669564086));
#15972=CARTESIAN_POINT('Ctrl Pts',(13.2216213369746,-42.2835109849067,19.7439683311336));
#15973=CARTESIAN_POINT('Ctrl Pts',(13.2227856645689,-42.2823599620334,19.7456000774117));
#15974=CARTESIAN_POINT('Ctrl Pts',(13.2405637499002,-42.2647850261129,19.7705151654961));
#15975=CARTESIAN_POINT('Ctrl Pts',(13.2598640476569,-42.2459665645706,19.794609810812));
#15976=CARTESIAN_POINT('Ctrl Pts',(13.280640545793,-42.2258491150598,19.817639793041));
#15977=CARTESIAN_POINT('Ctrl Pts',(13.3008006762611,-42.2063284814975,19.8399865544333));
#15978=CARTESIAN_POINT('Ctrl Pts',(13.3223509770152,-42.1855841698294,19.8613306716809));
#15979=CARTESIAN_POINT('Ctrl Pts',(13.3452294106433,-42.1635863623897,19.8814099110445));
#15980=CARTESIAN_POINT('Ctrl Pts',(13.3680574656428,-42.1416369944276,19.9014449356443));
#15981=CARTESIAN_POINT('Ctrl Pts',(13.3922081789123,-42.118438919148,19.920220446142));
#15982=CARTESIAN_POINT('Ctrl Pts',(13.4175949294985,-42.0939937051849,19.9374391968938));
#15983=CARTESIAN_POINT('Ctrl Pts',(13.4413843219079,-42.0710866070304,19.9535745276856));
#15984=CARTESIAN_POINT('Ctrl Pts',(13.4662591457969,-42.0470841490337,19.9683422449708));
#15985=CARTESIAN_POINT('Ctrl Pts',(13.4921236617146,-42.0220212156595,19.9814718214613));
#15986=CARTESIAN_POINT('Ctrl Pts',(13.5174413758943,-41.9974881377666,19.9943238255717));
#15987=CARTESIAN_POINT('Ctrl Pts',(13.5437075604478,-41.9719385906071,20.0056057520624));
#15988=CARTESIAN_POINT('Ctrl Pts',(13.570806305913,-41.9454430912019,20.0150455765278));
#15989=CARTESIAN_POINT('Ctrl Pts',(13.5971431853015,-41.9196924979476,20.0242200056066));
#15990=CARTESIAN_POINT('Ctrl Pts',(13.6242665788035,-41.8930481880007,20.0316539195686));
#15991=CARTESIAN_POINT('Ctrl Pts',(13.6520430849402,-41.8656150102203,20.0370874936393));
#15992=CARTESIAN_POINT('Ctrl Pts',(13.6599625404344,-41.8577934422582,20.0386366786886));
#15993=CARTESIAN_POINT('Ctrl Pts',(13.6679349096588,-41.8499080132866,20.0400232205286));
#15994=CARTESIAN_POINT('Ctrl Pts',(13.6759566644666,-41.8419618070235,20.0412410399504));
#15995=CARTESIAN_POINT('Ctrl Pts',(13.6895615020067,-41.8284850992632,20.0433064527912));
#15996=CARTESIAN_POINT('Ctrl Pts',(13.7033084869149,-41.8148334295775,20.0448865414525));
#15997=CARTESIAN_POINT('Ctrl Pts',(13.717179038175,-41.8010238866563,20.0459517007053));
#15998=CARTESIAN_POINT('Ctrl Pts',(13.724114313805,-41.7941191151957,20.0464842803318));
#15999=CARTESIAN_POINT('Ctrl Pts',(13.7310804857782,-41.7871748806342,20.0468881344742));
#16000=CARTESIAN_POINT('Ctrl Pts',(13.7380750284017,-41.7801936070758,20.0471595809273));
#16001=CARTESIAN_POINT('Ctrl Pts',(13.7415722997135,-41.7767029702966,20.0472953041538));
#16002=CARTESIAN_POINT('Ctrl Pts',(13.7450766640847,-41.7732030742176,20.0473979260408));
#16003=CARTESIAN_POINT('Ctrl Pts',(13.7485878000073,-41.7696942321775,20.0474669897581));
#16004=CARTESIAN_POINT('Ctrl Pts',(13.7512425761001,-41.7670411904934,20.0475192089571));
#16005=CARTESIAN_POINT('Ctrl Pts',(13.7543988140343,-41.7638864585117,20.0475555844872));
#16006=CARTESIAN_POINT('Ctrl Pts',(13.7569273746179,-41.7613564491054,20.0475673281273));
#16007=CARTESIAN_POINT('Ctrl Pts',(13.7577430206971,-41.7605403356747,20.0475711163117));
#16008=CARTESIAN_POINT('Ctrl Pts',(13.7584934884386,-41.7597892758663,20.0475727773388));
#16009=CARTESIAN_POINT('Ctrl Pts',(13.7591411982523,-41.759141187524,20.0475730516392));
#16010=CARTESIAN_POINT('Ctrl Pts',(13.7804931212882,-41.737776786194,20.0475820940233));
#16011=CARTESIAN_POINT('Ctrl Pts',(13.8026529827082,-41.7156086502557,20.0462820505169));
#16012=CARTESIAN_POINT('Ctrl Pts',(13.8254839294119,-41.6927124027106,20.0434202458328));
#16013=CARTESIAN_POINT('Ctrl Pts',(13.8481437807808,-41.6699877398652,20.0405798875405));
#16014=CARTESIAN_POINT('Ctrl Pts',(13.8714648760683,-41.6465453989694,20.0362005538643));
#16015=CARTESIAN_POINT('Ctrl Pts',(13.8952849873058,-41.6225025400937,20.0300268826986));
#16016=CARTESIAN_POINT('Ctrl Pts',(13.9191050985433,-41.5984596812179,20.0238532115329));
#16017=CARTESIAN_POINT('Ctrl Pts',(13.9434244185068,-41.5738158694174,20.0158845175339));
#16018=CARTESIAN_POINT('Ctrl Pts',(13.9680493372696,-41.5487382983821,20.0058661742501));
#16019=CARTESIAN_POINT('Ctrl Pts',(13.9774576724811,-41.5391570202929,20.0020385095668));
#16020=CARTESIAN_POINT('Ctrl Pts',(13.9871299310897,-41.5292932146631,19.9978150358827));
#16021=CARTESIAN_POINT('Ctrl Pts',(13.9967972146374,-41.5194120987705,19.9932806172185));
#16022=CARTESIAN_POINT('Ctrl Pts',(14.0064058022661,-41.5095909771022,19.9887737297496));
#16023=CARTESIAN_POINT('Ctrl Pts',(14.0160093076807,-41.4997530911245,19.9839596557493));
#16024=CARTESIAN_POINT('Ctrl Pts',(14.0253653096026,-41.4901498663702,19.9789683806747));
#16025=CARTESIAN_POINT('Ctrl Pts',(14.0312956956529,-41.4840627759018,19.9758046160323));
#16026=CARTESIAN_POINT('Ctrl Pts',(14.0371270970891,-41.4780697607539,19.9725706227384));
#16027=CARTESIAN_POINT('Ctrl Pts',(14.0428025582095,-41.4722321415579,19.9693088409126));
#16028=CARTESIAN_POINT('Ctrl Pts',(14.0701611976478,-41.444091816856,19.9535853761571));
#16029=CARTESIAN_POINT('Ctrl Pts',(14.0963327095341,-41.4170311408489,19.9358471136713));
#16030=CARTESIAN_POINT('Ctrl Pts',(14.1212830788706,-41.3911979198333,19.9163451557992));
#16031=CARTESIAN_POINT('Ctrl Pts',(14.1394468349858,-41.3723914516857,19.9021478186062));
#16032=CARTESIAN_POINT('Ctrl Pts',(14.1569636554055,-41.3542343823022,19.8870160430856));
#16033=CARTESIAN_POINT('Ctrl Pts',(14.1738240978003,-41.3367668935452,19.871048245986));
#16034=CARTESIAN_POINT('Ctrl Pts',(14.1938343650591,-41.3160361730703,19.8520973857407));
#16035=CARTESIAN_POINT('Ctrl Pts',(14.2129199741926,-41.2962772848737,19.831969157362));
#16036=CARTESIAN_POINT('Ctrl Pts',(14.2310705495173,-41.277533093463,19.8108271604627));
#16037=CARTESIAN_POINT('Ctrl Pts',(14.2401458371797,-41.2681609977577,19.800256162013));
#16038=CARTESIAN_POINT('Ctrl Pts',(14.2489874564841,-41.2590421748574,19.7894316869671));
#16039=CARTESIAN_POINT('Ctrl Pts',(14.2575946377126,-41.2501796687351,19.778373856542));
#16040=CARTESIAN_POINT('Ctrl Pts',(14.2618982283269,-41.2457484156739,19.7728449413295));
#16041=CARTESIAN_POINT('Ctrl Pts',(14.2663517713443,-41.241168563312,19.7669825101897));
#16042=CARTESIAN_POINT('Ctrl Pts',(14.2706384453587,-41.2367626882401,19.7611973270011));
#16043=CARTESIAN_POINT('Ctrl Pts',(14.2749251193732,-41.2323568131681,19.7554121438125));
#16044=CARTESIAN_POINT('Ctrl Pts',(14.2790451446467,-41.2281247953352,19.7497046604192));
#16045=CARTESIAN_POINT('Ctrl Pts',(14.2827124379415,-41.224362680723,19.7445201065444));
#16046=CARTESIAN_POINT('Ctrl Pts',(14.2975068311355,-41.2091857645782,19.72360486405));
#16047=CARTESIAN_POINT('Ctrl Pts',(14.3123312731019,-41.1941459053188,19.7008120823962));
#16048=CARTESIAN_POINT('Ctrl Pts',(14.3269411120902,-41.1794304559121,19.6760414162875));
#16049=CARTESIAN_POINT('Ctrl Pts',(14.3413036351894,-41.1649641101715,19.6516900689212));
#16050=CARTESIAN_POINT('Ctrl Pts',(14.3554586875558,-41.1508114166492,19.6254266233223));
#16051=CARTESIAN_POINT('Ctrl Pts',(14.3691431631322,-41.1371752343504,19.5971850248702));
#16052=CARTESIAN_POINT('Ctrl Pts',(14.3779641249747,-41.1283854021742,19.5789805959956));
#16053=CARTESIAN_POINT('Ctrl Pts',(14.3865034944592,-41.1198922786354,19.5601396066395));
#16054=CARTESIAN_POINT('Ctrl Pts',(14.3947786423472,-41.1116665454347,19.5404841547009));
#16055=CARTESIAN_POINT('Ctrl Pts',(14.4028733946198,-41.1036201306248,19.5212571854187));
#16056=CARTESIAN_POINT('Ctrl Pts',(14.410715528531,-41.0958293476444,19.5012505187318));
#16057=CARTESIAN_POINT('Ctrl Pts',(14.4182846891418,-41.0882967432289,19.4802834847057));
#16058=CARTESIAN_POINT('Ctrl Pts',(14.4255810842607,-41.0810355869507,19.4600720276376));
#16059=CARTESIAN_POINT('Ctrl Pts',(14.4326239707515,-41.0740141774503,19.4389677887742));
#16060=CARTESIAN_POINT('Ctrl Pts',(14.4393582777847,-41.0672656586373,19.4168010068855));
#16061=CARTESIAN_POINT('Ctrl Pts',(14.4408457695643,-41.0657750277217,19.411904748714));
#16062=CARTESIAN_POINT('Ctrl Pts',(14.4423180536051,-41.0642978397888,19.4069566312962));
#16063=CARTESIAN_POINT('Ctrl Pts',(14.4437742694652,-41.0628346783189,19.4019548009798));
#16064=CARTESIAN_POINT('Ctrl Pts',(14.4516573514502,-41.0549139969553,19.3748778822768));
#16065=CARTESIAN_POINT('Ctrl Pts',(14.4582965000516,-41.0480624381763,19.3489100621108));
#16066=CARTESIAN_POINT('Ctrl Pts',(14.4639363713605,-41.042118421645,19.324216500453));
#16067=CARTESIAN_POINT('Ctrl Pts',(14.4661232995477,-41.039813557476,19.314641273808));
#16068=CARTESIAN_POINT('Ctrl Pts',(14.4681597602495,-41.0376451182981,19.3052571196166));
#16069=CARTESIAN_POINT('Ctrl Pts',(14.4700591414188,-41.0356036616017,19.2960717818563));
#16070=CARTESIAN_POINT('Ctrl Pts',(14.4734579900107,-41.0319505758862,19.2796350745664));
#16071=CARTESIAN_POINT('Ctrl Pts',(14.476418228949,-41.0287040152659,19.2638355064284));
#16072=CARTESIAN_POINT('Ctrl Pts',(14.4790122221541,-41.0258106568904,19.2487099851427));
#16073=CARTESIAN_POINT('Ctrl Pts',(14.4803092187566,-41.0243639777027,19.2411472244999));
#16074=CARTESIAN_POINT('Ctrl Pts',(14.481514544451,-41.0230055973116,19.2337529579336));
#16075=CARTESIAN_POINT('Ctrl Pts',(14.4826367188961,-41.0217290413751,19.2265308114627));
#16076=CARTESIAN_POINT('Ctrl Pts',(14.4833342254105,-41.0209355764324,19.2220417641192));
#16077=CARTESIAN_POINT('Ctrl Pts',(14.4839235680074,-41.0202614215225,19.2181274901393));
#16078=CARTESIAN_POINT('Ctrl Pts',(14.4845504272508,-41.0195394890262,19.2138416173666));
#16079=CARTESIAN_POINT('Ctrl Pts',(14.484932082493,-41.0190999496486,19.2112322184811));
#16080=CARTESIAN_POINT('Ctrl Pts',(14.4853270789767,-41.0186432748577,19.2084849018578));
#16081=CARTESIAN_POINT('Ctrl Pts',(14.4857618520254,-41.0181384289453,19.2053843140591));
#16082=CARTESIAN_POINT('Ctrl Pts',(14.4877126267577,-41.0158732456439,19.1914723469945));
#16083=CARTESIAN_POINT('Ctrl Pts',(14.489515707467,-41.0137373207059,19.1771172760478));
#16084=CARTESIAN_POINT('Ctrl Pts',(14.4911115466222,-41.0118111922518,19.1626248789929));
#16085=CARTESIAN_POINT('Ctrl Pts',(14.4926914198304,-41.0099043342014,19.1482774745222));
#16086=CARTESIAN_POINT('Ctrl Pts',(14.4940681434128,-41.0082032646087,19.1337957756093));
#16087=CARTESIAN_POINT('Ctrl Pts',(14.4952182617322,-41.0067485658386,19.1194855917744));
#16088=CARTESIAN_POINT('Ctrl Pts',(14.4956431563988,-41.0062111483064,19.1141989002344));
#16089=CARTESIAN_POINT('Ctrl Pts',(14.496037463468,-41.0057069741921,19.1089356844527));
#16090=CARTESIAN_POINT('Ctrl Pts',(14.4964011799049,-41.0052367471062,19.1037115483395));
#16091=CARTESIAN_POINT('Ctrl Pts',(14.4971421260223,-41.004278822475,19.0930691825373));
#16092=CARTESIAN_POINT('Ctrl Pts',(14.4977897638712,-41.0034179669619,19.082068267));
#16093=CARTESIAN_POINT('Ctrl Pts',(14.4983114829805,-41.0026999974748,19.0711014063315));
#16094=CARTESIAN_POINT('Ctrl Pts',(14.4986145428171,-41.0022829383494,19.0647308997844));
#16095=CARTESIAN_POINT('Ctrl Pts',(14.4988757478153,-41.0019133711413,19.0583720003773));
#16096=CARTESIAN_POINT('Ctrl Pts',(14.4990939964136,-41.0015941473328,19.052102289881));
#16097=CARTESIAN_POINT('Ctrl Pts',(14.4993692046759,-41.0011916108204,19.0441962774544));
#16098=CARTESIAN_POINT('Ctrl Pts',(14.4995892916705,-41.0008491769556,19.0359872297785));
#16099=CARTESIAN_POINT('Ctrl Pts',(14.4997384818162,-41.0005921979,19.0280024188491));
#16100=CARTESIAN_POINT('Ctrl Pts',(14.4997502855326,-41.0005718660751,19.0273706717324));
#16101=CARTESIAN_POINT('Ctrl Pts',(14.4997616629826,-41.0005520485121,19.0267403293932));
#16102=CARTESIAN_POINT('Ctrl Pts',(14.4997726153436,-41.0005327471464,19.0261116534472));
#16103=CARTESIAN_POINT('Ctrl Pts',(14.4998099608464,-41.000466933099,19.0239679860534));
#16104=CARTESIAN_POINT('Ctrl Pts',(14.4998429629253,-41.0004060665387,19.0218093930498));
#16105=CARTESIAN_POINT('Ctrl Pts',(14.4998714306183,-41.0003504001876,19.0196359067679));
#16106=CARTESIAN_POINT('Ctrl Pts',(14.4998913569851,-41.0003114357332,19.0181145441214));
#16107=CARTESIAN_POINT('Ctrl Pts',(14.4998972483194,-41.0002995822785,19.0176308540144));
#16108=CARTESIAN_POINT('Ctrl Pts',(14.4999147420325,-41.0002622818382,19.0159905547722));
#16109=CARTESIAN_POINT('Ctrl Pts',(14.4999222406152,-41.000246293212,19.0152874496266));
#16110=CARTESIAN_POINT('Ctrl Pts',(14.4999316961465,-41.0002258364841,19.0143718261369));
#16111=CARTESIAN_POINT('Ctrl Pts',(14.499943037045,-41.0001992580938,19.0130708039746));
#16112=CARTESIAN_POINT('Ctrl Pts',(14.4999813878673,-41.0001093795772,19.0086712169236));
#16113=CARTESIAN_POINT('Ctrl Pts',(14.4999919153304,-41.0000539915017,19.0053844424774));
#16114=CARTESIAN_POINT('Ctrl Pts',(14.4999965710787,-41.0000280644151,19.003207173894));
#16115=CARTESIAN_POINT('Ctrl Pts',(14.5000010927214,-41.0000028841408,19.0010926200623));
#16116=CARTESIAN_POINT('Ctrl Pts',(14.5,-41.0000001237228,19.0000246345942));
#16117=CARTESIAN_POINT('Ctrl Pts',(14.5,-41.,19.));
#16118=CARTESIAN_POINT('Origin',(-14.5,-42.5,-20.5));
#16119=CARTESIAN_POINT('',(13.5,-42.5,17.));
#16120=CARTESIAN_POINT('',(13.4999999999999,-42.4999999999994,18.4999999994848));
#16121=CARTESIAN_POINT('',(13.5,-42.5,-20.5));
#16122=CARTESIAN_POINT('Ctrl Pts',(13.4999999999999,-42.4999999999986,18.4999999994848));
#16123=CARTESIAN_POINT('Ctrl Pts',(13.5000000000266,-42.4999999999987,18.5175482730347));
#16124=CARTESIAN_POINT('Ctrl Pts',(13.4986337558358,-42.5000000000026,18.5351573548439));
#16125=CARTESIAN_POINT('Ctrl Pts',(13.4959747613953,-42.4999999999946,18.5528292058201));
#16126=CARTESIAN_POINT('Ctrl Pts',(13.4941761705346,-42.4999999999891,18.5647827583261));
#16127=CARTESIAN_POINT('Ctrl Pts',(13.4917848454981,-42.4999999999802,18.5767650851484));
#16128=CARTESIAN_POINT('Ctrl Pts',(13.4888102900511,-42.499999999916,18.5887750039491));
#16129=CARTESIAN_POINT('Ctrl Pts',(13.4863781587337,-42.4999999998636,18.5985948577578));
#16130=CARTESIAN_POINT('Ctrl Pts',(13.4834985579312,-42.4999999998589,18.6086211899905));
#16131=CARTESIAN_POINT('Ctrl Pts',(13.4802054497616,-42.4999999998767,18.6186663958456));
#16132=CARTESIAN_POINT('Ctrl Pts',(13.4768015227683,-42.4999999998951,18.6290496403681));
#16133=CARTESIAN_POINT('Ctrl Pts',(13.4729558419144,-42.4999999999242,18.6394525253292));
#16134=CARTESIAN_POINT('Ctrl Pts',(13.4687628721224,-42.4999999999245,18.6496758796856));
#16135=CARTESIAN_POINT('Ctrl Pts',(13.4647167019552,-42.4999999999248,18.6595413052567));
#16136=CARTESIAN_POINT('Ctrl Pts',(13.4603480054249,-42.4999999999231,18.6692392546691));
#16137=CARTESIAN_POINT('Ctrl Pts',(13.4557857876007,-42.499999999774,18.6786040936032));
#16138=CARTESIAN_POINT('Ctrl Pts',(13.4451257644337,-42.4999999994256,18.7004858633564));
#16139=CARTESIAN_POINT('Ctrl Pts',(13.4327339021801,-42.4999999992441,18.7218831631332));
#16140=CARTESIAN_POINT('Ctrl Pts',(13.4187879601852,-42.4999999993707,18.7426611284788));
#16141=CARTESIAN_POINT('Ctrl Pts',(13.4045377764472,-42.4999999995,18.7638923815546));
#16142=CARTESIAN_POINT('Ctrl Pts',(13.3886636880513,-42.499999999749,18.7844784249754));
#16143=CARTESIAN_POINT('Ctrl Pts',(13.3713104340802,-42.4999999997995,18.8042484071092));
#16144=CARTESIAN_POINT('Ctrl Pts',(13.3614729450939,-42.499999999828,18.8154559294462));
#16145=CARTESIAN_POINT('Ctrl Pts',(13.3511593888156,-42.4999999998311,18.8264005904639));
#16146=CARTESIAN_POINT('Ctrl Pts',(13.3403924032599,-42.4999999996694,18.8370447253153));
#16147=CARTESIAN_POINT('Ctrl Pts',(13.3283055921268,-42.4999999994878,18.848993626608));
#16148=CARTESIAN_POINT('Ctrl Pts',(13.3159610585321,-42.4999999993708,18.8602430590866));
#16149=CARTESIAN_POINT('Ctrl Pts',(13.303331566112,-42.499999999374,18.8708954642608));
#16150=CARTESIAN_POINT('Ctrl Pts',(13.2909314512315,-42.4999999993771,18.8813543998633));
#16151=CARTESIAN_POINT('Ctrl Pts',(13.2782554811413,-42.499999999477,18.8912384137336));
#16152=CARTESIAN_POINT('Ctrl Pts',(13.2652378046748,-42.4999999995746,18.9006092703813));
#16153=CARTESIAN_POINT('Ctrl Pts',(13.2518589264016,-42.499999999675,18.9102401404316));
#16154=CARTESIAN_POINT('Ctrl Pts',(13.2381182986558,-42.4999999997664,18.9193301169329));
#16155=CARTESIAN_POINT('Ctrl Pts',(13.2239161523732,-42.4999999997977,18.9278952079878));
#16156=CARTESIAN_POINT('Ctrl Pts',(13.2110597721419,-42.4999999998261,18.935648688703));
#16157=CARTESIAN_POINT('Ctrl Pts',(13.1978243246456,-42.4999999998288,18.9429720735206));
#16158=CARTESIAN_POINT('Ctrl Pts',(13.1841254335216,-42.4999999996881,18.9498297778044));
#16159=CARTESIAN_POINT('Ctrl Pts',(13.1826914760402,-42.4999999996733,18.9505476210426));
#16160=CARTESIAN_POINT('Ctrl Pts',(13.1812524367053,-42.4999999996567,18.9512603143427));
#16161=CARTESIAN_POINT('Ctrl Pts',(13.1798082169117,-42.4999999996377,18.9519677825118));
#16162=CARTESIAN_POINT('Ctrl Pts',(13.1618474281236,-42.499999999402,18.9607660876009));
#16163=CARTESIAN_POINT('Ctrl Pts',(13.1439125685113,-42.4999999992861,18.9683362971943));
#16164=CARTESIAN_POINT('Ctrl Pts',(13.1260291942023,-42.4999999993601,18.9747217350995));
#16165=CARTESIAN_POINT('Ctrl Pts',(13.1083133090592,-42.4999999994334,18.9810473693206));
#16166=CARTESIAN_POINT('Ctrl Pts',(13.0906467851646,-42.4999999996451,18.9862110000933));
#16167=CARTESIAN_POINT('Ctrl Pts',(13.0730280313959,-42.4999999997876,18.990211796952));
#16168=CARTESIAN_POINT('Ctrl Pts',(13.0561751561859,-42.4999999999239,18.9940386811394));
#16169=CARTESIAN_POINT('Ctrl Pts',(13.0393650740392,-42.4999999999852,18.9968019370571));
#16170=CARTESIAN_POINT('Ctrl Pts',(13.0225870886961,-42.4999999999965,18.9984547549262));
#16171=CARTESIAN_POINT('Ctrl Pts',(13.0150519404101,-42.5000000000015,18.9991970507072));
#16172=CARTESIAN_POINT('Ctrl Pts',(13.0075232175578,-42.5000000000005,18.9997147100955));
#16173=CARTESIAN_POINT('Ctrl Pts',(13.,-42.5000000000005,19.));
#16174=CARTESIAN_POINT('',(-13.5,-42.5000000000008,18.4999999994861));
#16175=CARTESIAN_POINT('Ctrl Pts',(-13.5,-42.5000000000019,18.4999999994861));
#16176=CARTESIAN_POINT('Ctrl Pts',(-13.5000000003688,-42.5000000000027,
18.7411872045822));
#16177=CARTESIAN_POINT('Ctrl Pts',(-13.2411750364478,-42.5000000000008,
18.9975772517629));
#16178=CARTESIAN_POINT('Ctrl Pts',(-13.,-42.5000000000013,18.9999999999985));
#16179=CARTESIAN_POINT('',(-13.5,-42.5,17.));
#16180=CARTESIAN_POINT('',(-13.5,-42.5,-20.5));
#16181=CARTESIAN_POINT('',(-14.5,-42.5,17.));
#16182=CARTESIAN_POINT('Origin',(-13.,-41.,19.));
#16183=CARTESIAN_POINT('Ctrl Pts',(-14.5000000000002,-41.,18.9999999095867));
#16184=CARTESIAN_POINT('Ctrl Pts',(-14.5,-41.0002683704709,19.0070720742973));
#16185=CARTESIAN_POINT('Ctrl Pts',(-14.5008952119788,-41.0008162323375,
19.0450824562715));
#16186=CARTESIAN_POINT('Ctrl Pts',(-14.4931017851684,-41.0110134479768,
19.1473283609849));
#16187=CARTESIAN_POINT('Ctrl Pts',(-14.4888014238237,-41.0161476273397,
19.1889301853449));
#16188=CARTESIAN_POINT('Ctrl Pts',(-14.4769322259473,-41.0289667632409,
19.2616359812436));
#16189=CARTESIAN_POINT('Ctrl Pts',(-14.4720622413127,-41.0341016700835,
19.2875788666429));
#16190=CARTESIAN_POINT('Ctrl Pts',(-14.4629416839819,-41.0434746813108,
19.3288153342504));
#16191=CARTESIAN_POINT('Ctrl Pts',(-14.457926662538,-41.0485793737959,19.3500126255628));
#16192=CARTESIAN_POINT('Ctrl Pts',(-14.4511743173683,-41.0553534003836,
19.3756863417945));
#16193=CARTESIAN_POINT('Ctrl Pts',(-14.4480754803318,-41.0584413889369,
19.3868828151956));
#16194=CARTESIAN_POINT('Ctrl Pts',(-14.4459627179151,-41.0605421677126,
19.3943891095111));
#16195=CARTESIAN_POINT('Ctrl Pts',(-14.4444040881135,-41.0620877097344,
19.3998091262352));
#16196=CARTESIAN_POINT('Ctrl Pts',(-14.4237756906892,-41.082512704408,19.470717215942));
#16197=CARTESIAN_POINT('Ctrl Pts',(-14.3993690637951,-41.1063530632061,
19.5340649357977));
#16198=CARTESIAN_POINT('Ctrl Pts',(-14.3583270196759,-41.1468285268692,
19.6201464487667));
#16199=CARTESIAN_POINT('Ctrl Pts',(-14.3439056403296,-41.1611049530719,
19.6473572697789));
#16200=CARTESIAN_POINT('Ctrl Pts',(-14.3139153763818,-41.1909975274763,
19.6987524160638));
#16201=CARTESIAN_POINT('Ctrl Pts',(-14.2976357723493,-41.2073325510989,
19.7239445601018));
#16202=CARTESIAN_POINT('Ctrl Pts',(-14.2518083414019,-41.2536918915089,
19.788911112031));
#16203=CARTESIAN_POINT('Ctrl Pts',(-14.2168974150804,-41.2896437989156,
19.8306766770144));
#16204=CARTESIAN_POINT('Ctrl Pts',(-14.1571767183321,-41.3517717037646,
19.8879120782401));
#16205=CARTESIAN_POINT('Ctrl Pts',(-14.1360457868065,-41.373839332279,19.9060806952706));
#16206=CARTESIAN_POINT('Ctrl Pts',(-14.0912261827393,-41.4206695624726,
19.9400003402846));
#16207=CARTESIAN_POINT('Ctrl Pts',(-14.0688649668164,-41.4440503251661,
19.9549959653011));
#16208=CARTESIAN_POINT('Ctrl Pts',(-13.9898492874905,-41.5263333774401,
19.9999263838317));
#16209=CARTESIAN_POINT('Ctrl Pts',(-13.9384829545777,-41.5789080828669,
20.0192563633802));
#16210=CARTESIAN_POINT('Ctrl Pts',(-13.866731070959,-41.6514471380887,20.0371046073534));
#16211=CARTESIAN_POINT('Ctrl Pts',(-13.8436826949272,-41.6745978993848,
20.0411970669137));
#16212=CARTESIAN_POINT('Ctrl Pts',(-13.8107160108182,-41.707607683097,20.0451193489531));
#16213=CARTESIAN_POINT('Ctrl Pts',(-13.7946330526831,-41.7236851791086,
20.0465257906122));
#16214=CARTESIAN_POINT('Ctrl Pts',(-13.7766256908422,-41.7416724003402,
20.0473128143693));
#16215=CARTESIAN_POINT('Ctrl Pts',(-13.7690755742822,-41.7492147607254,
20.0474791032033));
#16216=CARTESIAN_POINT('Ctrl Pts',(-13.7640799210929,-41.754205865215,20.0475532708898));
#16217=CARTESIAN_POINT('Ctrl Pts',(-13.7625698364561,-41.7557145519479,
20.0475716004369));
#16218=CARTESIAN_POINT('Ctrl Pts',(-13.6494244217153,-41.8687938800138,
20.047619490084));
#16219=CARTESIAN_POINT('Ctrl Pts',(-13.5458171257079,-41.9707644713532,
20.014226165779));
#16220=CARTESIAN_POINT('Ctrl Pts',(-13.4098535901852,-42.1031060930784,
19.9326926928269));
#16221=CARTESIAN_POINT('Ctrl Pts',(-13.3676863827572,-42.1439053577592,
19.9002696352513));
#16222=CARTESIAN_POINT('Ctrl Pts',(-13.3098169226224,-42.1998618651295,
19.8458099780668));
#16223=CARTESIAN_POINT('Ctrl Pts',(-13.2914204068261,-42.2176450616891,
19.8266825482741));
#16224=CARTESIAN_POINT('Ctrl Pts',(-13.2652190679525,-42.2430175435658,
19.796751892831));
#16225=CARTESIAN_POINT('Ctrl Pts',(-13.2567173583245,-42.2512581854533,
19.7865681729868));
#16226=CARTESIAN_POINT('Ctrl Pts',(-13.240185134444,-42.2673080364076,19.7658209853051));
#16227=CARTESIAN_POINT('Ctrl Pts',(-13.2329761306684,-42.2743164823624,
19.7563895777004));
#16228=CARTESIAN_POINT('Ctrl Pts',(-13.1899088809412,-42.3162962602579,
19.6970422219206));
#16229=CARTESIAN_POINT('Ctrl Pts',(-13.1591326285696,-42.3469593113915,
19.644299869016));
#16230=CARTESIAN_POINT('Ctrl Pts',(-13.1187018339568,-42.387576618264,19.5583253785839));
#16231=CARTESIAN_POINT('Ctrl Pts',(-13.1061787094213,-42.4002185564297,
19.5285226500102));
#16232=CARTESIAN_POINT('Ctrl Pts',(-13.0830590577013,-42.4235267889694,
19.4667920197459));
#16233=CARTESIAN_POINT('Ctrl Pts',(-13.0729799647175,-42.4336781543728,
19.4366329174016));
#16234=CARTESIAN_POINT('Ctrl Pts',(-13.0222535327245,-42.4841587298348,
19.2632423352929));
#16235=CARTESIAN_POINT('Ctrl Pts',(-13.0012852487877,-42.5,19.1269410506494));
#16236=CARTESIAN_POINT('Ctrl Pts',(-13.,-42.5000000000004,18.9999999999985));
#16237=CARTESIAN_POINT('Origin',(-14.5,13.,-20.5));
#16238=CARTESIAN_POINT('',(-14.5,11.5,17.));
#16239=CARTESIAN_POINT('',(-14.5,11.5,-20.5));
#16240=CARTESIAN_POINT('',(-14.5,-41.5,17.));
#16241=CARTESIAN_POINT('',(-14.5,13.,17.));
#16242=CARTESIAN_POINT('',(-14.4999999999994,-41.4999999999999,18.4999999994854));
#16243=CARTESIAN_POINT('',(-14.5,-41.5,-20.5));
#16244=CARTESIAN_POINT('Ctrl Pts',(-14.4999999999986,-41.5,18.4999999994854));
#16245=CARTESIAN_POINT('Ctrl Pts',(-14.4999999999987,-41.5000000000266,
18.5175482730428));
#16246=CARTESIAN_POINT('Ctrl Pts',(-14.5000000000027,-41.4986337558346,
18.5351573548596));
#16247=CARTESIAN_POINT('Ctrl Pts',(-14.4999999999946,-41.4959747613919,
18.5528292058435));
#16248=CARTESIAN_POINT('Ctrl Pts',(-14.4999999999891,-41.4941761705316,
18.564782758342));
#16249=CARTESIAN_POINT('Ctrl Pts',(-14.4999999999802,-41.4917848454962,
18.5767650851567));
#16250=CARTESIAN_POINT('Ctrl Pts',(-14.499999999916,-41.4888102900512,18.5887750039498));
#16251=CARTESIAN_POINT('Ctrl Pts',(-14.4999999998636,-41.4863781587332,
18.5985948577608));
#16252=CARTESIAN_POINT('Ctrl Pts',(-14.4999999998589,-41.4834985579299,
18.6086211899957));
#16253=CARTESIAN_POINT('Ctrl Pts',(-14.4999999998767,-41.4802054497594,
18.618666395853));
#16254=CARTESIAN_POINT('Ctrl Pts',(-14.4999999998951,-41.4768015227651,
18.6290496403776));
#16255=CARTESIAN_POINT('Ctrl Pts',(-14.4999999999242,-41.4729558419101,
18.6394525253408));
#16256=CARTESIAN_POINT('Ctrl Pts',(-14.4999999999246,-41.4687628721168,
18.6496758796993));
#16257=CARTESIAN_POINT('Ctrl Pts',(-14.4999999999249,-41.4647167019513,
18.6595413052655));
#16258=CARTESIAN_POINT('Ctrl Pts',(-14.4999999999231,-41.4603480054228,
18.6692392546731));
#16259=CARTESIAN_POINT('Ctrl Pts',(-14.499999999774,-41.4557857876006,18.6786040936032));
#16260=CARTESIAN_POINT('Ctrl Pts',(-14.4999999994256,-41.445125764451,18.7004858633204));
#16261=CARTESIAN_POINT('Ctrl Pts',(-14.4999999992441,-41.4327339022211,
18.721883163062));
#16262=CARTESIAN_POINT('Ctrl Pts',(-14.4999999993707,-41.4187879602549,
18.7426611283747));
#16263=CARTESIAN_POINT('Ctrl Pts',(-14.4999999995,-41.4045377765463,18.7638923814168));
#16264=CARTESIAN_POINT('Ctrl Pts',(-14.499999999749,-41.388663688185,18.7844784248062));
#16265=CARTESIAN_POINT('Ctrl Pts',(-14.4999999997995,-41.3713104342529,
18.8042484069122));
#16266=CARTESIAN_POINT('Ctrl Pts',(-14.4999999998281,-41.3614729452147,
18.8154559293178));
#16267=CARTESIAN_POINT('Ctrl Pts',(-14.4999999998311,-41.3511593888788,
18.8264005904013));
#16268=CARTESIAN_POINT('Ctrl Pts',(-14.4999999996694,-41.3403924032599,
18.8370447253151));
#16269=CARTESIAN_POINT('Ctrl Pts',(-14.4999999994878,-41.3283055921264,
18.848993626608));
#16270=CARTESIAN_POINT('Ctrl Pts',(-14.4999999993708,-41.3159610585317,
18.8602430590867));
#16271=CARTESIAN_POINT('Ctrl Pts',(-14.499999999374,-41.3033315661115,18.8708954642609));
#16272=CARTESIAN_POINT('Ctrl Pts',(-14.4999999993771,-41.2909314512325,
18.8813543998622));
#16273=CARTESIAN_POINT('Ctrl Pts',(-14.499999999477,-41.2782554811439,18.8912384137313));
#16274=CARTESIAN_POINT('Ctrl Pts',(-14.4999999995746,-41.2652378046791,
18.900609270378));
#16275=CARTESIAN_POINT('Ctrl Pts',(-14.499999999675,-41.2518589264053,18.910240140429));
#16276=CARTESIAN_POINT('Ctrl Pts',(-14.4999999997664,-41.2381182986589,
18.9193301169308));
#16277=CARTESIAN_POINT('Ctrl Pts',(-14.4999999997977,-41.2239161523756,
18.9278952079862));
#16278=CARTESIAN_POINT('Ctrl Pts',(-14.4999999998261,-41.211059772146,18.9356486887005));
#16279=CARTESIAN_POINT('Ctrl Pts',(-14.4999999998288,-41.1978243246514,
18.9429720735174));
#16280=CARTESIAN_POINT('Ctrl Pts',(-14.4999999996881,-41.1841254335292,
18.9498297778006));
#16281=CARTESIAN_POINT('Ctrl Pts',(-14.4999999996733,-41.1826914760453,
18.95054762104));
#16282=CARTESIAN_POINT('Ctrl Pts',(-14.4999999996567,-41.1812524367078,
18.9512603143414));
#16283=CARTESIAN_POINT('Ctrl Pts',(-14.4999999996378,-41.1798082169117,
18.9519677825117));
#16284=CARTESIAN_POINT('Ctrl Pts',(-14.499999999402,-41.161847433483,18.9607660849755));
#16285=CARTESIAN_POINT('Ctrl Pts',(-14.4999999992861,-41.1439125794643,
18.9683362925574));
#16286=CARTESIAN_POINT('Ctrl Pts',(-14.4999999993601,-41.1260292108387,
18.9747217291591));
#16287=CARTESIAN_POINT('Ctrl Pts',(-14.4999999994335,-41.108313331451,18.9810473620443));
#16288=CARTESIAN_POINT('Ctrl Pts',(-14.4999999996451,-41.0906468133997,
18.9862109921918));
#16289=CARTESIAN_POINT('Ctrl Pts',(-14.4999999997876,-41.0730280654294,
18.9902117892228));
#16290=CARTESIAN_POINT('Ctrl Pts',(-14.4999999999239,-41.0561751957912,
18.9940386735692));
#16291=CARTESIAN_POINT('Ctrl Pts',(-14.4999999999852,-41.0393651191756,
18.9968019303783));
#16292=CARTESIAN_POINT('Ctrl Pts',(-14.4999999999965,-41.0225871392088,
18.9984547499492));
#16293=CARTESIAN_POINT('Ctrl Pts',(-14.5000000000015,-41.0150519763219,
18.9991970481707));
#16294=CARTESIAN_POINT('Ctrl Pts',(-14.5000000000006,-41.0075232388665,
18.9997147091494));
#16295=CARTESIAN_POINT('Ctrl Pts',(-14.5000000000005,-41.0000000066869,
18.9999999997464));
#16296=CARTESIAN_POINT('Origin',(-13.94140536675,11.,17.13971317669));
#16297=CARTESIAN_POINT('',(-15.5952583708893,12.1246200428121,14.5));
#16298=CARTESIAN_POINT('',(-15.5952583708895,12.1246200428123,17.));
#16299=CARTESIAN_POINT('',(-15.5952583708915,12.124620042811,17.13971317669));
#16300=CARTESIAN_POINT('Origin',(-13.94140536675,11.,17.));
#16301=CARTESIAN_POINT('Origin',(-13.94140536675,11.,14.5));
#16302=CARTESIAN_POINT('Origin',(-12.5,11.,20.63971317669));
#16303=CARTESIAN_POINT('',(-14.5,11.,-14.5));
#16304=CARTESIAN_POINT('',(-14.5,11.,14.5));
#16305=CARTESIAN_POINT('',(-14.5,11.,20.63971317669));
#16306=CARTESIAN_POINT('Origin',(-12.5,11.,14.5));
#16307=CARTESIAN_POINT('Origin',(-12.5,11.,-14.5));
#16308=CARTESIAN_POINT('Origin',(-13.94140536675,11.,-12.36535464022));
#16309=CARTESIAN_POINT('',(-15.5952583708895,12.1246200428123,-17.));
#16310=CARTESIAN_POINT('',(-15.5952583708896,12.1246200428122,-14.5));
#16311=CARTESIAN_POINT('',(-15.5952583708915,12.124620042811,-12.36535464022));
#16312=CARTESIAN_POINT('Origin',(-13.94140536675,11.,-14.5));
#16313=CARTESIAN_POINT('Origin',(-13.94140536675,11.,-17.));
#16314=CARTESIAN_POINT('Origin',(0.,0.,-17.));
#16315=CARTESIAN_POINT('',(20.1,-39.67662948547,-17.));
#16316=CARTESIAN_POINT('',(20.1,4.576629485471,-17.));
#16317=CARTESIAN_POINT('',(20.1,0.,-17.));
#16318=CARTESIAN_POINT('',(19.5807795062094,-41.3635595496909,-17.));
#16319=CARTESIAN_POINT('Origin',(17.1,-39.67662948547,-17.));
#16320=CARTESIAN_POINT('',(15.8928875563296,-46.786930064221,-17.));
#16321=CARTESIAN_POINT('',(15.89288755633,-46.78693006422,-17.));
#16322=CARTESIAN_POINT('',(13.41210805012,-48.1,-17.));
#16323=CARTESIAN_POINT('Origin',(13.41210805012,-45.1,-17.));
#16324=CARTESIAN_POINT('',(-13.41210805012,-48.1,-17.));
#16325=CARTESIAN_POINT('',(0.,-48.1,-17.));
#16326=CARTESIAN_POINT('',(-15.8928875563294,-46.7869300642209,-17.));
#16327=CARTESIAN_POINT('Origin',(-13.41210805012,-45.1,-17.));
#16328=CARTESIAN_POINT('',(-19.5807795062097,-41.3635595496911,-17.));
#16329=CARTESIAN_POINT('',(-19.58077950621,-41.36355954969,-17.));
#16330=CARTESIAN_POINT('',(-20.1,-39.67662948547,-17.));
#16331=CARTESIAN_POINT('Origin',(-17.1,-39.67662948547,-17.));
#16332=CARTESIAN_POINT('',(-20.1,4.576629485471,-17.));
#16333=CARTESIAN_POINT('',(-20.1,0.,-17.));
#16334=CARTESIAN_POINT('',(-19.5807795062095,6.26355954969313,-17.));
#16335=CARTESIAN_POINT('Origin',(-17.1,4.576629485471,-17.));
#16336=CARTESIAN_POINT('',(-15.59525837089,12.12462004281,-17.));
#16337=CARTESIAN_POINT('',(-8.15,11.5,-17.));
#16338=CARTESIAN_POINT('Origin',(-6.65,11.5,-17.));
#16339=CARTESIAN_POINT('',(-8.15,9.,-17.));
#16340=CARTESIAN_POINT('',(-8.15,0.,-17.));
#16341=CARTESIAN_POINT('',(-10.5,6.65,-17.));
#16342=CARTESIAN_POINT('Origin',(-10.5,9.,-17.));
#16343=CARTESIAN_POINT('',(-13.5,6.65,-17.));
#16344=CARTESIAN_POINT('',(0.,6.65,-17.));
#16345=CARTESIAN_POINT('',(-14.5,5.65,-17.));
#16346=CARTESIAN_POINT('Origin',(-13.5,5.65,-17.));
#16347=CARTESIAN_POINT('',(-14.5,-35.15,-17.));
#16348=CARTESIAN_POINT('',(-14.5,0.,-17.));
#16349=CARTESIAN_POINT('',(-13.5,-36.15,-17.));
#16350=CARTESIAN_POINT('Origin',(-13.5,-35.15,-17.));
#16351=CARTESIAN_POINT('',(-10.5,-36.15,-17.));
#16352=CARTESIAN_POINT('',(0.,-36.15,-17.));
#16353=CARTESIAN_POINT('',(-8.15,-38.5,-17.));
#16354=CARTESIAN_POINT('Origin',(-10.5,-38.5,-17.));
#16355=CARTESIAN_POINT('',(-8.15,-41.5,-17.));
#16356=CARTESIAN_POINT('',(-8.15,0.,-17.));
#16357=CARTESIAN_POINT('',(-7.15,-42.5,-17.));
#16358=CARTESIAN_POINT('Origin',(-7.15,-41.5,-17.));
#16359=CARTESIAN_POINT('',(7.15,-42.5,-17.));
#16360=CARTESIAN_POINT('',(0.,-42.5,-17.));
#16361=CARTESIAN_POINT('',(8.15,-41.5,-17.));
#16362=CARTESIAN_POINT('Origin',(7.15,-41.5,-17.));
#16363=CARTESIAN_POINT('',(8.15,-38.5,-17.));
#16364=CARTESIAN_POINT('',(8.15,0.,-17.));
#16365=CARTESIAN_POINT('',(10.5,-36.15,-17.));
#16366=CARTESIAN_POINT('Origin',(10.5,-38.5,-17.));
#16367=CARTESIAN_POINT('',(13.5,-36.15,-17.));
#16368=CARTESIAN_POINT('',(0.,-36.15,-17.));
#16369=CARTESIAN_POINT('',(14.5,-35.15,-17.));
#16370=CARTESIAN_POINT('Origin',(13.5,-35.15,-17.));
#16371=CARTESIAN_POINT('',(14.5,5.65,-17.));
#16372=CARTESIAN_POINT('',(14.5,0.,-17.));
#16373=CARTESIAN_POINT('',(13.5,6.65,-17.));
#16374=CARTESIAN_POINT('Origin',(13.5,5.65,-17.));
#16375=CARTESIAN_POINT('',(10.5,6.65,-17.));
#16376=CARTESIAN_POINT('',(0.,6.65,-17.));
#16377=CARTESIAN_POINT('',(8.15,9.000000000459,-17.));
#16378=CARTESIAN_POINT('Origin',(10.5,9.,-17.));
#16379=CARTESIAN_POINT('',(8.15,11.5,-17.));
#16380=CARTESIAN_POINT('',(8.15,0.,-17.));
#16381=CARTESIAN_POINT('Origin',(6.64999999999999,11.5,-17.));
#16382=CARTESIAN_POINT('',(15.5952583708895,12.1246200428123,-17.));
#16383=CARTESIAN_POINT('Origin',(13.94140536675,11.,-17.));
#16384=CARTESIAN_POINT('',(19.5807795062092,6.26355954969299,-17.));
#16385=CARTESIAN_POINT('',(19.58077950621,6.263559549693,-17.));
#16386=CARTESIAN_POINT('Origin',(17.1,4.576629485471,-17.));
#16387=CARTESIAN_POINT('Origin',(-14.64391314335,9.5,-17.));
#16388=CARTESIAN_POINT('',(-6.65,9.5,-20.5));
#16389=CARTESIAN_POINT('Origin',(-6.65,9.5,-17.));
#16390=CARTESIAN_POINT('',(6.650000000118,9.5,-20.5));
#16391=CARTESIAN_POINT('Origin',(6.65,9.5,-17.));
#16392=CARTESIAN_POINT('',(-14.64391314335,9.5,-20.5));
#16393=CARTESIAN_POINT('Origin',(13.94140536675,11.,-12.38062237617));
#16394=CARTESIAN_POINT('',(15.5952583708891,12.124620042812,-14.5));
#16395=CARTESIAN_POINT('Origin',(13.94140536675,11.,-14.5));
#16396=CARTESIAN_POINT('',(15.5952583708915,12.124620042811,-12.38062237617));
#16397=CARTESIAN_POINT('Origin',(12.5,11.,20.63971317669));
#16398=CARTESIAN_POINT('',(14.5,11.,14.5));
#16399=CARTESIAN_POINT('Origin',(12.5,11.,14.5));
#16400=CARTESIAN_POINT('',(14.5,11.,-14.5));
#16401=CARTESIAN_POINT('',(14.5,11.,20.63971317669));
#16402=CARTESIAN_POINT('Origin',(12.5,11.,-14.5));
#16403=CARTESIAN_POINT('Origin',(13.94140536675,11.,17.20607693562));
#16404=CARTESIAN_POINT('',(15.5952583708895,12.1246200428123,17.));
#16405=CARTESIAN_POINT('Origin',(13.94140536675,11.,17.));
#16406=CARTESIAN_POINT('',(15.5952583708896,12.1246200428122,14.5));
#16407=CARTESIAN_POINT('',(15.5952583708915,12.124620042811,17.20607693562));
#16408=CARTESIAN_POINT('Origin',(13.94140536675,11.,14.5));
#16409=CARTESIAN_POINT('Origin',(13.,11.5,18.63971317669));
#16410=CARTESIAN_POINT('Origin',(13.,11.5,17.));
#16411=CARTESIAN_POINT('Origin',(-13.,11.5,-17.13464535978));
#16412=CARTESIAN_POINT('Origin',(-13.,11.5,17.));
#16413=CARTESIAN_POINT('Origin',(0.,0.,17.));
#16414=CARTESIAN_POINT('',(19.5807795062093,-41.3635595496909,17.));
#16415=CARTESIAN_POINT('',(20.1,-39.67662948547,17.));
#16416=CARTESIAN_POINT('Origin',(17.1,-39.67662948547,17.));
#16417=CARTESIAN_POINT('',(20.1,4.576629485471,17.));
#16418=CARTESIAN_POINT('',(20.1,0.,17.));
#16419=CARTESIAN_POINT('',(19.5807795062093,6.26355954969304,17.));
#16420=CARTESIAN_POINT('Origin',(17.1,4.576629485471,17.));
#16421=CARTESIAN_POINT('',(19.58077950621,6.263559549693,17.));
#16422=CARTESIAN_POINT('Origin',(13.5,-41.5,17.));
#16423=CARTESIAN_POINT('Origin',(-13.5,-41.5,17.));
#16424=CARTESIAN_POINT('',(-19.5807795062095,6.26355954969313,17.));
#16425=CARTESIAN_POINT('',(-15.59525837089,12.12462004281,17.));
#16426=CARTESIAN_POINT('',(-20.1,4.576629485471,17.));
#16427=CARTESIAN_POINT('Origin',(-17.1,4.576629485471,17.));
#16428=CARTESIAN_POINT('',(-20.1,-39.67662948547,17.));
#16429=CARTESIAN_POINT('',(-20.1,0.,17.));
#16430=CARTESIAN_POINT('',(-19.5807795062097,-41.3635595496911,17.));
#16431=CARTESIAN_POINT('Origin',(-17.1,-39.67662948547,17.));
#16432=CARTESIAN_POINT('',(-15.8928875563294,-46.7869300642209,17.));
#16433=CARTESIAN_POINT('',(-19.58077950621,-41.36355954969,17.));
#16434=CARTESIAN_POINT('',(-13.41210805012,-48.1,17.));
#16435=CARTESIAN_POINT('Origin',(-13.41210805012,-45.1,17.));
#16436=CARTESIAN_POINT('',(13.41210805012,-48.1,17.));
#16437=CARTESIAN_POINT('',(0.,-48.1,17.));
#16438=CARTESIAN_POINT('',(15.8928875563296,-46.786930064221,17.));
#16439=CARTESIAN_POINT('Origin',(13.41210805012,-45.1,17.));
#16440=CARTESIAN_POINT('',(15.89288755633,-46.78693006422,17.));
#16441=CARTESIAN_POINT('Origin',(13.5,-41.5,20.63971317669));
#16442=CARTESIAN_POINT('Origin',(13.5,-41.5,18.4999999994851));
#16443=CARTESIAN_POINT('Ctrl Pts',(14.5000000000013,-40.9943380969227,19.0000100692442));
#16444=CARTESIAN_POINT('Ctrl Pts',(14.5000000000008,-41.2371059113903,19.0015933091084));
#16445=CARTESIAN_POINT('Ctrl Pts',(14.5000000000027,-41.5000000009281,18.7430757267126));
#16446=CARTESIAN_POINT('Ctrl Pts',(14.5000000000019,-41.5,18.4999999987137));
#16447=CARTESIAN_POINT('Ctrl Pts',(14.5000000000028,-40.995317328355,19.1412652085388));
#16448=CARTESIAN_POINT('Ctrl Pts',(14.5000000000014,-41.2564831044291,19.0954746833564));
#16449=CARTESIAN_POINT('Ctrl Pts',(14.5000000000026,-41.5369365607809,18.7901585471376));
#16450=CARTESIAN_POINT('Ctrl Pts',(14.5000000000014,-41.565449847102,18.4999999984638));
#16451=CARTESIAN_POINT('Ctrl Pts',(14.461088950263,-41.0396947394679,19.4141933256417));
#16452=CARTESIAN_POINT('Ctrl Pts',(14.4808879882492,-41.3232890737612,19.2739493035027));
#16453=CARTESIAN_POINT('Ctrl Pts',(14.4987197414757,-41.622688121818,18.8825190881865));
#16454=CARTESIAN_POINT('Ctrl Pts',(14.4871066327079,-41.6963473912737,18.4999999979725));
#16455=CARTESIAN_POINT('Ctrl Pts',(14.2951753510104,-41.2092320493177,19.7671081794723));
#16456=CARTESIAN_POINT('Ctrl Pts',(14.3829355447186,-41.4926490904922,19.5234352013656));
#16457=CARTESIAN_POINT('Ctrl Pts',(14.466126570005,-41.798927508403,18.9987393235418));
#16458=CARTESIAN_POINT('Ctrl Pts',(14.4298332811675,-41.8851496535818,18.4999999973609));
#16459=CARTESIAN_POINT('Ctrl Pts',(14.0470778370451,-41.4604801612305,20.0000694996508));
#16460=CARTESIAN_POINT('Ctrl Pts',(14.208692992919,-41.7204167792393,19.7008597170388));
#16461=CARTESIAN_POINT('Ctrl Pts',(14.373854422343,-42.0097950503571,19.0757337060923));
#16462=CARTESIAN_POINT('Ctrl Pts',(14.3368285937893,-42.059150964628,18.4999999969561));
#16463=CARTESIAN_POINT('Ctrl Pts',(13.7542691791144,-41.7542035734038,20.0822650788914));
#16464=CARTESIAN_POINT('Ctrl Pts',(13.9755845401677,-41.9754027621767,19.7657545358299));
#16465=CARTESIAN_POINT('Ctrl Pts',(14.2147126834794,-42.214781365487,19.1045289473882));
#16466=CARTESIAN_POINT('Ctrl Pts',(14.2116652821725,-42.2116652821764,18.4999999967981));
#16467=CARTESIAN_POINT('Ctrl Pts',(13.4602188374819,-42.0470674075824,20.0001437555219));
#16468=CARTESIAN_POINT('Ctrl Pts',(13.7204012871743,-42.209895391559,19.6998305081936));
#16469=CARTESIAN_POINT('Ctrl Pts',(14.0099355358227,-42.373720179787,19.0761517589292));
#16470=CARTESIAN_POINT('Ctrl Pts',(14.0591509646221,-42.3368285937868,18.4999999969514));
#16471=CARTESIAN_POINT('Ctrl Pts',(13.2100966184005,-42.2951361405335,19.7669964902518));
#16472=CARTESIAN_POINT('Ctrl Pts',(13.4934675131165,-42.3844114694822,19.5204897565771));
#16473=CARTESIAN_POINT('Ctrl Pts',(13.7991208871267,-42.4661360608768,18.9989428562529));
#16474=CARTESIAN_POINT('Ctrl Pts',(13.8851496535816,-42.4298332811645,18.4999999973594));
#16475=CARTESIAN_POINT('Ctrl Pts',(13.0371194604123,-42.4610525148315,19.4147999538865));
#16476=CARTESIAN_POINT('Ctrl Pts',(13.3212465098146,-42.4824926046905,19.2710925155892));
#16477=CARTESIAN_POINT('Ctrl Pts',(13.6219561650579,-42.4987406155644,18.8812429548123));
#16478=CARTESIAN_POINT('Ctrl Pts',(13.6963473912789,-42.4871066327043,18.4999999979835));
#16479=CARTESIAN_POINT('Ctrl Pts',(12.9992279345901,-42.5000000000002,19.1406085881773));
#16480=CARTESIAN_POINT('Ctrl Pts',(13.2589309435621,-42.5000000000008,19.0886851287514));
#16481=CARTESIAN_POINT('Ctrl Pts',(13.5382388686105,-42.4999999999992,18.7898907052044));
#16482=CARTESIAN_POINT('Ctrl Pts',(13.5654498470941,-42.4999999999989,18.4999999984642));
#16483=CARTESIAN_POINT('Ctrl Pts',(12.9943419397749,-42.5000000000005,19.0001703298077));
#16484=CARTESIAN_POINT('Ctrl Pts',(13.2369423184852,-42.5000000000009,18.9947709047232));
#16485=CARTESIAN_POINT('Ctrl Pts',(13.5000000009278,-42.4999999999995,18.7430757267406));
#16486=CARTESIAN_POINT('Ctrl Pts',(13.4999999999998,-42.4999999999986,18.499999998712));
#16487=CARTESIAN_POINT('Origin',(-13.5,-41.5,20.63971317669));
#16488=CARTESIAN_POINT('Origin',(-13.5,-41.5,18.4999999994858));
#16489=CARTESIAN_POINT('Ctrl Pts',(-12.9943339615788,-42.4999998766974,
18.9993941198875));
#16490=CARTESIAN_POINT('Ctrl Pts',(-13.2370215093323,-42.4999999394458,
19.001183925909));
#16491=CARTESIAN_POINT('Ctrl Pts',(-13.4998389829741,-42.4999999959596,
18.7428704243726));
#16492=CARTESIAN_POINT('Ctrl Pts',(-13.4997146170715,-42.4999999591457,
18.4999999987164));
#16493=CARTESIAN_POINT('Ctrl Pts',(-12.9952528645595,-42.5000565171419,
19.1408685031104));
#16494=CARTESIAN_POINT('Ctrl Pts',(-13.2563860300876,-42.500027753833,19.0952152741976));
#16495=CARTESIAN_POINT('Ctrl Pts',(-13.5368119425112,-42.5000018499864,
18.7900242984701));
#16496=CARTESIAN_POINT('Ctrl Pts',(-13.5652595922869,-42.500018726424,18.4999999984663));
#16497=CARTESIAN_POINT('Ctrl Pts',(-13.0396126018465,-42.4611693322662,
19.4140223450644));
#16498=CARTESIAN_POINT('Ctrl Pts',(-13.3232070220341,-42.4809354443569,
19.2738284322996));
#16499=CARTESIAN_POINT('Ctrl Pts',(-13.6226027371649,-42.4987355322512,
18.8824627816802));
#16500=CARTESIAN_POINT('Ctrl Pts',(-13.6962559201454,-42.4871343805644,
18.4999999979752));
#16501=CARTESIAN_POINT('Ctrl Pts',(-13.2092320493188,-42.2951753510108,
19.7671081794714));
#16502=CARTESIAN_POINT('Ctrl Pts',(-13.4926490904924,-42.3829355447187,
19.5234352013648));
#16503=CARTESIAN_POINT('Ctrl Pts',(-13.7989275084019,-42.4661265700046,
18.9987393235433));
#16504=CARTESIAN_POINT('Ctrl Pts',(-13.8851496535813,-42.4298332811677,
18.499999997364));
#16505=CARTESIAN_POINT('Ctrl Pts',(-13.4604801612315,-42.0470778370458,
20.0000694996497));
#16506=CARTESIAN_POINT('Ctrl Pts',(-13.7204167792395,-42.2086929929191,
19.7008597170379));
#16507=CARTESIAN_POINT('Ctrl Pts',(-14.009795050356,-42.3738544223422,19.0757337060942));
#16508=CARTESIAN_POINT('Ctrl Pts',(-14.0591509646277,-42.3368285937896,
18.4999999969598));
#16509=CARTESIAN_POINT('Ctrl Pts',(-13.7542035734047,-41.7542691791153,
20.0822650788902));
#16510=CARTESIAN_POINT('Ctrl Pts',(-13.9754027621768,-41.9755845401679,
19.7657545358289));
#16511=CARTESIAN_POINT('Ctrl Pts',(-14.214781365486,-42.2147126834784,19.1045289473902));
#16512=CARTESIAN_POINT('Ctrl Pts',(-14.2116652821764,-42.2116652821725,
18.4999999968019));
#16513=CARTESIAN_POINT('Ctrl Pts',(-14.047067407583,-41.4602188374757,20.0001437555207));
#16514=CARTESIAN_POINT('Ctrl Pts',(-14.209895391559,-41.7204012871736,19.6998305081927));
#16515=CARTESIAN_POINT('Ctrl Pts',(-14.3737201797862,-42.0099355358214,
19.0761517589311));
#16516=CARTESIAN_POINT('Ctrl Pts',(-14.336828593787,-42.0591509646218,18.499999996955));
#16517=CARTESIAN_POINT('Ctrl Pts',(-14.2951361405339,-41.2100966184016,
19.7669964902508));
#16518=CARTESIAN_POINT('Ctrl Pts',(-14.3844114694822,-41.4934675131167,
19.5204897565763));
#16519=CARTESIAN_POINT('Ctrl Pts',(-14.4661360608765,-41.7991208871255,
18.9989428562544));
#16520=CARTESIAN_POINT('Ctrl Pts',(-14.4298332811648,-41.8851496535811,
18.4999999973626));
#16521=CARTESIAN_POINT('Ctrl Pts',(-14.4611328981796,-41.0370356562491,
19.4146293213196));
#16522=CARTESIAN_POINT('Ctrl Pts',(-14.482540123147,-41.3211630719932,19.2709716873381));
#16523=CARTESIAN_POINT('Ctrl Pts',(-14.498756411855,-41.6218703320968,18.8811859314354));
#16524=CARTESIAN_POINT('Ctrl Pts',(-14.4871343805609,-41.6962559201502,
18.4999999979862));
#16525=CARTESIAN_POINT('Ctrl Pts',(-14.5000565701147,-40.9991729022973,
19.1402100457667));
#16526=CARTESIAN_POINT('Ctrl Pts',(-14.5000254207208,-41.2588403991452,
19.0884200014296));
#16527=CARTESIAN_POINT('Ctrl Pts',(-14.5000018196287,-41.5381172084285,
18.7897579230842));
#16528=CARTESIAN_POINT('Ctrl Pts',(-14.5000187264216,-41.5652595922781,
18.4999999984667));
#16529=CARTESIAN_POINT('Ctrl Pts',(-14.4999998765811,-40.9943207243138,
18.9995579515035));
#16530=CARTESIAN_POINT('Ctrl Pts',(-14.4999999445343,-41.2368464989228,
18.9943613905473));
#16531=CARTESIAN_POINT('Ctrl Pts',(-14.4999999960226,-41.4998332897727,
18.7428715907787));
#16532=CARTESIAN_POINT('Ctrl Pts',(-14.4999999591424,-41.49971461707,18.4999999987146));
#16533=CARTESIAN_POINT('Origin',(0.,0.,23.5));
#16534=CARTESIAN_POINT('Origin',(-15.,13.,14.5));
#16535=CARTESIAN_POINT('',(-19.4370000000001,6.47500000000004,12.5));
#16536=CARTESIAN_POINT('',(-19.437,6.475,14.5));
#16537=CARTESIAN_POINT('',(-19.4370000000002,6.47500000000015,14.5));
#16538=CARTESIAN_POINT('',(-19.5807795062061,6.26355954969803,14.5));
#16539=CARTESIAN_POINT('',(-19.58077950621,6.263559549693,14.5));
#16540=CARTESIAN_POINT('',(-19.5807795062094,6.26355954969258,14.5));
#16541=CARTESIAN_POINT('',(-18.4170000000002,7.97500000000007,14.5));
#16542=CARTESIAN_POINT('',(-15.,13.,14.5));
#16543=CARTESIAN_POINT('',(-18.4170000000001,7.97500000000006,12.5));
#16544=CARTESIAN_POINT('',(-18.4170000000002,7.97500000000011,14.5));
#16545=CARTESIAN_POINT('',(-15.,13.,12.5));
#16546=CARTESIAN_POINT('Origin',(0.,0.,14.5));
#16547=CARTESIAN_POINT('',(-14.5,7.975,14.5));
#16548=CARTESIAN_POINT('',(-14.5,0.,14.5));
#16549=CARTESIAN_POINT('',(0.,7.975,14.5));
#16550=CARTESIAN_POINT('Origin',(-14.5,13.,-20.5));
#16551=CARTESIAN_POINT('',(-14.5,-40.5,12.5));
#16552=CARTESIAN_POINT('',(-14.5,-48.1,12.5));
#16553=CARTESIAN_POINT('',(-14.5,13.,12.5));
#16554=CARTESIAN_POINT('',(-14.5,-48.1,14.5));
#16555=CARTESIAN_POINT('',(-14.5,-48.1,-20.5));
#16556=CARTESIAN_POINT('',(-14.5,-47.8957988313507,14.5));
#16557=CARTESIAN_POINT('',(-14.5,13.,14.5));
#16558=CARTESIAN_POINT('',(-14.5,-21.975,14.5));
#16559=CARTESIAN_POINT('',(-14.5,13.,14.5));
#16560=CARTESIAN_POINT('',(-14.5,-21.975,12.5));
#16561=CARTESIAN_POINT('',(-14.5,-21.975,-20.5));
#16562=CARTESIAN_POINT('',(-14.5000000000001,-18.10025773881,12.5));
#16563=CARTESIAN_POINT('',(-14.5,13.,12.5));
#16564=CARTESIAN_POINT('',(-14.5,-17.89974226119,12.5));
#16565=CARTESIAN_POINT('',(-14.5,13.,12.5));
#16566=CARTESIAN_POINT('',(-14.5,-14.025,12.5));
#16567=CARTESIAN_POINT('',(-14.5,13.,12.5));
#16568=CARTESIAN_POINT('',(-14.5,-14.025,14.5));
#16569=CARTESIAN_POINT('',(-14.5,-14.025,-20.5));
#16570=CARTESIAN_POINT('',(-14.5,0.0250000000000005,14.5));
#16571=CARTESIAN_POINT('',(-14.5,13.,14.5));
#16572=CARTESIAN_POINT('',(-14.5,0.0250000000000005,12.5));
#16573=CARTESIAN_POINT('',(-14.5,0.0250000000000007,-20.5));
#16574=CARTESIAN_POINT('',(-14.4999999999997,3.89974226119284,12.5));
#16575=CARTESIAN_POINT('',(-14.5,13.,12.5));
#16576=CARTESIAN_POINT('',(-14.5,4.100257738807,12.5));
#16577=CARTESIAN_POINT('',(-14.5,13.,12.5));
#16578=CARTESIAN_POINT('',(-14.5,7.975,12.5));
#16579=CARTESIAN_POINT('',(-14.5,13.,12.5));
#16580=CARTESIAN_POINT('',(-14.5,7.975,-20.5));
#16581=CARTESIAN_POINT('',(-14.5,7.975,-14.5));
#16582=CARTESIAN_POINT('',(-14.5,13.,-14.5));
#16583=CARTESIAN_POINT('',(-14.5,7.975,-12.5));
#16584=CARTESIAN_POINT('',(-14.5,7.975,-20.5));
#16585=CARTESIAN_POINT('',(-14.500000000001,4.1002577388064,-12.5));
#16586=CARTESIAN_POINT('',(-14.5,13.,-12.5));
#16587=CARTESIAN_POINT('',(-14.5,3.899742261193,-12.5));
#16588=CARTESIAN_POINT('',(-14.5,13.,-12.5));
#16589=CARTESIAN_POINT('',(-14.5,0.0250000000000004,-12.5));
#16590=CARTESIAN_POINT('',(-14.5,13.,-12.5));
#16591=CARTESIAN_POINT('',(-14.5,0.0250000000000004,-14.5));
#16592=CARTESIAN_POINT('',(-14.5,0.0250000000000007,-20.5));
#16593=CARTESIAN_POINT('',(-14.5,-14.025,-14.5));
#16594=CARTESIAN_POINT('',(-14.5,13.,-14.5));
#16595=CARTESIAN_POINT('',(-14.5,-14.025,-12.5));
#16596=CARTESIAN_POINT('',(-14.5,-14.025,-20.5));
#16597=CARTESIAN_POINT('',(-14.5000000000011,-17.8997422611906,-12.5));
#16598=CARTESIAN_POINT('',(-14.5,13.,-12.5));
#16599=CARTESIAN_POINT('',(-14.5,-18.10025773881,-12.5));
#16600=CARTESIAN_POINT('',(-14.5,13.,-12.5));
#16601=CARTESIAN_POINT('',(-14.5,-21.75,-12.5));
#16602=CARTESIAN_POINT('',(-14.5,13.,-12.5));
#16603=CARTESIAN_POINT('',(-14.5,-21.75,-5.));
#16604=CARTESIAN_POINT('',(-14.5,-21.75,-20.5));
#16605=CARTESIAN_POINT('',(-14.5,-22.475,-5.));
#16606=CARTESIAN_POINT('',(-14.5,0.,-5.));
#16607=CARTESIAN_POINT('',(-14.5,-22.475,12.5));
#16608=CARTESIAN_POINT('',(-14.5,-22.475,-20.5));
#16609=CARTESIAN_POINT('',(-14.5,-38.525,12.5));
#16610=CARTESIAN_POINT('',(-14.5,13.,12.5));
#16611=CARTESIAN_POINT('',(-14.5,-38.525,-5.));
#16612=CARTESIAN_POINT('',(-14.5,-38.525,-20.5));
#16613=CARTESIAN_POINT('',(-14.5,-39.25,-5.));
#16614=CARTESIAN_POINT('',(-14.5,0.,-5.));
#16615=CARTESIAN_POINT('',(-14.5,-39.25,-14.5));
#16616=CARTESIAN_POINT('',(-14.5,-39.25,-20.5));
#16617=CARTESIAN_POINT('',(-14.5,-47.8957988313507,-14.5));
#16618=CARTESIAN_POINT('',(-14.5,13.,-14.5));
#16619=CARTESIAN_POINT('',(-14.5,-48.1,-14.5));
#16620=CARTESIAN_POINT('',(-14.5,13.,-14.5));
#16621=CARTESIAN_POINT('',(-14.5,-48.1,-12.5));
#16622=CARTESIAN_POINT('',(-14.5,-48.1,-20.5));
#16623=CARTESIAN_POINT('',(-14.5,-40.5,-12.5));
#16624=CARTESIAN_POINT('',(-14.5,13.,-12.5));
#16625=CARTESIAN_POINT('',(-14.5,-40.5,-20.5));
#16626=CARTESIAN_POINT('Origin',(0.,0.,-14.5));
#16627=CARTESIAN_POINT('',(-18.4170000000001,7.97500000000004,-14.5));
#16628=CARTESIAN_POINT('',(-15.59525837089,12.12462004281,-14.5));
#16629=CARTESIAN_POINT('',(0.,7.975,-14.5));
#16630=CARTESIAN_POINT('Origin',(-15.,13.,-14.5));
#16631=CARTESIAN_POINT('',(-19.5807795062061,6.26355954969803,-14.5));
#16632=CARTESIAN_POINT('',(-19.437,6.475,-14.5));
#16633=CARTESIAN_POINT('',(-19.58077950621,6.263559549693,-14.5));
#16634=CARTESIAN_POINT('',(-19.4370000000001,6.47500000000004,-12.5));
#16635=CARTESIAN_POINT('',(-19.4370000000002,6.47500000000015,-14.5));
#16636=CARTESIAN_POINT('',(-18.4170000000002,7.97500000000007,-12.5));
#16637=CARTESIAN_POINT('',(-15.,13.,-12.5));
#16638=CARTESIAN_POINT('',(-18.4170000000002,7.97500000000011,-14.5));
#16639=CARTESIAN_POINT('',(-19.5807795062094,6.26355954969258,-14.5));
#16640=CARTESIAN_POINT('Origin',(17.1,4.576629485471,-12.38062237617));
#16641=CARTESIAN_POINT('',(19.5807795062088,6.26355954969267,-14.5));
#16642=CARTESIAN_POINT('',(19.580779506209,6.26355954969229,-12.38062237617));
#16643=CARTESIAN_POINT('',(20.1,4.576629485471,-14.5));
#16644=CARTESIAN_POINT('Origin',(17.1,4.576629485471,-14.5));
#16645=CARTESIAN_POINT('',(20.1,4.576629485471,-12.38062237617));
#16646=CARTESIAN_POINT('Origin',(20.1,-40.6,-14.5));
#16647=CARTESIAN_POINT('',(20.1,1.525,-14.5));
#16648=CARTESIAN_POINT('',(20.1,-40.6,-14.5));
#16649=CARTESIAN_POINT('',(20.1,1.525,-12.5));
#16650=CARTESIAN_POINT('',(20.1,1.525,-14.5));
#16651=CARTESIAN_POINT('',(20.1,0.0249999999999991,-12.5));
#16652=CARTESIAN_POINT('',(20.1,0.,-12.5));
#16653=CARTESIAN_POINT('',(20.1,0.025,-14.5));
#16654=CARTESIAN_POINT('',(20.1,0.0249999999999972,-14.5));
#16655=CARTESIAN_POINT('',(20.1,-14.025,-14.5));
#16656=CARTESIAN_POINT('',(20.1,-40.6,-14.5));
#16657=CARTESIAN_POINT('',(20.1,-14.025,-12.5));
#16658=CARTESIAN_POINT('',(20.1,-14.025,-14.5));
#16659=CARTESIAN_POINT('',(20.1,-15.525,-12.5));
#16660=CARTESIAN_POINT('',(20.1,0.,-12.5));
#16661=CARTESIAN_POINT('',(20.1,-15.525,-14.5));
#16662=CARTESIAN_POINT('',(20.1,-15.525,-14.5));
#16663=CARTESIAN_POINT('',(20.1,-20.475,-14.5));
#16664=CARTESIAN_POINT('',(20.1,-40.6,-14.5));
#16665=CARTESIAN_POINT('',(20.1,-20.475,-12.5));
#16666=CARTESIAN_POINT('',(20.1,-20.475,-14.5));
#16667=CARTESIAN_POINT('',(20.1,-21.975,-12.5));
#16668=CARTESIAN_POINT('',(20.1,0.,-12.5));
#16669=CARTESIAN_POINT('',(20.1,-21.975,-14.5));
#16670=CARTESIAN_POINT('',(20.1,-21.975,-14.5));
#16671=CARTESIAN_POINT('',(20.1,-39.67662948547,-14.5));
#16672=CARTESIAN_POINT('',(20.1,-40.6,-14.5));
#16673=CARTESIAN_POINT('',(20.1,-39.67662948547,-14.5));
#16674=CARTESIAN_POINT('Origin',(17.1,-39.67662948547,-14.38062237617));
#16675=CARTESIAN_POINT('',(19.5807795062097,-41.3635595496912,-14.5));
#16676=CARTESIAN_POINT('Origin',(17.1,-39.67662948547,-14.5));
#16677=CARTESIAN_POINT('',(19.5807795062099,-41.3635595496899,-14.38062237617));
#16678=CARTESIAN_POINT('Origin',(15.,-48.1,-14.5));
#16679=CARTESIAN_POINT('',(15.8928875563296,-46.7869300642212,-14.5));
#16680=CARTESIAN_POINT('',(15.,-48.1,-14.5));
#16681=CARTESIAN_POINT('',(15.8928875563303,-46.7869300642202,-14.5));
#16682=CARTESIAN_POINT('Origin',(13.41210805012,-45.1,-14.36535464022));
#16683=CARTESIAN_POINT('',(14.5,-47.8957988313507,-14.5));
#16684=CARTESIAN_POINT('',(13.4749927141525,-48.0996705000861,-14.5));
#16685=CARTESIAN_POINT('Origin',(13.41210805012,-45.1,-14.5));
#16686=CARTESIAN_POINT('',(13.41210805012,-48.1,-14.5));
#16687=CARTESIAN_POINT('Origin',(13.41210805012,-45.1,-14.5));
#16688=CARTESIAN_POINT('',(13.41210805012,-48.1,-14.36535464022));
#16689=CARTESIAN_POINT('Origin',(13.41210805012,-45.1,-14.5));
#16690=CARTESIAN_POINT('Origin',(-15.,-48.1,-14.5));
#16691=CARTESIAN_POINT('',(8.525,-48.1,-14.5));
#16692=CARTESIAN_POINT('',(-15.,-48.1,-14.5));
#16693=CARTESIAN_POINT('',(8.525,-48.1,-12.5));
#16694=CARTESIAN_POINT('',(8.525,-48.1,-14.5));
#16695=CARTESIAN_POINT('',(7.025,-48.1,-12.5));
#16696=CARTESIAN_POINT('',(0.,-48.1,-12.5));
#16697=CARTESIAN_POINT('',(7.025,-48.1,-14.5));
#16698=CARTESIAN_POINT('',(7.025,-48.1,-14.5));
#16699=CARTESIAN_POINT('',(-7.025,-48.1,-14.5));
#16700=CARTESIAN_POINT('',(-15.,-48.1,-14.5));
#16701=CARTESIAN_POINT('',(-7.025,-48.1,-12.5));
#16702=CARTESIAN_POINT('',(-7.025,-48.1,-14.5));
#16703=CARTESIAN_POINT('',(-8.525,-48.1,-12.5));
#16704=CARTESIAN_POINT('',(0.,-48.1,-12.5));
#16705=CARTESIAN_POINT('',(-8.525,-48.1,-14.5));
#16706=CARTESIAN_POINT('',(-8.525,-48.1,-14.5));
#16707=CARTESIAN_POINT('',(-13.41210805012,-48.1,-14.5));
#16708=CARTESIAN_POINT('',(-15.,-48.1,-14.5));
#16709=CARTESIAN_POINT('',(-13.41210805012,-48.1,-14.5));
#16710=CARTESIAN_POINT('Origin',(-13.41210805012,-45.1,-14.38062237617));
#16711=CARTESIAN_POINT('',(-13.4749927055872,-48.0996705002657,-14.5));
#16712=CARTESIAN_POINT('Origin',(-13.41210805012,-45.1,-14.5));
#16713=CARTESIAN_POINT('',(-15.8928875563293,-46.786930064221,-14.5));
#16714=CARTESIAN_POINT('Origin',(-13.41210805012,-45.1,-14.5));
#16715=CARTESIAN_POINT('',(-15.8928875563299,-46.7869300642199,-14.38062237617));
#16716=CARTESIAN_POINT('Origin',(-13.41210805012,-45.1,-14.5));
#16717=CARTESIAN_POINT('Origin',(-20.1,-40.6,-14.5));
#16718=CARTESIAN_POINT('',(-19.5807795062098,-41.3635595496914,-14.5));
#16719=CARTESIAN_POINT('',(-20.1,-40.6,-14.5));
#16720=CARTESIAN_POINT('',(-19.5807795062105,-41.3635595496904,-14.5));
#16721=CARTESIAN_POINT('Origin',(-17.1,-39.67662948547,-14.36535464022));
#16722=CARTESIAN_POINT('',(-20.1,-39.67662948547,-14.5));
#16723=CARTESIAN_POINT('Origin',(-17.1,-39.67662948547,-14.5));
#16724=CARTESIAN_POINT('',(-20.1,-39.67662948547,-14.36535464022));
#16725=CARTESIAN_POINT('Origin',(-20.1,5.5,-14.5));
#16726=CARTESIAN_POINT('',(-20.1,-21.975,-14.5));
#16727=CARTESIAN_POINT('',(-20.1,5.5,-14.5));
#16728=CARTESIAN_POINT('',(-20.1,-21.975,-12.5));
#16729=CARTESIAN_POINT('',(-20.1,-21.975,-14.5));
#16730=CARTESIAN_POINT('',(-20.1,-20.475,-12.5));
#16731=CARTESIAN_POINT('',(-20.1,5.5,-12.5));
#16732=CARTESIAN_POINT('',(-20.1,-20.475,-14.5));
#16733=CARTESIAN_POINT('',(-20.1,-20.475,-14.5));
#16734=CARTESIAN_POINT('',(-20.1,-15.525,-14.5));
#16735=CARTESIAN_POINT('',(-20.1,5.5,-14.5));
#16736=CARTESIAN_POINT('',(-20.1,-15.525,-12.5));
#16737=CARTESIAN_POINT('',(-20.1,-15.525,-14.5));
#16738=CARTESIAN_POINT('',(-20.1,-14.025,-12.5));
#16739=CARTESIAN_POINT('',(-20.1,5.5,-12.5));
#16740=CARTESIAN_POINT('',(-20.1,-14.025,-14.5));
#16741=CARTESIAN_POINT('',(-20.1,-14.025,-14.5));
#16742=CARTESIAN_POINT('',(-20.1,0.0249999999999999,-14.5));
#16743=CARTESIAN_POINT('',(-20.1,5.5,-14.5));
#16744=CARTESIAN_POINT('',(-20.1,0.0249999999999999,-12.5));
#16745=CARTESIAN_POINT('',(-20.1,0.0249999999999998,-14.5));
#16746=CARTESIAN_POINT('',(-20.1,1.525,-12.5));
#16747=CARTESIAN_POINT('',(-20.1,5.5,-12.5));
#16748=CARTESIAN_POINT('',(-20.1,1.525,-14.5));
#16749=CARTESIAN_POINT('',(-20.1,1.525,-14.5));
#16750=CARTESIAN_POINT('',(-20.1,4.576629485471,-14.5));
#16751=CARTESIAN_POINT('',(-20.1,5.5,-14.5));
#16752=CARTESIAN_POINT('',(-20.1,4.576629485471,-14.5));
#16753=CARTESIAN_POINT('Origin',(-17.1,4.576629485471,-12.38062237617));
#16754=CARTESIAN_POINT('Origin',(-17.1,4.576629485471,-14.5));
#16755=CARTESIAN_POINT('Origin',(-6.64999999999998,9.49999999999996,-17.));
#16756=CARTESIAN_POINT('',(-8.15,9.5,-19.));
#16757=CARTESIAN_POINT('Origin',(-6.65,9.5,-19.));
#16758=CARTESIAN_POINT('Origin',(-8.15,9.49999999999999,-17.));
#16759=CARTESIAN_POINT('Origin',(-8.15,13.,-20.5));
#16760=CARTESIAN_POINT('',(-8.15,9.00000000030975,-19.));
#16761=CARTESIAN_POINT('',(-8.15,13.,-19.));
#16762=CARTESIAN_POINT('',(-8.15,9.,-20.5));
#16763=CARTESIAN_POINT('Origin',(-10.5,9.,-20.5));
#16764=CARTESIAN_POINT('',(-10.5,6.65,-19.));
#16765=CARTESIAN_POINT('',(-10.5,6.65,-20.5));
#16766=CARTESIAN_POINT('Origin',(-10.5,9.,-19.));
#16767=CARTESIAN_POINT('Origin',(-10.5,6.65,-20.5));
#16768=CARTESIAN_POINT('',(-13.5,6.6500000000001,-18.4999999994861));
#16769=CARTESIAN_POINT('',(-13.,6.65000000000009,-18.9999999999985));
#16770=CARTESIAN_POINT('Ctrl Pts',(-13.5,6.65000000000025,-18.4999999994861));
#16771=CARTESIAN_POINT('Ctrl Pts',(-13.5000000003688,6.65000000000034,-18.7411872045822));
#16772=CARTESIAN_POINT('Ctrl Pts',(-13.2411750364478,6.65000000000035,-18.9975772517629));
#16773=CARTESIAN_POINT('Ctrl Pts',(-13.,6.65000000000028,-18.9999999999985));
#16774=CARTESIAN_POINT('',(-13.5,6.65,-20.5));
#16775=CARTESIAN_POINT('',(-10.5,6.65,-19.));
#16776=CARTESIAN_POINT('Origin',(-13.5,5.65,-16.88062237617));
#16777=CARTESIAN_POINT('',(-14.4999999999994,5.65,-18.4999999994854));
#16778=CARTESIAN_POINT('Origin',(-13.5000000000004,5.65000000000104,-18.5000000058401));
#16779=CARTESIAN_POINT('',(-14.5,5.65,-16.88062237617));
#16780=CARTESIAN_POINT('Origin',(-14.5,13.,-20.5));
#16781=CARTESIAN_POINT('',(-14.5000000000002,5.14999999999998,-18.9999999999996));
#16782=CARTESIAN_POINT('Ctrl Pts',(-14.5000000000005,5.14999999999998,-18.9999999999996));
#16783=CARTESIAN_POINT('Ctrl Pts',(-14.5000000000009,5.39101397566289,-18.9908604458716));
#16784=CARTESIAN_POINT('Ctrl Pts',(-14.4999999999995,5.65000000036765,-18.7411872045961));
#16785=CARTESIAN_POINT('Ctrl Pts',(-14.4999999999986,5.65,-18.4999999994854));
#16786=CARTESIAN_POINT('',(-14.5000000000004,-34.65,-18.9999999999984));
#16787=CARTESIAN_POINT('',(-14.5,13.,-19.));
#16788=CARTESIAN_POINT('',(-14.5000000000008,-35.15,-18.4999999994855));
#16789=CARTESIAN_POINT('Ctrl Pts',(-14.5000000000019,-35.15,-18.4999999994855));
#16790=CARTESIAN_POINT('Ctrl Pts',(-14.5000000000027,-35.1500000003693,
-18.7411872045814));
#16791=CARTESIAN_POINT('Ctrl Pts',(-14.5000000000008,-34.891175036448,-18.9975772517615));
#16792=CARTESIAN_POINT('Ctrl Pts',(-14.5000000000013,-34.65,-18.9999999999984));
#16793=CARTESIAN_POINT('',(-14.5,-35.15,-20.5));
#16794=CARTESIAN_POINT('Origin',(-13.5,-35.15,-20.63464535978));
#16795=CARTESIAN_POINT('',(-13.4999999999999,-36.1499999999995,-18.4999999994848));
#16796=CARTESIAN_POINT('Origin',(-13.4999999999957,-35.1499999999943,-18.500000005847));
#16797=CARTESIAN_POINT('',(-13.5,-36.15,-20.63464535978));
#16798=CARTESIAN_POINT('Origin',(-14.5,-36.15,-20.5));
#16799=CARTESIAN_POINT('',(-10.5,-36.15,-19.));
#16800=CARTESIAN_POINT('',(-10.5,-36.15,-20.5));
#16801=CARTESIAN_POINT('',(-13.,-36.1500000000002,-19.));
#16802=CARTESIAN_POINT('Ctrl Pts',(-13.,-36.1500000000006,-19.));
#16803=CARTESIAN_POINT('Ctrl Pts',(-13.2410139756646,-36.1500000000009,
-18.9908604458711));
#16804=CARTESIAN_POINT('Ctrl Pts',(-13.5000000003674,-36.1499999999995,
-18.7411872045957));
#16805=CARTESIAN_POINT('Ctrl Pts',(-13.4999999999999,-36.1499999999986,
-18.4999999994848));
#16806=CARTESIAN_POINT('',(-14.5,-36.15,-19.));
#16807=CARTESIAN_POINT('Origin',(-10.5,-38.5,-20.5));
#16808=CARTESIAN_POINT('',(-8.15,-38.5000000003124,-19.));
#16809=CARTESIAN_POINT('',(-8.15,-38.5,-20.5));
#16810=CARTESIAN_POINT('Origin',(-10.5,-38.5,-19.));
#16811=CARTESIAN_POINT('Origin',(-8.15,-38.5,-20.5));
#16812=CARTESIAN_POINT('',(-8.1500000000001,-41.5,-18.4999999994855));
#16813=CARTESIAN_POINT('',(-8.14999999999996,-41.,-18.9999999999984));
#16814=CARTESIAN_POINT('Ctrl Pts',(-8.15000000000025,-41.5,-18.4999999994855));
#16815=CARTESIAN_POINT('Ctrl Pts',(-8.15000000000033,-41.5000000003692,
-18.7411872045814));
#16816=CARTESIAN_POINT('Ctrl Pts',(-8.1500000000003,-41.241175036448,-18.9975772517615));
#16817=CARTESIAN_POINT('Ctrl Pts',(-8.14999999999988,-41.,-18.9999999999984));
#16818=CARTESIAN_POINT('',(-8.15,-41.5,-20.5));
#16819=CARTESIAN_POINT('',(-8.15,-38.5,-19.));
#16820=CARTESIAN_POINT('Origin',(-7.15,-41.5,-16.88062237617));
#16821=CARTESIAN_POINT('',(-7.15,-42.4999999999995,-18.4999999994848));
#16822=CARTESIAN_POINT('Origin',(-7.15000000000103,-41.5000000000004,-18.500000005847));
#16823=CARTESIAN_POINT('',(-7.15,-42.5,-16.88062237617));
#16824=CARTESIAN_POINT('Origin',(-14.5,-42.5,-20.5));
#16825=CARTESIAN_POINT('',(-6.64999999999998,-42.5000000000002,-18.9999999999996));
#16826=CARTESIAN_POINT('Ctrl Pts',(-6.64999999999998,-42.5000000000005,
-18.9999999999996));
#16827=CARTESIAN_POINT('Ctrl Pts',(-6.89101397566309,-42.5000000000009,
-18.9908604458716));
#16828=CARTESIAN_POINT('Ctrl Pts',(-7.15000000036808,-42.4999999999995,
-18.7411872045957));
#16829=CARTESIAN_POINT('Ctrl Pts',(-7.15,-42.4999999999986,-18.4999999994848));
#16830=CARTESIAN_POINT('',(6.65,-42.5000000000004,-19.));
#16831=CARTESIAN_POINT('',(-14.5,-42.5,-19.));
#16832=CARTESIAN_POINT('',(7.15,-42.5000000000008,-18.4999999994861));
#16833=CARTESIAN_POINT('Ctrl Pts',(7.15,-42.5000000000019,-18.4999999994861));
#16834=CARTESIAN_POINT('Ctrl Pts',(7.15000000036776,-42.5000000000027,-18.7411872045842));
#16835=CARTESIAN_POINT('Ctrl Pts',(6.89117503644782,-42.5000000000008,-18.997577251766));
#16836=CARTESIAN_POINT('Ctrl Pts',(6.65,-42.5000000000013,-19.));
#16837=CARTESIAN_POINT('',(7.15,-42.5,-20.5));
#16838=CARTESIAN_POINT('Origin',(7.15,-41.5,-20.63464535978));
#16839=CARTESIAN_POINT('',(8.15000000000002,-41.4999999999999,-18.4999999994854));
#16840=CARTESIAN_POINT('Origin',(7.149999999994,-41.4999999999948,-18.5000000058402));
#16841=CARTESIAN_POINT('',(8.15,-41.5,-20.63464535978));
#16842=CARTESIAN_POINT('Origin',(8.15,-42.5,-20.5));
#16843=CARTESIAN_POINT('',(8.15,-38.5,-19.));
#16844=CARTESIAN_POINT('',(8.15,-38.5,-20.5));
#16845=CARTESIAN_POINT('',(8.15,-41.,-19.));
#16846=CARTESIAN_POINT('Ctrl Pts',(8.14999999999999,-41.,-19.));
#16847=CARTESIAN_POINT('Ctrl Pts',(8.15000000000028,-41.2410139756644,-18.9908604458711));
#16848=CARTESIAN_POINT('Ctrl Pts',(8.15000000000017,-41.5000000003669,-18.7411872045961));
#16849=CARTESIAN_POINT('Ctrl Pts',(8.15000000000004,-41.5,-18.4999999994854));
#16850=CARTESIAN_POINT('',(8.15,-42.5,-19.));
#16851=CARTESIAN_POINT('Origin',(10.5,-38.5,-20.5));
#16852=CARTESIAN_POINT('',(10.5000000003124,-36.15,-19.));
#16853=CARTESIAN_POINT('',(10.5,-36.15,-20.5));
#16854=CARTESIAN_POINT('Origin',(10.5,-38.5,-19.));
#16855=CARTESIAN_POINT('Origin',(10.5,-36.15,-20.5));
#16856=CARTESIAN_POINT('',(13.5,-36.1500000000008,-18.4999999994861));
#16857=CARTESIAN_POINT('',(13.,-36.1500000000004,-18.9999999999985));
#16858=CARTESIAN_POINT('Ctrl Pts',(13.5,-36.1500000000019,-18.4999999994861));
#16859=CARTESIAN_POINT('Ctrl Pts',(13.5000000003688,-36.1500000000027,-18.7411872045822));
#16860=CARTESIAN_POINT('Ctrl Pts',(13.2411750364478,-36.1500000000008,-18.9975772517629));
#16861=CARTESIAN_POINT('Ctrl Pts',(13.,-36.1500000000013,-18.9999999999985));
#16862=CARTESIAN_POINT('',(13.5,-36.15,-20.5));
#16863=CARTESIAN_POINT('',(10.5,-36.15,-19.));
#16864=CARTESIAN_POINT('Origin',(13.5,-35.15,-16.88062237617));
#16865=CARTESIAN_POINT('',(14.4999999999994,-35.1499999999999,-18.4999999994854));
#16866=CARTESIAN_POINT('Origin',(13.4999999999943,-35.1499999999957,-18.5000000058401));
#16867=CARTESIAN_POINT('',(14.5,-35.15,-16.88062237617));
#16868=CARTESIAN_POINT('Origin',(14.5,-42.5,-20.5));
#16869=CARTESIAN_POINT('',(14.5000000000002,-34.65,-19.));
#16870=CARTESIAN_POINT('Ctrl Pts',(14.5000000000005,-34.65,-19.));
#16871=CARTESIAN_POINT('Ctrl Pts',(14.5000000000009,-34.8910139756644,-18.9908604458711));
#16872=CARTESIAN_POINT('Ctrl Pts',(14.4999999999995,-35.1500000003669,-18.7411872045961));
#16873=CARTESIAN_POINT('Ctrl Pts',(14.4999999999986,-35.1499999999999,-18.4999999994854));
#16874=CARTESIAN_POINT('',(14.5000000000004,5.15,-18.9999999999998));
#16875=CARTESIAN_POINT('',(14.5,-42.5,-19.));
#16876=CARTESIAN_POINT('',(14.5000000000008,5.65,-18.4999999994855));
#16877=CARTESIAN_POINT('Ctrl Pts',(14.5000000000019,5.65,-18.4999999994855));
#16878=CARTESIAN_POINT('Ctrl Pts',(14.5000000000027,5.65000000036822,-18.7411872045835));
#16879=CARTESIAN_POINT('Ctrl Pts',(14.5000000000008,5.39117503644798,-18.9975772517647));
#16880=CARTESIAN_POINT('Ctrl Pts',(14.5000000000013,5.15,-18.9999999999998));
#16881=CARTESIAN_POINT('',(14.5,5.65,-20.5));
#16882=CARTESIAN_POINT('Origin',(13.5,5.65,-20.63464535978));
#16883=CARTESIAN_POINT('',(13.4999999999999,6.65000000000002,-18.4999999994848));
#16884=CARTESIAN_POINT('Origin',(13.4999999999948,5.649999999994,-18.500000005847));
#16885=CARTESIAN_POINT('',(13.5,6.65,-20.63464535978));
#16886=CARTESIAN_POINT('Origin',(14.5,6.65,-20.5));
#16887=CARTESIAN_POINT('',(10.5,6.65,-19.));
#16888=CARTESIAN_POINT('',(10.5,6.65,-20.5));
#16889=CARTESIAN_POINT('',(13.,6.65,-19.));
#16890=CARTESIAN_POINT('Ctrl Pts',(13.,6.64999999999999,-19.));
#16891=CARTESIAN_POINT('Ctrl Pts',(13.2410139756646,6.65000000000028,-18.9908604458711));
#16892=CARTESIAN_POINT('Ctrl Pts',(13.5000000003674,6.65000000000017,-18.7411872045957));
#16893=CARTESIAN_POINT('Ctrl Pts',(13.4999999999999,6.65000000000004,-18.4999999994848));
#16894=CARTESIAN_POINT('',(14.5,6.65,-19.));
#16895=CARTESIAN_POINT('Origin',(10.5,9.,-20.5));
#16896=CARTESIAN_POINT('',(8.15,9.000000000459,-19.));
#16897=CARTESIAN_POINT('',(8.15,9.000000000918,-20.5));
#16898=CARTESIAN_POINT('Origin',(10.5,9.,-19.));
#16899=CARTESIAN_POINT('Origin',(8.15,9.,-20.5));
#16900=CARTESIAN_POINT('',(8.15,9.5,-19.));
#16901=CARTESIAN_POINT('',(8.15,9.639713176691,-19.));
#16902=CARTESIAN_POINT('Origin',(8.15,9.49999999999999,-17.));
#16903=CARTESIAN_POINT('Origin',(6.65,9.50000000000007,-17.0000000000001));
#16904=CARTESIAN_POINT('Origin',(6.65,9.5,-19.));
#16905=CARTESIAN_POINT('Origin',(20.1,5.5,-14.5));
#16906=CARTESIAN_POINT('',(18.4169999999999,7.97499999999996,-14.5));
#16907=CARTESIAN_POINT('',(20.1,5.5,-14.5));
#16908=CARTESIAN_POINT('',(18.4169999999999,7.97499999999996,-12.5));
#16909=CARTESIAN_POINT('',(18.4169999999999,7.97499999999994,-14.5));
#16910=CARTESIAN_POINT('',(19.437,6.47499999999999,-12.5));
#16911=CARTESIAN_POINT('',(20.1,5.5,-12.5));
#16912=CARTESIAN_POINT('',(19.437,6.47499999999999,-14.5));
#16913=CARTESIAN_POINT('',(19.437,6.47499999999998,-14.5));
#16914=CARTESIAN_POINT('',(20.1,5.5,-14.5));
#16915=CARTESIAN_POINT('Origin',(0.,0.,-20.5));
#16916=CARTESIAN_POINT('',(10.5000000000002,5.1500005893432,-20.4999999999999));
#16917=CARTESIAN_POINT('',(6.65000039306064,9.00000000001898,-20.4999999999998));
#16918=CARTESIAN_POINT('Origin',(10.5000016830354,9.0000020756571,-20.5000000000012));
#16919=CARTESIAN_POINT('',(13.,5.15,-20.5));
#16920=CARTESIAN_POINT('',(0.,5.15,-20.5));
#16921=CARTESIAN_POINT('',(13.,-34.65000000018,-20.5));
#16922=CARTESIAN_POINT('',(13.,0.,-20.5));
#16923=CARTESIAN_POINT('',(10.5000000005402,-34.6500004912993,-20.4999999999998));
#16924=CARTESIAN_POINT('',(0.,-34.65000000024,-20.5));
#16925=CARTESIAN_POINT('',(6.6500005893432,-38.5000000000002,-20.4999999999999));
#16926=CARTESIAN_POINT('Origin',(10.5000017894248,-38.5000015931868,-20.500000000001));
#16927=CARTESIAN_POINT('',(6.65,-41.,-20.5));
#16928=CARTESIAN_POINT('',(6.65,0.,-20.5));
#16929=CARTESIAN_POINT('',(-6.650000000177,-41.,-20.5));
#16930=CARTESIAN_POINT('',(0.,-41.,-20.5));
#16931=CARTESIAN_POINT('',(-6.65000049129643,-38.5000000005401,-20.4999999999998));
#16932=CARTESIAN_POINT('',(-6.650000000236,0.,-20.5));
#16933=CARTESIAN_POINT('',(-10.4999999999999,-34.6500012274245,-20.4999999999997));
#16934=CARTESIAN_POINT('Origin',(-10.4999997334424,-38.5000012060096,-20.5000000000009));
#16935=CARTESIAN_POINT('',(-13.,-34.65,-20.5));
#16936=CARTESIAN_POINT('',(0.,-34.65,-20.5));
#16937=CARTESIAN_POINT('',(-13.,5.1500019635795,-20.5));
#16938=CARTESIAN_POINT('',(-13.,0.,-20.5));
#16939=CARTESIAN_POINT('',(-10.5000000000006,5.15000274884423,-20.4999999999992));
#16940=CARTESIAN_POINT('',(0.,5.150003927159,-20.5));
#16941=CARTESIAN_POINT('',(-6.65000000007813,9.00000000072159,-20.5));
#16942=CARTESIAN_POINT('Origin',(-10.499997711063,8.99999928187284,-20.5));
#16943=CARTESIAN_POINT('',(-6.65,0.,-20.5));
#16944=CARTESIAN_POINT('',(6.650000000236,0.,-20.5));
#16945=CARTESIAN_POINT('Origin',(0.,0.,-14.5));
#16946=CARTESIAN_POINT('',(14.5,7.975,-14.5));
#16947=CARTESIAN_POINT('',(0.,7.975,-14.5));
#16948=CARTESIAN_POINT('',(14.5,0.,-14.5));
#16949=CARTESIAN_POINT('Origin',(0.,0.,14.5));
#16950=CARTESIAN_POINT('',(18.417,7.97499999999998,14.5));
#16951=CARTESIAN_POINT('',(18.417,7.975,14.5));
#16952=CARTESIAN_POINT('',(14.5,7.975,14.5));
#16953=CARTESIAN_POINT('',(0.,7.975,14.5));
#16954=CARTESIAN_POINT('',(14.5,0.,14.5));
#16955=CARTESIAN_POINT('Origin',(14.5,-42.5,-20.5));
#16956=CARTESIAN_POINT('',(14.5,-21.975,12.5));
#16957=CARTESIAN_POINT('',(14.5,-21.975,14.5));
#16958=CARTESIAN_POINT('',(14.5,-21.975,-20.5));
#16959=CARTESIAN_POINT('',(14.5,-47.8957988313507,14.5));
#16960=CARTESIAN_POINT('',(14.5,-42.5,14.5));
#16961=CARTESIAN_POINT('',(14.5,-48.1,14.5));
#16962=CARTESIAN_POINT('',(14.5,-42.5,14.5));
#16963=CARTESIAN_POINT('',(14.5,-48.1,12.5));
#16964=CARTESIAN_POINT('',(14.5,-48.1,-20.5));
#16965=CARTESIAN_POINT('',(14.5,-40.5,12.5));
#16966=CARTESIAN_POINT('',(14.5,-42.5,12.5));
#16967=CARTESIAN_POINT('',(14.5,-40.5,-12.5));
#16968=CARTESIAN_POINT('',(14.5,-40.5,-20.5));
#16969=CARTESIAN_POINT('',(14.5,-48.1,-12.5));
#16970=CARTESIAN_POINT('',(14.5,-42.5,-12.5));
#16971=CARTESIAN_POINT('',(14.5,-48.1,-14.5));
#16972=CARTESIAN_POINT('',(14.5,-48.1,-20.5));
#16973=CARTESIAN_POINT('',(14.5,-42.5,-14.5));
#16974=CARTESIAN_POINT('',(14.5,-39.25,-14.5));
#16975=CARTESIAN_POINT('',(14.5,-42.5,-14.5));
#16976=CARTESIAN_POINT('',(14.5,-39.25,-5.));
#16977=CARTESIAN_POINT('',(14.5,-39.25,-20.5));
#16978=CARTESIAN_POINT('',(14.5,-38.525,-5.));
#16979=CARTESIAN_POINT('',(14.5,0.,-5.));
#16980=CARTESIAN_POINT('',(14.5,-38.525,12.5));
#16981=CARTESIAN_POINT('',(14.5,-38.525,-20.5));
#16982=CARTESIAN_POINT('',(14.5,-22.475,12.5));
#16983=CARTESIAN_POINT('',(14.5,-42.5,12.5));
#16984=CARTESIAN_POINT('',(14.5,-22.475,-5.));
#16985=CARTESIAN_POINT('',(14.5,-22.475,-20.5));
#16986=CARTESIAN_POINT('',(14.5,-21.75,-5.));
#16987=CARTESIAN_POINT('',(14.5,0.,-5.));
#16988=CARTESIAN_POINT('',(14.5,-21.75,-12.5));
#16989=CARTESIAN_POINT('',(14.5,-21.75,-20.5));
#16990=CARTESIAN_POINT('',(14.5,-18.10025773881,-12.5));
#16991=CARTESIAN_POINT('',(14.5,-42.5,-12.5));
#16992=CARTESIAN_POINT('',(14.5,-17.89974226119,-12.5));
#16993=CARTESIAN_POINT('',(14.5,-42.5,-12.5));
#16994=CARTESIAN_POINT('',(14.5,-14.025,-12.5));
#16995=CARTESIAN_POINT('',(14.5,-42.5,-12.5));
#16996=CARTESIAN_POINT('',(14.5,-14.025,-14.5));
#16997=CARTESIAN_POINT('',(14.5,-14.025,-20.5));
#16998=CARTESIAN_POINT('',(14.5,0.0249999999999982,-14.5));
#16999=CARTESIAN_POINT('',(14.5,-42.5,-14.5));
#17000=CARTESIAN_POINT('',(14.5,0.0249999999999982,-12.5));
#17001=CARTESIAN_POINT('',(14.5,0.0249999999999972,-20.5));
#17002=CARTESIAN_POINT('',(14.5,3.899742261193,-12.5));
#17003=CARTESIAN_POINT('',(14.5,-42.5,-12.5));
#17004=CARTESIAN_POINT('',(14.5,4.100257738807,-12.5));
#17005=CARTESIAN_POINT('',(14.5,-42.5,-12.5));
#17006=CARTESIAN_POINT('',(14.5,7.975,-12.5));
#17007=CARTESIAN_POINT('',(14.5,-42.5,-12.5));
#17008=CARTESIAN_POINT('',(14.5,7.975,-20.5));
#17009=CARTESIAN_POINT('',(14.5,7.975,12.5));
#17010=CARTESIAN_POINT('',(14.5,7.975,-20.5));
#17011=CARTESIAN_POINT('',(14.4999999999997,4.10025773880716,12.5));
#17012=CARTESIAN_POINT('',(14.5,-42.5,12.5));
#17013=CARTESIAN_POINT('',(14.5,3.899742261193,12.5));
#17014=CARTESIAN_POINT('',(14.5,-42.5,12.5));
#17015=CARTESIAN_POINT('',(14.5,0.0249999999999982,12.5));
#17016=CARTESIAN_POINT('',(14.5,-42.5,12.5));
#17017=CARTESIAN_POINT('',(14.5,0.0249999999999982,14.5));
#17018=CARTESIAN_POINT('',(14.5,0.0249999999999972,-20.5));
#17019=CARTESIAN_POINT('',(14.5,-14.025,14.5));
#17020=CARTESIAN_POINT('',(14.5,-42.5,14.5));
#17021=CARTESIAN_POINT('',(14.5,-14.025,12.5));
#17022=CARTESIAN_POINT('',(14.5,-14.025,-20.5));
#17023=CARTESIAN_POINT('',(14.5000000000001,-17.89974226119,12.5));
#17024=CARTESIAN_POINT('',(14.5,-42.5,12.5));
#17025=CARTESIAN_POINT('',(14.5,-18.10025773881,12.5));
#17026=CARTESIAN_POINT('',(14.5,-42.5,12.5));
#17027=CARTESIAN_POINT('',(14.5,-42.5,12.5));
#17028=CARTESIAN_POINT('Origin',(20.1,5.5,14.5));
#17029=CARTESIAN_POINT('',(19.580779506206,6.26355954969795,14.5));
#17030=CARTESIAN_POINT('',(19.5807795062091,6.26355954969241,14.5));
#17031=CARTESIAN_POINT('',(19.437,6.47499999999999,14.5));
#17032=CARTESIAN_POINT('',(19.437,6.475,14.5));
#17033=CARTESIAN_POINT('',(19.437,6.47499999999999,12.5));
#17034=CARTESIAN_POINT('',(19.437,6.47499999999998,14.5));
#17035=CARTESIAN_POINT('',(18.417,7.97499999999996,12.5));
#17036=CARTESIAN_POINT('',(20.1,5.5,12.5));
#17037=CARTESIAN_POINT('',(18.4169999999999,7.97499999999994,14.5));
#17038=CARTESIAN_POINT('Origin',(20.1,-40.6,14.5));
#17039=CARTESIAN_POINT('',(20.1,1.525,12.5));
#17040=CARTESIAN_POINT('',(20.1,1.525,14.5));
#17041=CARTESIAN_POINT('',(20.1,1.525,14.5));
#17042=CARTESIAN_POINT('',(20.1,4.576629485471,14.5));
#17043=CARTESIAN_POINT('',(20.1,-40.6,14.5));
#17044=CARTESIAN_POINT('',(20.1,4.576629485471,14.5));
#17045=CARTESIAN_POINT('',(20.1,-39.67662948547,14.5));
#17046=CARTESIAN_POINT('',(20.1,-39.67662948547,14.5));
#17047=CARTESIAN_POINT('',(20.1,-21.975,14.5));
#17048=CARTESIAN_POINT('',(20.1,-40.6,14.5));
#17049=CARTESIAN_POINT('',(20.1,-21.975,12.5));
#17050=CARTESIAN_POINT('',(20.1,-21.975,14.5));
#17051=CARTESIAN_POINT('',(20.1,-20.475,12.5));
#17052=CARTESIAN_POINT('',(20.1,-40.6,12.5));
#17053=CARTESIAN_POINT('',(20.1,-20.475,14.5));
#17054=CARTESIAN_POINT('',(20.1,-20.475,14.5));
#17055=CARTESIAN_POINT('',(20.1,-15.525,14.5));
#17056=CARTESIAN_POINT('',(20.1,-40.6,14.5));
#17057=CARTESIAN_POINT('',(20.1,-15.525,12.5));
#17058=CARTESIAN_POINT('',(20.1,-15.525,14.5));
#17059=CARTESIAN_POINT('',(20.1,-14.025,12.5));
#17060=CARTESIAN_POINT('',(20.1,-40.6,12.5));
#17061=CARTESIAN_POINT('',(20.1,-14.025,14.5));
#17062=CARTESIAN_POINT('',(20.1,-14.025,14.5));
#17063=CARTESIAN_POINT('',(20.1,0.0249999999999982,14.5));
#17064=CARTESIAN_POINT('',(20.1,-40.6,14.5));
#17065=CARTESIAN_POINT('',(20.1,0.0249999999999982,12.5));
#17066=CARTESIAN_POINT('',(20.1,0.0249999999999972,14.5));
#17067=CARTESIAN_POINT('',(20.1,-40.6,12.5));
#17068=CARTESIAN_POINT('Origin',(17.1,-39.67662948547,17.13971317669));
#17069=CARTESIAN_POINT('',(19.5807795062097,-41.3635595496912,14.5));
#17070=CARTESIAN_POINT('',(19.5807795062099,-41.3635595496899,17.13971317669));
#17071=CARTESIAN_POINT('Origin',(17.1,-39.67662948547,14.5));
#17072=CARTESIAN_POINT('Origin',(15.,-48.1,14.5));
#17073=CARTESIAN_POINT('',(15.8928875563296,-46.7869300642212,14.5));
#17074=CARTESIAN_POINT('',(15.8928875563303,-46.7869300642202,14.5));
#17075=CARTESIAN_POINT('',(15.,-48.1,14.5));
#17076=CARTESIAN_POINT('Origin',(13.41210805012,-45.1,17.13971317669));
#17077=CARTESIAN_POINT('',(13.41210805012,-48.1,14.5));
#17078=CARTESIAN_POINT('',(13.41210805012,-48.1,17.13971317669));
#17079=CARTESIAN_POINT('',(13.4749927054462,-48.0996705002687,14.5));
#17080=CARTESIAN_POINT('Origin',(13.41210805012,-45.1,14.5));
#17081=CARTESIAN_POINT('Origin',(13.41210805012,-45.1,14.5));
#17082=CARTESIAN_POINT('Origin',(13.41210805012,-45.1,14.5));
#17083=CARTESIAN_POINT('Origin',(-15.,-48.1,14.5));
#17084=CARTESIAN_POINT('',(8.525,-48.1,12.5));
#17085=CARTESIAN_POINT('',(8.525,-48.1,14.5));
#17086=CARTESIAN_POINT('',(8.525,-48.1,14.5));
#17087=CARTESIAN_POINT('',(-15.,-48.1,14.5));
#17088=CARTESIAN_POINT('',(-13.41210805012,-48.1,14.5));
#17089=CARTESIAN_POINT('',(-13.41210805012,-48.1,14.5));
#17090=CARTESIAN_POINT('',(-8.525,-48.1,14.5));
#17091=CARTESIAN_POINT('',(-15.,-48.1,14.5));
#17092=CARTESIAN_POINT('',(-8.525,-48.1,12.5));
#17093=CARTESIAN_POINT('',(-8.525,-48.1,14.5));
#17094=CARTESIAN_POINT('',(-7.025,-48.1,12.5));
#17095=CARTESIAN_POINT('',(0.,-48.1,12.5));
#17096=CARTESIAN_POINT('',(-7.025,-48.1,14.5));
#17097=CARTESIAN_POINT('',(-7.025,-48.1,14.5));
#17098=CARTESIAN_POINT('',(7.025,-48.1,14.5));
#17099=CARTESIAN_POINT('',(-15.,-48.1,14.5));
#17100=CARTESIAN_POINT('',(7.025,-48.1,12.5));
#17101=CARTESIAN_POINT('',(7.025,-48.1,14.5));
#17102=CARTESIAN_POINT('',(0.,-48.1,12.5));
#17103=CARTESIAN_POINT('Origin',(-13.41210805012,-45.1,17.13971317669));
#17104=CARTESIAN_POINT('',(-15.8928875563293,-46.786930064221,14.5));
#17105=CARTESIAN_POINT('',(-15.8928875563299,-46.7869300642199,17.13971317669));
#17106=CARTESIAN_POINT('Origin',(-13.41210805012,-45.1,14.5));
#17107=CARTESIAN_POINT('',(-13.4749927055872,-48.0996705002657,14.5));
#17108=CARTESIAN_POINT('Origin',(-13.41210805012,-45.1,14.5));
#17109=CARTESIAN_POINT('Origin',(-13.41210805012,-45.1,14.5));
#17110=CARTESIAN_POINT('Origin',(-20.1,-40.6,14.5));
#17111=CARTESIAN_POINT('',(-19.5807795062098,-41.3635595496914,14.5));
#17112=CARTESIAN_POINT('',(-19.5807795062105,-41.3635595496904,14.5));
#17113=CARTESIAN_POINT('',(-20.1,-40.6,14.5));
#17114=CARTESIAN_POINT('Origin',(-17.1,-39.67662948547,17.13971317669));
#17115=CARTESIAN_POINT('',(-20.1,-39.67662948547,14.5));
#17116=CARTESIAN_POINT('',(-20.1,-39.67662948547,17.13971317669));
#17117=CARTESIAN_POINT('Origin',(-17.1,-39.67662948547,14.5));
#17118=CARTESIAN_POINT('Origin',(-20.1,5.5,14.5));
#17119=CARTESIAN_POINT('',(-20.1,-21.975,12.5));
#17120=CARTESIAN_POINT('',(-20.1,-21.975,14.5));
#17121=CARTESIAN_POINT('',(-20.1,-21.975,14.5));
#17122=CARTESIAN_POINT('',(-20.1,5.5,14.5));
#17123=CARTESIAN_POINT('',(-20.1,4.576629485471,14.5));
#17124=CARTESIAN_POINT('',(-20.1,4.576629485471,14.5));
#17125=CARTESIAN_POINT('',(-20.1,1.525,14.5));
#17126=CARTESIAN_POINT('',(-20.1,5.5,14.5));
#17127=CARTESIAN_POINT('',(-20.1,1.525,12.5));
#17128=CARTESIAN_POINT('',(-20.1,1.525,14.5));
#17129=CARTESIAN_POINT('',(-20.1,0.0249999999999999,12.5));
#17130=CARTESIAN_POINT('',(-20.1,5.5,12.5));
#17131=CARTESIAN_POINT('',(-20.1,0.0249999999999999,14.5));
#17132=CARTESIAN_POINT('',(-20.1,0.0249999999999998,14.5));
#17133=CARTESIAN_POINT('',(-20.1,-14.025,14.5));
#17134=CARTESIAN_POINT('',(-20.1,5.5,14.5));
#17135=CARTESIAN_POINT('',(-20.1,-14.025,12.5));
#17136=CARTESIAN_POINT('',(-20.1,-14.025,14.5));
#17137=CARTESIAN_POINT('',(-20.1,-15.525,12.5));
#17138=CARTESIAN_POINT('',(-20.1,5.5,12.5));
#17139=CARTESIAN_POINT('',(-20.1,-15.525,14.5));
#17140=CARTESIAN_POINT('',(-20.1,-15.525,14.5));
#17141=CARTESIAN_POINT('',(-20.1,-20.475,14.5));
#17142=CARTESIAN_POINT('',(-20.1,5.5,14.5));
#17143=CARTESIAN_POINT('',(-20.1,-20.475,12.5));
#17144=CARTESIAN_POINT('',(-20.1,-20.475,14.5));
#17145=CARTESIAN_POINT('',(-20.1,5.5,12.5));
#17146=CARTESIAN_POINT('Origin',(-17.1,4.576629485471,17.13971317669));
#17147=CARTESIAN_POINT('Origin',(-17.1,4.576629485471,14.5));
#17148=CARTESIAN_POINT('Origin',(17.1,4.576629485471,17.13971317669));
#17149=CARTESIAN_POINT('Origin',(17.1,4.576629485471,14.5));
#17150=CARTESIAN_POINT('Origin',(-20.1,6.475,12.5));
#17151=CARTESIAN_POINT('',(-15.87105808376,6.475,12.5));
#17152=CARTESIAN_POINT('',(-20.1,6.475,12.5));
#17153=CARTESIAN_POINT('',(-15.87105808376,6.475,14.5));
#17154=CARTESIAN_POINT('',(-15.87105808376,6.475,12.5));
#17155=CARTESIAN_POINT('',(-20.1,6.475,14.5));
#17156=CARTESIAN_POINT('Origin',(0.,0.,12.5));
#17157=CARTESIAN_POINT('',(0.,7.975,12.5));
#17158=CARTESIAN_POINT('',(-15.87105808376,6.475,12.5));
#17159=CARTESIAN_POINT('Origin',(-14.5,7.975,12.5));
#17160=CARTESIAN_POINT('Origin',(-15.,-48.1,14.5));
#17161=CARTESIAN_POINT('',(-13.475,-48.1,12.5));
#17162=CARTESIAN_POINT('',(-15.,-48.1,12.5));
#17163=CARTESIAN_POINT('',(-13.475,-48.1,12.5));
#17164=CARTESIAN_POINT('',(-15.,-48.1,14.5));
#17165=CARTESIAN_POINT('Origin',(0.,0.,12.5));
#17166=CARTESIAN_POINT('',(-13.475,-43.87105808376,12.5));
#17167=CARTESIAN_POINT('',(-11.1002577388094,-42.5000000000011,12.5));
#17168=CARTESIAN_POINT('',(-13.475,-43.87105808376,12.5));
#17169=CARTESIAN_POINT('',(-13.475,0.,12.5));
#17170=CARTESIAN_POINT('',(-12.5,-42.5,12.5));
#17171=CARTESIAN_POINT('Origin',(-12.5,-40.5,12.5));
#17172=CARTESIAN_POINT('',(-14.5,-42.5,12.5));
#17173=CARTESIAN_POINT('Origin',(-12.5,-40.5,20.63971317669));
#17174=CARTESIAN_POINT('',(-12.5,-42.5,-12.5));
#17175=CARTESIAN_POINT('',(-12.5,-42.5,20.63971317669));
#17176=CARTESIAN_POINT('Origin',(-12.5,-40.5,-12.5));
#17177=CARTESIAN_POINT('Origin',(0.,0.,-12.5));
#17178=CARTESIAN_POINT('',(-11.1002577388094,-42.5000000000011,-12.5));
#17179=CARTESIAN_POINT('',(0.,-42.5,-12.5));
#17180=CARTESIAN_POINT('',(-13.475,-48.1,-12.5));
#17181=CARTESIAN_POINT('',(0.,-48.1,-12.5));
#17182=CARTESIAN_POINT('',(-13.475,-43.87105808376,-12.5));
#17183=CARTESIAN_POINT('',(-13.475,0.,-12.5));
#17184=CARTESIAN_POINT('',(-13.475,-43.87105808376,-12.5));
#17185=CARTESIAN_POINT('Origin',(-15.,-48.1,-14.5));
#17186=CARTESIAN_POINT('',(-13.475,-48.1,-12.5));
#17187=CARTESIAN_POINT('',(0.,-48.1,-14.5));
#17188=CARTESIAN_POINT('Origin',(0.,0.,-14.5));
#17189=CARTESIAN_POINT('Origin',(0.,0.,-14.5));
#17190=CARTESIAN_POINT('',(-19.1,-39.25,-14.5));
#17191=CARTESIAN_POINT('',(0.,-39.25,-14.5));
#17192=CARTESIAN_POINT('',(-19.1,-21.975,-14.5));
#17193=CARTESIAN_POINT('',(-19.1,0.,-14.5));
#17194=CARTESIAN_POINT('',(0.,-21.975,-14.5));
#17195=CARTESIAN_POINT('Origin',(-13.75,-39.25,-5.));
#17196=CARTESIAN_POINT('',(-19.1,-39.25,-5.));
#17197=CARTESIAN_POINT('',(-19.1,-39.25,-5.));
#17198=CARTESIAN_POINT('',(-13.75,-39.25,-5.));
#17199=CARTESIAN_POINT('Origin',(-14.5,-38.525,12.5));
#17200=CARTESIAN_POINT('',(-13.75,-38.525,12.5));
#17201=CARTESIAN_POINT('',(-14.5,-38.525,12.5));
#17202=CARTESIAN_POINT('',(-13.75,-38.525,-5.));
#17203=CARTESIAN_POINT('',(-13.75,-38.525,12.5));
#17204=CARTESIAN_POINT('',(-14.5,-38.525,-5.));
#17205=CARTESIAN_POINT('Origin',(0.,0.,12.5));
#17206=CARTESIAN_POINT('',(-13.75,-22.475,12.5));
#17207=CARTESIAN_POINT('',(0.,-22.475,12.5));
#17208=CARTESIAN_POINT('',(-13.75,0.,12.5));
#17209=CARTESIAN_POINT('Origin',(-13.75,-22.475,12.5));
#17210=CARTESIAN_POINT('',(-13.75,-22.475,-5.));
#17211=CARTESIAN_POINT('',(-13.75,-22.475,12.5));
#17212=CARTESIAN_POINT('',(-13.75,-22.475,-5.));
#17213=CARTESIAN_POINT('Origin',(-19.1,-21.75,-5.));
#17214=CARTESIAN_POINT('',(-19.1,-21.75,-12.5));
#17215=CARTESIAN_POINT('',(-19.1,-21.75,-5.));
#17216=CARTESIAN_POINT('',(-19.1,-21.75,-5.));
#17217=CARTESIAN_POINT('',(-19.1,-21.75,-5.));
#17218=CARTESIAN_POINT('',(-19.1,-21.75,-12.5));
#17219=CARTESIAN_POINT('Origin',(0.,0.,-12.5));
#17220=CARTESIAN_POINT('',(-19.1,-21.975,-12.5));
#17221=CARTESIAN_POINT('',(0.,-21.975,-12.5));
#17222=CARTESIAN_POINT('',(-19.1,0.,-12.5));
#17223=CARTESIAN_POINT('',(-15.87105808376,-20.475,-12.5));
#17224=CARTESIAN_POINT('',(-14.5,-18.10025773881,-12.5));
#17225=CARTESIAN_POINT('',(0.,-20.475,-12.5));
#17226=CARTESIAN_POINT('Origin',(0.,0.,-12.5));
#17227=CARTESIAN_POINT('',(-14.4421161675114,-18.0000000000008,-12.5));
#17228=CARTESIAN_POINT('',(-15.87105808376,-15.525,-12.5));
#17229=CARTESIAN_POINT('',(-14.44211616751,-18.,-12.5));
#17230=CARTESIAN_POINT('Origin',(0.,0.,-12.5));
#17231=CARTESIAN_POINT('',(0.,-14.025,-12.5));
#17232=CARTESIAN_POINT('',(-15.87105808376,-15.525,-12.5));
#17233=CARTESIAN_POINT('',(0.,-15.525,-12.5));
#17234=CARTESIAN_POINT('',(-15.87105808376,-15.525,-12.5));
#17235=CARTESIAN_POINT('Origin',(-14.5,-14.025,-12.5));
#17236=CARTESIAN_POINT('',(-14.5,-14.025,-14.5));
#17237=CARTESIAN_POINT('Origin',(0.,0.,-14.5));
#17238=CARTESIAN_POINT('',(0.,0.025,-14.5));
#17239=CARTESIAN_POINT('Origin',(-20.1,0.025,-12.5));
#17240=CARTESIAN_POINT('',(-20.1,0.025,-12.5));
#17241=CARTESIAN_POINT('Origin',(0.,0.,-12.5));
#17242=CARTESIAN_POINT('',(-15.87105808376,1.525,-12.5));
#17243=CARTESIAN_POINT('',(-14.5,3.899742261193,-12.5));
#17244=CARTESIAN_POINT('',(0.,1.525,-12.5));
#17245=CARTESIAN_POINT('Origin',(0.,0.,-12.5));
#17246=CARTESIAN_POINT('',(-14.4421161675114,3.99999999999919,-12.5));
#17247=CARTESIAN_POINT('',(-15.87105808376,6.475,-12.5));
#17248=CARTESIAN_POINT('',(-14.44211616751,4.,-12.5));
#17249=CARTESIAN_POINT('Origin',(0.,0.,-12.5));
#17250=CARTESIAN_POINT('',(0.,7.975,-12.5));
#17251=CARTESIAN_POINT('',(-15.87105808376,6.475,-12.5));
#17252=CARTESIAN_POINT('',(0.,6.475,-12.5));
#17253=CARTESIAN_POINT('',(-15.87105808376,6.475,-12.5));
#17254=CARTESIAN_POINT('Origin',(-14.5,7.975,-12.5));
#17255=CARTESIAN_POINT('Origin',(0.,0.,12.5));
#17256=CARTESIAN_POINT('',(-14.4421161675114,3.99999999999919,12.5));
#17257=CARTESIAN_POINT('',(-14.44211616751,4.,12.5));
#17258=CARTESIAN_POINT('',(-14.5,4.100257738807,12.5));
#17259=CARTESIAN_POINT('Origin',(0.,0.,12.5));
#17260=CARTESIAN_POINT('',(0.,0.025,12.5));
#17261=CARTESIAN_POINT('',(-15.87105808376,1.525,12.5));
#17262=CARTESIAN_POINT('',(0.,1.525,12.5));
#17263=CARTESIAN_POINT('',(-14.5,3.899742261193,12.5));
#17264=CARTESIAN_POINT('Origin',(-20.1,0.025,12.5));
#17265=CARTESIAN_POINT('',(-20.1,0.025,14.5));
#17266=CARTESIAN_POINT('Origin',(0.,0.,14.5));
#17267=CARTESIAN_POINT('',(0.,-14.025,14.5));
#17268=CARTESIAN_POINT('Origin',(-14.5,-14.025,12.5));
#17269=CARTESIAN_POINT('',(-14.5,-14.025,12.5));
#17270=CARTESIAN_POINT('Origin',(0.,0.,12.5));
#17271=CARTESIAN_POINT('',(-15.87105808376,-15.525,12.5));
#17272=CARTESIAN_POINT('',(-15.87105808376,-15.525,12.5));
#17273=CARTESIAN_POINT('',(0.,-15.525,12.5));
#17274=CARTESIAN_POINT('Origin',(0.,0.,12.5));
#17275=CARTESIAN_POINT('',(-14.4421161675114,-18.0000000000008,12.5));
#17276=CARTESIAN_POINT('',(-14.44211616751,-18.,12.5));
#17277=CARTESIAN_POINT('',(-14.5,-17.89974226119,12.5));
#17278=CARTESIAN_POINT('Origin',(0.,0.,12.5));
#17279=CARTESIAN_POINT('',(0.,-21.975,12.5));
#17280=CARTESIAN_POINT('',(-15.87105808376,-20.475,12.5));
#17281=CARTESIAN_POINT('',(0.,-20.475,12.5));
#17282=CARTESIAN_POINT('',(-14.5,-18.10025773881,12.5));
#17283=CARTESIAN_POINT('Origin',(-20.1,-21.975,12.5));
#17284=CARTESIAN_POINT('',(-20.1,-21.975,14.5));
#17285=CARTESIAN_POINT('Origin',(0.,0.,14.5));
#17286=CARTESIAN_POINT('Origin',(0.,0.,14.5));
#17287=CARTESIAN_POINT('Origin',(-20.1,6.475,-12.5));
#17288=CARTESIAN_POINT('',(-15.87105808376,6.475,-14.5));
#17289=CARTESIAN_POINT('',(-15.87105808376,6.475,-12.5));
#17290=CARTESIAN_POINT('',(-20.1,6.475,-14.5));
#17291=CARTESIAN_POINT('Origin',(0.,0.,-14.5));
#17292=CARTESIAN_POINT('',(13.475,-43.87105808376,-14.5));
#17293=CARTESIAN_POINT('',(13.475,-43.87105808376,-14.5));
#17294=CARTESIAN_POINT('',(11.,-42.44211616751,-14.5));
#17295=CARTESIAN_POINT('',(11.,-42.44211616751,-14.5));
#17296=CARTESIAN_POINT('',(8.525,-43.87105808376,-14.5));
#17297=CARTESIAN_POINT('',(8.525,-43.87105808376,-14.5));
#17298=CARTESIAN_POINT('',(8.525,0.,-14.5));
#17299=CARTESIAN_POINT('Origin',(0.,0.,-14.5));
#17300=CARTESIAN_POINT('',(15.8710580837579,-15.5249999999988,-14.5));
#17301=CARTESIAN_POINT('',(0.,-15.525,-14.5));
#17302=CARTESIAN_POINT('',(14.44211616751,-18.,-14.5));
#17303=CARTESIAN_POINT('',(14.44211616751,-18.,-14.5));
#17304=CARTESIAN_POINT('',(15.87105808376,-20.475,-14.5));
#17305=CARTESIAN_POINT('',(15.87105808376,-20.475,-14.5));
#17306=CARTESIAN_POINT('',(0.,-20.475,-14.5));
#17307=CARTESIAN_POINT('Origin',(0.,0.,-14.5));
#17308=CARTESIAN_POINT('',(15.87105808376,6.475,-14.5));
#17309=CARTESIAN_POINT('',(0.,6.475,-14.5));
#17310=CARTESIAN_POINT('',(14.44211616751,4.,-14.5));
#17311=CARTESIAN_POINT('',(14.44211616751,4.,-14.5));
#17312=CARTESIAN_POINT('',(15.87105808376,1.525,-14.5));
#17313=CARTESIAN_POINT('',(15.87105808376,1.525,-14.5));
#17314=CARTESIAN_POINT('',(0.,1.525,-14.5));
#17315=CARTESIAN_POINT('Origin',(0.,0.,-14.5));
#17316=CARTESIAN_POINT('',(-8.52499999999879,-43.8710580837579,-14.5));
#17317=CARTESIAN_POINT('',(-8.525,0.,-14.5));
#17318=CARTESIAN_POINT('',(-10.9999999999988,-42.4421161675121,-14.5));
#17319=CARTESIAN_POINT('',(-11.,-42.44211616751,-14.5));
#17320=CARTESIAN_POINT('',(-13.475,-43.87105808376,-14.5));
#17321=CARTESIAN_POINT('',(-13.475,-43.87105808376,-14.5));
#17322=CARTESIAN_POINT('',(-13.475,-48.1,-14.5));
#17323=CARTESIAN_POINT('Origin',(0.,0.,-14.5));
#17324=CARTESIAN_POINT('',(-15.87105808376,-20.475,-14.5));
#17325=CARTESIAN_POINT('',(0.,-20.475,-14.5));
#17326=CARTESIAN_POINT('',(-14.44211616751,-18.,-14.5));
#17327=CARTESIAN_POINT('',(-14.44211616751,-18.,-14.5));
#17328=CARTESIAN_POINT('',(-15.87105808376,-15.525,-14.5));
#17329=CARTESIAN_POINT('',(-15.87105808376,-15.525,-14.5));
#17330=CARTESIAN_POINT('',(0.,-15.525,-14.5));
#17331=CARTESIAN_POINT('Origin',(0.,0.,-14.5));
#17332=CARTESIAN_POINT('',(-15.87105808376,1.525,-14.5));
#17333=CARTESIAN_POINT('',(0.,1.525,-14.5));
#17334=CARTESIAN_POINT('',(-14.44211616751,4.,-14.5));
#17335=CARTESIAN_POINT('',(-14.44211616751,4.,-14.5));
#17336=CARTESIAN_POINT('',(-15.87105808376,6.475,-14.5));
#17337=CARTESIAN_POINT('Origin',(20.1,1.525,-12.5));
#17338=CARTESIAN_POINT('',(15.87105808376,1.525,-12.5));
#17339=CARTESIAN_POINT('',(15.87105808376,1.525,-12.5));
#17340=CARTESIAN_POINT('',(20.1,1.525,-12.5));
#17341=CARTESIAN_POINT('Origin',(14.5,0.025,-12.5));
#17342=CARTESIAN_POINT('',(14.5,0.025,-14.5));
#17343=CARTESIAN_POINT('',(14.5,0.025,-12.5));
#17344=CARTESIAN_POINT('Origin',(0.,0.,-14.5));
#17345=CARTESIAN_POINT('',(0.,-14.025,-14.5));
#17346=CARTESIAN_POINT('Origin',(20.1,-14.025,-12.5));
#17347=CARTESIAN_POINT('',(20.1,-14.025,-12.5));
#17348=CARTESIAN_POINT('Origin',(15.87105808376,-15.525,-12.5));
#17349=CARTESIAN_POINT('',(15.8710580837595,-15.525,-12.5));
#17350=CARTESIAN_POINT('',(15.87105808376,-15.525,-12.5));
#17351=CARTESIAN_POINT('',(15.87105808376,-15.525,-12.5));
#17352=CARTESIAN_POINT('Origin',(20.1,-20.475,-12.5));
#17353=CARTESIAN_POINT('',(15.87105808376,-20.475,-12.5));
#17354=CARTESIAN_POINT('',(15.87105808376,-20.475,-12.5));
#17355=CARTESIAN_POINT('',(20.1,-20.475,-12.5));
#17356=CARTESIAN_POINT('Origin',(14.5,-21.975,-12.5));
#17357=CARTESIAN_POINT('',(19.1,-21.975,-14.5));
#17358=CARTESIAN_POINT('',(14.5,-21.975,-14.5));
#17359=CARTESIAN_POINT('',(19.1,-21.975,-12.5));
#17360=CARTESIAN_POINT('',(14.5,-21.975,-12.5));
#17361=CARTESIAN_POINT('',(19.1,-21.975,-12.5));
#17362=CARTESIAN_POINT('Origin',(0.,0.,-14.5));
#17363=CARTESIAN_POINT('',(19.1,-39.25,-14.5));
#17364=CARTESIAN_POINT('',(19.1,0.,-14.5));
#17365=CARTESIAN_POINT('',(0.,-39.25,-14.5));
#17366=CARTESIAN_POINT('Origin',(0.,0.,-14.5));
#17367=CARTESIAN_POINT('',(-15.,-48.1,-14.5));
#17368=CARTESIAN_POINT('Origin',(8.525,-48.1,-12.5));
#17369=CARTESIAN_POINT('',(8.525,-43.87105808376,-12.5));
#17370=CARTESIAN_POINT('',(8.525,-43.87105808376,-12.5));
#17371=CARTESIAN_POINT('',(8.525,-48.1,-12.5));
#17372=CARTESIAN_POINT('Origin',(7.025,-42.5,-12.5));
#17373=CARTESIAN_POINT('',(7.025,-42.5,-14.5));
#17374=CARTESIAN_POINT('',(7.025,-42.5,-14.5));
#17375=CARTESIAN_POINT('',(7.025,-42.5,-12.5));
#17376=CARTESIAN_POINT('',(7.025,-42.5,-12.5));
#17377=CARTESIAN_POINT('',(7.025,-42.5,-12.5));
#17378=CARTESIAN_POINT('Origin',(0.,0.,-14.5));
#17379=CARTESIAN_POINT('',(-7.025,-42.5,-14.5));
#17380=CARTESIAN_POINT('',(-7.025,0.,-14.5));
#17381=CARTESIAN_POINT('',(0.,-42.5,-14.5));
#17382=CARTESIAN_POINT('Origin',(-7.025,-48.1,-12.5));
#17383=CARTESIAN_POINT('',(-7.025,-42.5,-12.5));
#17384=CARTESIAN_POINT('',(-7.025,-48.1,-12.5));
#17385=CARTESIAN_POINT('',(-7.025,-42.5,-12.5));
#17386=CARTESIAN_POINT('Origin',(-8.525,-43.87105808376,-12.5));
#17387=CARTESIAN_POINT('',(-8.52499999999757,-43.8710580837558,-12.5));
#17388=CARTESIAN_POINT('',(-8.525,-43.87105808376,-12.5));
#17389=CARTESIAN_POINT('',(-8.525,-43.87105808376,-12.5));
#17390=CARTESIAN_POINT('Origin',(-20.1,-21.975,-12.5));
#17391=CARTESIAN_POINT('',(-19.1,-21.975,-12.5));
#17392=CARTESIAN_POINT('Origin',(-15.87105808376,-20.475,-12.5));
#17393=CARTESIAN_POINT('',(-15.87105808376,-20.475,-12.5));
#17394=CARTESIAN_POINT('Origin',(-20.1,-15.525,-12.5));
#17395=CARTESIAN_POINT('',(-15.87105808376,-15.525,-12.5));
#17396=CARTESIAN_POINT('Origin',(-15.87105808376,1.525,-12.5));
#17397=CARTESIAN_POINT('',(-15.87105808376,1.525,-12.5));
#17398=CARTESIAN_POINT('Origin',(-6.65,8.804969405268,-19.));
#17399=CARTESIAN_POINT('Origin',(-6.65,9.000000000629,-19.));
#17400=CARTESIAN_POINT('Origin',(-10.5,9.00000000000002,-19.));
#17401=CARTESIAN_POINT('Origin',(-10.5,5.15,-19.));
#17402=CARTESIAN_POINT('Origin',(-14.67485779376,5.15,-19.));
#17403=CARTESIAN_POINT('Origin',(-13.,5.15,-19.));
#17404=CARTESIAN_POINT('Origin',(-13.,-42.63464535978,-19.));
#17405=CARTESIAN_POINT('Origin',(-13.,5.15,-19.));
#17406=CARTESIAN_POINT('Origin',(-13.,-34.65,-19.));
#17407=CARTESIAN_POINT('Origin',(14.65914844686,-34.65,-19.));
#17408=CARTESIAN_POINT('Origin',(-10.5,-34.65,-19.));
#17409=CARTESIAN_POINT('Origin',(-13.,-34.65,-19.));
#17410=CARTESIAN_POINT('Origin',(-10.5000000000001,-38.5000000000001,-19.0000000000001));
#17411=CARTESIAN_POINT('Origin',(-6.65,-38.50000000054,-19.));
#17412=CARTESIAN_POINT('Origin',(-6.65,-42.69230397724,-19.));
#17413=CARTESIAN_POINT('Origin',(-6.65,-41.,-19.));
#17414=CARTESIAN_POINT('Origin',(13.69503059473,-41.,-19.));
#17415=CARTESIAN_POINT('Origin',(-6.65,-41.,-19.));
#17416=CARTESIAN_POINT('Origin',(6.65,-41.,-19.));
#17417=CARTESIAN_POINT('Origin',(6.65,9.717758793986,-19.));
#17418=CARTESIAN_POINT('Origin',(6.65,-38.5,-19.));
#17419=CARTESIAN_POINT('Origin',(6.65,-41.,-19.));
#17420=CARTESIAN_POINT('Origin',(10.5,-38.5,-19.));
#17421=CARTESIAN_POINT('Origin',(10.50000000054,-34.65,-19.));
#17422=CARTESIAN_POINT('Origin',(14.65914844686,-34.65,-19.));
#17423=CARTESIAN_POINT('Origin',(13.,-34.65,-19.));
#17424=CARTESIAN_POINT('Origin',(13.,9.639713176691,-19.));
#17425=CARTESIAN_POINT('Origin',(13.,-34.65,-19.));
#17426=CARTESIAN_POINT('Origin',(13.,5.15,-19.));
#17427=CARTESIAN_POINT('Origin',(-14.67485779376,5.15,-19.));
#17428=CARTESIAN_POINT('Origin',(10.5,5.15,-19.));
#17429=CARTESIAN_POINT('Origin',(13.,5.15,-19.));
#17430=CARTESIAN_POINT('Origin',(10.5,8.99999999999997,-19.));
#17431=CARTESIAN_POINT('Origin',(6.65,9.,-19.));
#17432=CARTESIAN_POINT('Origin',(6.65,9.639713176691,-19.));
#17433=CARTESIAN_POINT('Origin',(18.417,7.975,-12.5));
#17434=CARTESIAN_POINT('',(18.417,7.975,-12.5));
#17435=CARTESIAN_POINT('Origin',(0.,0.,-12.5));
#17436=CARTESIAN_POINT('',(15.87105808376,6.475,-12.5));
#17437=CARTESIAN_POINT('',(14.5,4.100257738807,-12.5));
#17438=CARTESIAN_POINT('',(0.,6.475,-12.5));
#17439=CARTESIAN_POINT('Origin',(15.87105808376,6.475,-12.5));
#17440=CARTESIAN_POINT('',(15.87105808376,6.475,-12.5));
#17441=CARTESIAN_POINT('Origin',(18.417,7.975,12.5));
#17442=CARTESIAN_POINT('',(18.417,7.975,12.5));
#17443=CARTESIAN_POINT('Origin',(0.,0.,14.5));
#17444=CARTESIAN_POINT('',(0.,-21.975,14.5));
#17445=CARTESIAN_POINT('Origin',(14.5,-21.975,12.5));
#17446=CARTESIAN_POINT('',(14.5,-21.975,12.5));
#17447=CARTESIAN_POINT('Origin',(0.,0.,12.5));
#17448=CARTESIAN_POINT('',(15.87105808376,-20.475,12.5));
#17449=CARTESIAN_POINT('',(15.87105808376,-20.475,12.5));
#17450=CARTESIAN_POINT('',(0.,-20.475,12.5));
#17451=CARTESIAN_POINT('Origin',(0.,0.,12.5));
#17452=CARTESIAN_POINT('',(14.4421161675114,-17.9999999999992,12.5));
#17453=CARTESIAN_POINT('',(14.44211616751,-18.,12.5));
#17454=CARTESIAN_POINT('',(14.5,-18.10025773881,12.5));
#17455=CARTESIAN_POINT('Origin',(0.,0.,12.5));
#17456=CARTESIAN_POINT('',(0.,-14.025,12.5));
#17457=CARTESIAN_POINT('',(15.87105808376,-15.525,12.5));
#17458=CARTESIAN_POINT('',(0.,-15.525,12.5));
#17459=CARTESIAN_POINT('',(14.5,-17.89974226119,12.5));
#17460=CARTESIAN_POINT('Origin',(20.1,-14.025,12.5));
#17461=CARTESIAN_POINT('',(20.1,-14.025,14.5));
#17462=CARTESIAN_POINT('Origin',(0.,0.,14.5));
#17463=CARTESIAN_POINT('',(0.,0.025,14.5));
#17464=CARTESIAN_POINT('Origin',(14.5,0.025,12.5));
#17465=CARTESIAN_POINT('',(14.5,0.025,12.5));
#17466=CARTESIAN_POINT('Origin',(0.,0.,12.5));
#17467=CARTESIAN_POINT('',(15.87105808376,1.525,12.5));
#17468=CARTESIAN_POINT('',(15.87105808376,1.525,12.5));
#17469=CARTESIAN_POINT('',(0.,1.525,12.5));
#17470=CARTESIAN_POINT('Origin',(0.,0.,12.5));
#17471=CARTESIAN_POINT('',(14.4421161675114,4.00000000000081,12.5));
#17472=CARTESIAN_POINT('',(14.44211616751,4.,12.5));
#17473=CARTESIAN_POINT('',(14.5,3.899742261193,12.5));
#17474=CARTESIAN_POINT('Origin',(0.,0.,12.5));
#17475=CARTESIAN_POINT('',(15.87105808376,6.475,12.5));
#17476=CARTESIAN_POINT('',(0.,6.475,12.5));
#17477=CARTESIAN_POINT('',(14.5,4.100257738807,12.5));
#17478=CARTESIAN_POINT('Origin',(0.,0.,-12.5));
#17479=CARTESIAN_POINT('',(14.44211616751,4.,-12.5));
#17480=CARTESIAN_POINT('',(14.5,3.899742261193,-12.5));
#17481=CARTESIAN_POINT('',(14.44211616751,4.,-12.5));
#17482=CARTESIAN_POINT('Origin',(0.,0.,-12.5));
#17483=CARTESIAN_POINT('',(15.87105808376,1.525,-12.5));
#17484=CARTESIAN_POINT('Origin',(0.,0.,-12.5));
#17485=CARTESIAN_POINT('',(14.5,-17.89974226119,-12.5));
#17486=CARTESIAN_POINT('Origin',(0.,0.,-12.5));
#17487=CARTESIAN_POINT('',(14.44211616751,-18.,-12.5));
#17488=CARTESIAN_POINT('',(14.5,-18.10025773881,-12.5));
#17489=CARTESIAN_POINT('',(14.44211616751,-18.,-12.5));
#17490=CARTESIAN_POINT('Origin',(0.,0.,-12.5));
#17491=CARTESIAN_POINT('',(15.87105808376,-20.475,-12.5));
#17492=CARTESIAN_POINT('',(19.1,-21.75,-12.5));
#17493=CARTESIAN_POINT('',(0.,-21.75,-12.5));
#17494=CARTESIAN_POINT('',(19.1,0.,-12.5));
#17495=CARTESIAN_POINT('Origin',(13.75,-21.75,-5.));
#17496=CARTESIAN_POINT('',(19.1,-21.75,-5.));
#17497=CARTESIAN_POINT('',(19.1,-21.75,-5.));
#17498=CARTESIAN_POINT('',(13.75,-21.75,-5.));
#17499=CARTESIAN_POINT('Origin',(14.5,-22.475,12.5));
#17500=CARTESIAN_POINT('',(13.75,-22.475,12.5));
#17501=CARTESIAN_POINT('',(14.5,-22.475,12.5));
#17502=CARTESIAN_POINT('',(13.75,-22.475,-5.));
#17503=CARTESIAN_POINT('',(13.75,-22.475,12.5));
#17504=CARTESIAN_POINT('',(14.5,-22.475,-5.));
#17505=CARTESIAN_POINT('Origin',(0.,0.,12.5));
#17506=CARTESIAN_POINT('',(13.75,-38.525,12.5));
#17507=CARTESIAN_POINT('',(0.,-38.525,12.5));
#17508=CARTESIAN_POINT('',(13.75,0.,12.5));
#17509=CARTESIAN_POINT('Origin',(13.75,-38.525,12.5));
#17510=CARTESIAN_POINT('',(13.75,-38.525,-5.));
#17511=CARTESIAN_POINT('',(13.75,-38.525,12.5));
#17512=CARTESIAN_POINT('',(13.75,-38.525,-5.));
#17513=CARTESIAN_POINT('Origin',(19.1,-39.25,-5.));
#17514=CARTESIAN_POINT('',(19.1,-39.25,-5.));
#17515=CARTESIAN_POINT('',(19.1,-39.25,-5.));
#17516=CARTESIAN_POINT('',(19.1,-39.25,-5.));
#17517=CARTESIAN_POINT('Origin',(-15.,-48.1,-14.5));
#17518=CARTESIAN_POINT('',(13.475,-48.1,-12.5));
#17519=CARTESIAN_POINT('',(-15.,-48.1,-12.5));
#17520=CARTESIAN_POINT('',(13.475,-48.1,-12.5));
#17521=CARTESIAN_POINT('Origin',(0.,0.,-12.5));
#17522=CARTESIAN_POINT('',(12.5,-42.5,-12.5));
#17523=CARTESIAN_POINT('Origin',(12.5,-40.5,-12.5));
#17524=CARTESIAN_POINT('',(11.10025773881,-42.5000000000001,-12.5));
#17525=CARTESIAN_POINT('',(0.,-42.5,-12.5));
#17526=CARTESIAN_POINT('',(13.475,-43.87105808376,-12.5));
#17527=CARTESIAN_POINT('',(11.10025773881,-42.5,-12.5));
#17528=CARTESIAN_POINT('',(13.475,0.,-12.5));
#17529=CARTESIAN_POINT('Origin',(12.5,-40.5,20.63971317669));
#17530=CARTESIAN_POINT('',(12.5,-42.5,12.5));
#17531=CARTESIAN_POINT('Origin',(12.5,-40.5,12.5));
#17532=CARTESIAN_POINT('',(12.5,-42.5,20.63971317669));
#17533=CARTESIAN_POINT('Origin',(0.,0.,12.5));
#17534=CARTESIAN_POINT('',(13.475,-48.1,12.5));
#17535=CARTESIAN_POINT('',(0.,-48.1,12.5));
#17536=CARTESIAN_POINT('',(13.475,-43.87105808376,12.5));
#17537=CARTESIAN_POINT('',(13.475,0.,12.5));
#17538=CARTESIAN_POINT('',(11.10025773881,-42.5000000000001,12.5));
#17539=CARTESIAN_POINT('',(11.10025773881,-42.5,12.5));
#17540=CARTESIAN_POINT('',(0.,-42.5,12.5));
#17541=CARTESIAN_POINT('Origin',(-15.,-48.1,14.5));
#17542=CARTESIAN_POINT('',(-15.,-48.1,14.5));
#17543=CARTESIAN_POINT('',(13.475,-48.1,12.5));
#17544=CARTESIAN_POINT('Origin',(0.,0.,14.5));
#17545=CARTESIAN_POINT('Origin',(15.87105808376,6.475,12.5));
#17546=CARTESIAN_POINT('',(15.87105808376,6.475,14.5));
#17547=CARTESIAN_POINT('',(15.87105808376,6.475,14.5));
#17548=CARTESIAN_POINT('',(15.87105808376,6.475,12.5));
#17549=CARTESIAN_POINT('Origin',(0.,0.,14.5));
#17550=CARTESIAN_POINT('',(13.475,-43.87105808376,14.5));
#17551=CARTESIAN_POINT('',(13.475,0.,14.5));
#17552=CARTESIAN_POINT('',(8.525,-43.87105808376,14.5));
#17553=CARTESIAN_POINT('',(8.525,0.,14.5));
#17554=CARTESIAN_POINT('',(11.,-42.44211616751,14.5));
#17555=CARTESIAN_POINT('',(8.525,-43.87105808376,14.5));
#17556=CARTESIAN_POINT('',(11.,-42.44211616751,14.5));
#17557=CARTESIAN_POINT('Origin',(0.,0.,14.5));
#17558=CARTESIAN_POINT('',(14.4421161675114,-17.9999999999992,14.5));
#17559=CARTESIAN_POINT('',(15.87105808376,-15.525,14.5));
#17560=CARTESIAN_POINT('',(14.44211616751,-18.,14.5));
#17561=CARTESIAN_POINT('',(0.,-15.525,14.5));
#17562=CARTESIAN_POINT('',(15.87105808376,-20.475,14.5));
#17563=CARTESIAN_POINT('',(0.,-20.475,14.5));
#17564=CARTESIAN_POINT('',(15.87105808376,-20.475,14.5));
#17565=CARTESIAN_POINT('Origin',(0.,0.,14.5));
#17566=CARTESIAN_POINT('',(15.87105808376,1.525,14.5));
#17567=CARTESIAN_POINT('',(0.,1.525,14.5));
#17568=CARTESIAN_POINT('',(14.4421161675114,4.00000000000081,14.5));
#17569=CARTESIAN_POINT('',(15.87105808376,1.525,14.5));
#17570=CARTESIAN_POINT('',(14.44211616751,4.,14.5));
#17571=CARTESIAN_POINT('Origin',(0.,0.,14.5));
#17572=CARTESIAN_POINT('',(-8.52499999999879,-43.8710580837579,14.5));
#17573=CARTESIAN_POINT('',(-8.525,0.,14.5));
#17574=CARTESIAN_POINT('',(-13.475,-43.87105808376,14.5));
#17575=CARTESIAN_POINT('',(-13.475,0.,14.5));
#17576=CARTESIAN_POINT('',(-10.9999999999988,-42.4421161675121,14.5));
#17577=CARTESIAN_POINT('',(-13.475,-43.87105808376,14.5));
#17578=CARTESIAN_POINT('',(-11.,-42.44211616751,14.5));
#17579=CARTESIAN_POINT('Origin',(0.,0.,14.5));
#17580=CARTESIAN_POINT('',(-14.4421161675114,-18.0000000000008,14.5));
#17581=CARTESIAN_POINT('',(-15.87105808376,-20.475,14.5));
#17582=CARTESIAN_POINT('',(-14.44211616751,-18.,14.5));
#17583=CARTESIAN_POINT('',(0.,-20.475,14.5));
#17584=CARTESIAN_POINT('',(-15.87105808376,-15.525,14.5));
#17585=CARTESIAN_POINT('',(0.,-15.525,14.5));
#17586=CARTESIAN_POINT('',(-15.87105808376,-15.525,14.5));
#17587=CARTESIAN_POINT('Origin',(0.,0.,14.5));
#17588=CARTESIAN_POINT('',(-15.87105808376,1.525,14.5));
#17589=CARTESIAN_POINT('',(0.,1.525,14.5));
#17590=CARTESIAN_POINT('',(-14.4421161675114,3.99999999999919,14.5));
#17591=CARTESIAN_POINT('',(-15.87105808376,6.475,14.5));
#17592=CARTESIAN_POINT('',(-14.44211616751,4.,14.5));
#17593=CARTESIAN_POINT('Origin',(20.1,1.525,12.5));
#17594=CARTESIAN_POINT('',(15.87105808376,1.525,12.5));
#17595=CARTESIAN_POINT('Origin',(15.87105808376,-15.525,12.5));
#17596=CARTESIAN_POINT('',(15.87105808376,-15.525,12.5));
#17597=CARTESIAN_POINT('Origin',(20.1,-20.475,12.5));
#17598=CARTESIAN_POINT('',(15.87105808376,-20.475,12.5));
#17599=CARTESIAN_POINT('Origin',(8.525,-48.1,12.5));
#17600=CARTESIAN_POINT('',(8.525,-43.87105808376,12.5));
#17601=CARTESIAN_POINT('',(8.525,-48.1,12.5));
#17602=CARTESIAN_POINT('',(8.525,-43.87105808376,12.5));
#17603=CARTESIAN_POINT('Origin',(7.025,-42.5,12.5));
#17604=CARTESIAN_POINT('',(7.025,-42.5,14.5));
#17605=CARTESIAN_POINT('',(7.025,-42.5,14.5));
#17606=CARTESIAN_POINT('',(7.025,-42.5,12.5));
#17607=CARTESIAN_POINT('',(7.025,-42.5,12.5));
#17608=CARTESIAN_POINT('',(7.025,-42.5,12.5));
#17609=CARTESIAN_POINT('Origin',(0.,0.,14.5));
#17610=CARTESIAN_POINT('',(-7.025,-42.5,14.5));
#17611=CARTESIAN_POINT('',(-7.025,0.,14.5));
#17612=CARTESIAN_POINT('',(0.,-42.5,14.5));
#17613=CARTESIAN_POINT('Origin',(-7.025,-48.1,12.5));
#17614=CARTESIAN_POINT('',(-7.025,-42.5,12.5));
#17615=CARTESIAN_POINT('',(-7.025,-48.1,12.5));
#17616=CARTESIAN_POINT('',(-7.025,-42.5,12.5));
#17617=CARTESIAN_POINT('Origin',(-8.525,-43.87105808376,12.5));
#17618=CARTESIAN_POINT('',(-8.52499999999757,-43.8710580837558,12.5));
#17619=CARTESIAN_POINT('',(-8.525,-43.87105808376,12.5));
#17620=CARTESIAN_POINT('',(-8.525,-43.87105808376,12.5));
#17621=CARTESIAN_POINT('Origin',(-15.87105808376,-20.475,12.5));
#17622=CARTESIAN_POINT('',(-15.87105808376,-20.475,12.5));
#17623=CARTESIAN_POINT('Origin',(-20.1,-15.525,12.5));
#17624=CARTESIAN_POINT('',(-15.87105808376,-15.525,12.5));
#17625=CARTESIAN_POINT('Origin',(-15.87105808376,1.525,12.5));
#17626=CARTESIAN_POINT('',(-15.87105808376,1.525,12.5));
#17627=CARTESIAN_POINT('Origin',(0.,0.,25.));
#17628=CARTESIAN_POINT('Origin',(-15.87105808376,6.475,12.5));
#17629=CARTESIAN_POINT('',(-14.4421161675142,3.99999999999757,12.5));
#17630=CARTESIAN_POINT('Origin',(-13.475,-48.1,12.5));
#17631=CARTESIAN_POINT('',(-13.475,-43.87105808376,12.5));
#17632=CARTESIAN_POINT('Origin',(-13.475,-43.87105808376,12.5));
#17633=CARTESIAN_POINT('',(-10.9999999999983,-42.4421161675124,12.5));
#17634=CARTESIAN_POINT('',(-13.475,-43.87105808376,12.5));
#17635=CARTESIAN_POINT('',(-10.9999999999976,-42.4421161675142,12.5));
#17636=CARTESIAN_POINT('Origin',(-14.5,-42.5,-20.5));
#17637=CARTESIAN_POINT('',(10.8997422611913,-42.5000000000022,-12.5));
#17638=CARTESIAN_POINT('',(-14.5,-42.5,-12.5));
#17639=CARTESIAN_POINT('',(10.8997422611913,-42.5000000000022,12.5));
#17640=CARTESIAN_POINT('',(-14.5,-42.5,12.5));
#17641=CARTESIAN_POINT('',(-14.5,-42.5,12.5));
#17642=CARTESIAN_POINT('',(-10.8997422611901,-42.5000000000001,12.5));
#17643=CARTESIAN_POINT('',(-14.5,-42.5,12.5));
#17644=CARTESIAN_POINT('',(-14.5,-42.5,12.5));
#17645=CARTESIAN_POINT('',(-10.8997422611901,-42.5000000000001,-12.5));
#17646=CARTESIAN_POINT('',(-14.5,-42.5,-12.5));
#17647=CARTESIAN_POINT('',(-14.5,-42.5,-12.5));
#17648=CARTESIAN_POINT('',(-14.5,-42.5,-12.5));
#17649=CARTESIAN_POINT('Origin',(-13.475,-43.87105808376,-12.5));
#17650=CARTESIAN_POINT('',(-10.9999999999984,-42.4421161675128,-12.5));
#17651=CARTESIAN_POINT('',(-10.9999999999976,-42.4421161675142,-12.5));
#17652=CARTESIAN_POINT('',(-13.475,-43.87105808376,-12.5));
#17653=CARTESIAN_POINT('',(-13.475,-43.87105808376,-12.5));
#17654=CARTESIAN_POINT('Origin',(-13.475,-48.1,-12.5));
#17655=CARTESIAN_POINT('Origin',(-19.1,-39.25,-5.));
#17656=CARTESIAN_POINT('',(-19.1,-39.25,-5.));
#17657=CARTESIAN_POINT('Origin',(0.,0.,-5.));
#17658=CARTESIAN_POINT('',(-13.75,0.,-5.));
#17659=CARTESIAN_POINT('',(-13.98,-37.95,-5.));
#17660=CARTESIAN_POINT('',(-13.98,-23.05,-5.));
#17661=CARTESIAN_POINT('',(-13.98,0.,-5.));
#17662=CARTESIAN_POINT('',(-18.88,-37.95,-5.));
#17663=CARTESIAN_POINT('',(0.,-37.95,-5.));
#17664=CARTESIAN_POINT('',(-18.88,-23.05,-5.));
#17665=CARTESIAN_POINT('',(-18.88,0.,-5.));
#17666=CARTESIAN_POINT('',(0.,-23.05,-5.));
#17667=CARTESIAN_POINT('Origin',(-13.75,-38.525,12.5));
#17668=CARTESIAN_POINT('Origin',(-14.44211616751,-18.,-12.5));
#17669=CARTESIAN_POINT('',(-14.44211616751,-18.,-12.5));
#17670=CARTESIAN_POINT('Origin',(-15.87105808376,-15.525,-12.5));
#17671=CARTESIAN_POINT('Origin',(-14.44211616751,4.,-12.5));
#17672=CARTESIAN_POINT('',(-14.44211616751,4.,-12.5));
#17673=CARTESIAN_POINT('Origin',(-15.87105808376,6.475,-12.5));
#17674=CARTESIAN_POINT('Origin',(-14.44211616751,4.,12.5));
#17675=CARTESIAN_POINT('Origin',(-15.87105808376,-15.525,12.5));
#17676=CARTESIAN_POINT('',(-14.4421161675142,-18.0000000000024,12.5));
#17677=CARTESIAN_POINT('Origin',(-14.44211616751,-18.,12.5));
#17678=CARTESIAN_POINT('Origin',(13.475,-43.87105808376,-12.5));
#17679=CARTESIAN_POINT('',(13.475,-43.87105808376,-12.5));
#17680=CARTESIAN_POINT('Origin',(11.,-42.44211616751,-12.5));
#17681=CARTESIAN_POINT('',(11.0000000000008,-42.4421161675114,-12.5));
#17682=CARTESIAN_POINT('',(11.,-42.44211616751,-12.5));
#17683=CARTESIAN_POINT('',(11.,-42.44211616751,-12.5));
#17684=CARTESIAN_POINT('Origin',(8.525,-43.87105808376,-12.5));
#17685=CARTESIAN_POINT('',(8.525,-43.87105808376,-12.5));
#17686=CARTESIAN_POINT('',(8.525,-43.87105808376,-12.5));
#17687=CARTESIAN_POINT('Origin',(14.44211616751,-18.,-12.5));
#17688=CARTESIAN_POINT('',(14.44211616751,-18.,-12.5));
#17689=CARTESIAN_POINT('Origin',(15.87105808376,-20.475,-12.5));
#17690=CARTESIAN_POINT('Origin',(14.44211616751,4.,-12.5));
#17691=CARTESIAN_POINT('',(14.44211616751,4.,-12.5));
#17692=CARTESIAN_POINT('Origin',(15.87105808376,1.525,-12.5));
#17693=CARTESIAN_POINT('Origin',(-11.,-42.44211616751,-12.5));
#17694=CARTESIAN_POINT('',(-11.,-42.44211616751,-12.5));
#17695=CARTESIAN_POINT('',(-11.,-42.44211616751,-12.5));
#17696=CARTESIAN_POINT('Origin',(19.1,-21.75,-5.));
#17697=CARTESIAN_POINT('',(19.1,-21.75,-5.));
#17698=CARTESIAN_POINT('Origin',(0.,0.,-12.5));
#17699=CARTESIAN_POINT('Origin',(0.,0.,-12.5));
#17700=CARTESIAN_POINT('Origin',(-13.,5.15,-19.));
#17701=CARTESIAN_POINT('Ctrl Pts',(-14.5000000000002,5.14999999999998,-18.9999999999996));
#17702=CARTESIAN_POINT('Ctrl Pts',(-14.5,5.1502683704716,-19.0070720743157));
#17703=CARTESIAN_POINT('Ctrl Pts',(-14.5008952119779,5.15081623233879,-19.0450824562991));
#17704=CARTESIAN_POINT('Ctrl Pts',(-14.4931017851657,5.16101344797881,-19.1473283610123));
#17705=CARTESIAN_POINT('Ctrl Pts',(-14.4888014238203,5.16614762734179,-19.1889301853698));
#17706=CARTESIAN_POINT('Ctrl Pts',(-14.4769322259441,5.17896676324241,-19.2616359812616));
#17707=CARTESIAN_POINT('Ctrl Pts',(-14.4720622413096,5.18410167008481,-19.287578866658));
#17708=CARTESIAN_POINT('Ctrl Pts',(-14.4629416839796,5.19347468131139,-19.3288153342604));
#17709=CARTESIAN_POINT('Ctrl Pts',(-14.4579266625362,5.19857937379608,-19.35001262557));
#17710=CARTESIAN_POINT('Ctrl Pts',(-14.4511743173673,5.20535340038314,-19.3756863417983));
#17711=CARTESIAN_POINT('Ctrl Pts',(-14.4480754803313,5.20844138893622,-19.3868828151978));
#17712=CARTESIAN_POINT('Ctrl Pts',(-14.4459627179149,5.21054216771168,-19.3943891095122));
#17713=CARTESIAN_POINT('Ctrl Pts',(-14.4444040881137,5.21208770973309,-19.3998091262346));
#17714=CARTESIAN_POINT('Ctrl Pts',(-14.4237756906843,5.23251270441264,-19.470717215959));
#17715=CARTESIAN_POINT('Ctrl Pts',(-14.3993690637851,5.25635306321645,-19.5340649358218));
#17716=CARTESIAN_POINT('Ctrl Pts',(-14.3583270196641,5.29682852688184,-19.6201464487895));
#17717=CARTESIAN_POINT('Ctrl Pts',(-14.3439056403182,5.31110495308435,-19.6473572697992));
#17718=CARTESIAN_POINT('Ctrl Pts',(-14.3139153763737,5.34099752748566,-19.6987524160761));
#17719=CARTESIAN_POINT('Ctrl Pts',(-14.2976357723532,5.3573325510963,-19.7239445600959));
#17720=CARTESIAN_POINT('Ctrl Pts',(-14.251808341393,5.40369189151976,-19.788911112043));
#17721=CARTESIAN_POINT('Ctrl Pts',(-14.2168974150654,5.43964379893236,-19.8306766770307));
#17722=CARTESIAN_POINT('Ctrl Pts',(-14.1571767183151,5.5017717037822,-19.8879120782552));
#17723=CARTESIAN_POINT('Ctrl Pts',(-14.13604578679,5.52383933229555,-19.9060806952842));
#17724=CARTESIAN_POINT('Ctrl Pts',(-14.091226182727,5.57066956248382,-19.9400003402937));
#17725=CARTESIAN_POINT('Ctrl Pts',(-14.0688649668062,5.59405032517479,-19.9549959653081));
#17726=CARTESIAN_POINT('Ctrl Pts',(-13.9898492875009,5.67633337742647,-19.9999263838268));
#17727=CARTESIAN_POINT('Ctrl Pts',(-13.938482954597,5.7289080828448,-20.0192563633749));
#17728=CARTESIAN_POINT('Ctrl Pts',(-13.8667310709799,5.8014471380659,-20.0371046073501));
#17729=CARTESIAN_POINT('Ctrl Pts',(-13.8436826949468,5.82459789936379,-20.0411970669116));
#17730=CARTESIAN_POINT('Ctrl Pts',(-13.8107160108327,5.85760768308144,-20.0451193489524));
#17731=CARTESIAN_POINT('Ctrl Pts',(-13.7946330526942,5.87368517909651,-20.0465257906122));
#17732=CARTESIAN_POINT('Ctrl Pts',(-13.776625690848,5.89167240033343,-20.0473128143698));
#17733=CARTESIAN_POINT('Ctrl Pts',(-13.7690755742853,5.89921476072116,-20.0474791032041));
#17734=CARTESIAN_POINT('Ctrl Pts',(-13.7640799210943,5.90420586521239,-20.0475532708907));
#17735=CARTESIAN_POINT('Ctrl Pts',(-13.7625698364558,5.90571455194702,-20.0475716004378));
#17736=CARTESIAN_POINT('Ctrl Pts',(-13.6494244217083,6.01879388001767,-20.0476194900863));
#17737=CARTESIAN_POINT('Ctrl Pts',(-13.5458171256965,6.12076447135899,-20.0142261657798));
#17738=CARTESIAN_POINT('Ctrl Pts',(-13.4098535901725,6.25310609308376,-19.9326926928262));
#17739=CARTESIAN_POINT('Ctrl Pts',(-13.3676863827449,6.29390535776389,-19.9002696352502));
#17740=CARTESIAN_POINT('Ctrl Pts',(-13.309816922612,6.34986186513291,-19.8458099780658));
#17741=CARTESIAN_POINT('Ctrl Pts',(-13.2914204068164,6.36764506169195,-19.8266825482732));
#17742=CARTESIAN_POINT('Ctrl Pts',(-13.2652190679446,6.39301754356787,-19.7967518928305));
#17743=CARTESIAN_POINT('Ctrl Pts',(-13.2567173583171,6.40125818545505,-19.7865681729864));
#17744=CARTESIAN_POINT('Ctrl Pts',(-13.2401851344379,6.41730803640871,-19.7658209853051));
#17745=CARTESIAN_POINT('Ctrl Pts',(-13.2329761306639,6.42431648236243,-19.7563895777018));
#17746=CARTESIAN_POINT('Ctrl Pts',(-13.1899088809362,6.46629626026074,-19.6970422219169));
#17747=CARTESIAN_POINT('Ctrl Pts',(-13.1591326285648,6.49695931139492,-19.6442998690099));
#17748=CARTESIAN_POINT('Ctrl Pts',(-13.1187018339531,6.5375766182669,-19.5583253785774));
#17749=CARTESIAN_POINT('Ctrl Pts',(-13.1061787094182,6.5502185564322,-19.528522650004));
#17750=CARTESIAN_POINT('Ctrl Pts',(-13.0830590576994,6.57352678897084,-19.4667920197417));
#17751=CARTESIAN_POINT('Ctrl Pts',(-13.0729825680116,6.5836755636959,-19.4366418158537));
#17752=CARTESIAN_POINT('Ctrl Pts',(-13.0222431195477,6.63416909254319,-19.263206741482));
#17753=CARTESIAN_POINT('Ctrl Pts',(-13.0012748264626,6.65,-19.1269039490329));
#17754=CARTESIAN_POINT('Ctrl Pts',(-13.,6.65000000000009,-18.9999999999985));
#17755=CARTESIAN_POINT('Origin',(-13.,-34.65,-19.));
#17756=CARTESIAN_POINT('Ctrl Pts',(-13.,-36.15,-19.));
#17757=CARTESIAN_POINT('Ctrl Pts',(-13.0022600019962,-36.15,-19.0595135681354));
#17758=CARTESIAN_POINT('Ctrl Pts',(-13.0073620228199,-36.1464573811096,
-19.118348117267));
#17759=CARTESIAN_POINT('Ctrl Pts',(-13.0153053530567,-36.1395493826994,
-19.1760919721841));
#17760=CARTESIAN_POINT('Ctrl Pts',(-13.0166707573576,-36.1383619448793,
-19.1860177470804));
#17761=CARTESIAN_POINT('Ctrl Pts',(-13.0181201082012,-36.1370749459201,
-19.1959113155705));
#17762=CARTESIAN_POINT('Ctrl Pts',(-13.019653390988,-36.1356891362019,-19.2057705877774));
#17763=CARTESIAN_POINT('Ctrl Pts',(-13.0232674597517,-36.1324226731215,
-19.2290096719323));
#17764=CARTESIAN_POINT('Ctrl Pts',(-13.0272781780458,-36.1286470144162,
-19.2518093520673));
#17765=CARTESIAN_POINT('Ctrl Pts',(-13.0317575007099,-36.1243454280086,
-19.2744030248717));
#17766=CARTESIAN_POINT('Ctrl Pts',(-13.0362018078249,-36.1200774677586,
-19.2968200794869));
#17767=CARTESIAN_POINT('Ctrl Pts',(-13.0411074346003,-36.115291625118,-19.31903476708));
#17768=CARTESIAN_POINT('Ctrl Pts',(-13.0465443279275,-36.1099219905614,
-19.3412644238901));
#17769=CARTESIAN_POINT('Ctrl Pts',(-13.051477160096,-36.105050181519,-19.3614331415028));
#17770=CARTESIAN_POINT('Ctrl Pts',(-13.0568473243463,-36.0996972429254,
-19.381614336502));
#17771=CARTESIAN_POINT('Ctrl Pts',(-13.0627066489669,-36.0937789851613,
-19.4019578562263));
#17772=CARTESIAN_POINT('Ctrl Pts',(-13.0781595750661,-36.0781706333824,
-19.4556102696443));
#17773=CARTESIAN_POINT('Ctrl Pts',(-13.0962876949103,-36.0596294661765,
-19.5068516934339));
#17774=CARTESIAN_POINT('Ctrl Pts',(-13.1170615404837,-36.038502108525,-19.5553003604907));
#17775=CARTESIAN_POINT('Ctrl Pts',(-13.1215965043751,-36.0338899723786,
-19.5658767824108));
#17776=CARTESIAN_POINT('Ctrl Pts',(-13.1262574478772,-36.0291544387819,
-19.5763200414124));
#17777=CARTESIAN_POINT('Ctrl Pts',(-13.1310438701045,-36.0242988849141,
-19.586626012918));
#17778=CARTESIAN_POINT('Ctrl Pts',(-13.1443999464778,-36.0107499029783,
-19.6153838900956));
#17779=CARTESIAN_POINT('Ctrl Pts',(-13.1587334900227,-35.9962665987231,
-19.6430731920865));
#17780=CARTESIAN_POINT('Ctrl Pts',(-13.1740297517348,-35.9809201189384,
-19.6696008381985));
#17781=CARTESIAN_POINT('Ctrl Pts',(-13.1816778825908,-35.9732468790461,
-19.6828646612545));
#17782=CARTESIAN_POINT('Ctrl Pts',(-13.1895666820908,-35.9653577656181,
-19.6958380292842));
#17783=CARTESIAN_POINT('Ctrl Pts',(-13.1976935757629,-35.9572615166724,
-19.7085086994028));
#17784=CARTESIAN_POINT('Ctrl Pts',(-13.201757022599,-35.9532133921996,-19.7148440344621));
#17785=CARTESIAN_POINT('Ctrl Pts',(-13.2058799925016,-35.9491134795596,
-19.7211036930482));
#17786=CARTESIAN_POINT('Ctrl Pts',(-13.2100621289874,-35.9449628612145,
-19.727286112916));
#17787=CARTESIAN_POINT('Ctrl Pts',(-13.2129317585397,-35.942114858261,-19.7315282639834));
#17788=CARTESIAN_POINT('Ctrl Pts',(-13.2161072666263,-35.9389722558302,
-19.7361264257704));
#17789=CARTESIAN_POINT('Ctrl Pts',(-13.2190161563155,-35.9360911505925,
-19.7402712176227));
#17790=CARTESIAN_POINT('Ctrl Pts',(-13.2203466199925,-35.9347733949269,
-19.7421669564088));
#17791=CARTESIAN_POINT('Ctrl Pts',(-13.2216213369746,-35.9335109849067,
-19.7439683311337));
#17792=CARTESIAN_POINT('Ctrl Pts',(-13.2227856645689,-35.9323599620334,
-19.7456000774117));
#17793=CARTESIAN_POINT('Ctrl Pts',(-13.2405637498969,-35.9147850261165,
-19.770515165491));
#17794=CARTESIAN_POINT('Ctrl Pts',(-13.2598640476502,-35.8959665645779,
-19.7946098108024));
#17795=CARTESIAN_POINT('Ctrl Pts',(-13.2806405457828,-35.875849115071,-19.8176397930277));
#17796=CARTESIAN_POINT('Ctrl Pts',(-13.3008006762476,-35.8563284815124,
-19.8399865544164));
#17797=CARTESIAN_POINT('Ctrl Pts',(-13.3223509769984,-35.8355841698481,
-19.8613306716612));
#17798=CARTESIAN_POINT('Ctrl Pts',(-13.3452294106231,-35.8135863624122,
-19.8814099110228));
#17799=CARTESIAN_POINT('Ctrl Pts',(-13.3680574656225,-35.7916369944506,
-19.9014449356234));
#17800=CARTESIAN_POINT('Ctrl Pts',(-13.3922081788925,-35.7684389191712,
-19.9202204461223));
#17801=CARTESIAN_POINT('Ctrl Pts',(-13.4175949294794,-35.7439937052078,
-19.9374391968756));
#17802=CARTESIAN_POINT('Ctrl Pts',(-13.4413843218865,-35.721086607056,-19.9535745276667));
#17803=CARTESIAN_POINT('Ctrl Pts',(-13.4662591457732,-35.6970841490617,
-19.9683422449517));
#17804=CARTESIAN_POINT('Ctrl Pts',(-13.4921236616887,-35.6720212156899,
-19.9814718214427));
#17805=CARTESIAN_POINT('Ctrl Pts',(-13.5174413758654,-35.6474881377999,
-19.9943238255531));
#17806=CARTESIAN_POINT('Ctrl Pts',(-13.5437075604159,-35.6219385906434,
-20.0056057520444));
#17807=CARTESIAN_POINT('Ctrl Pts',(-13.5708063058782,-35.5954430912409,
-20.0150455765111));
#17808=CARTESIAN_POINT('Ctrl Pts',(-13.5971431852752,-35.5696924979781,
-20.024220005595));
#17809=CARTESIAN_POINT('Ctrl Pts',(-13.6242665787865,-35.5430481880217,
-20.0316539195612));
#17810=CARTESIAN_POINT('Ctrl Pts',(-13.652043084933,-35.515615010231,-20.0370874936349));
#17811=CARTESIAN_POINT('Ctrl Pts',(-13.6599625404285,-35.5077934422674,
-20.0386366786848));
#17812=CARTESIAN_POINT('Ctrl Pts',(-13.6679349096542,-35.4999080132942,
-20.0400232205253));
#17813=CARTESIAN_POINT('Ctrl Pts',(-13.6759566644634,-35.4919618070296,
-20.0412410399475));
#17814=CARTESIAN_POINT('Ctrl Pts',(-13.689561502004,-35.4784850992684,-20.0433064527889));
#17815=CARTESIAN_POINT('Ctrl Pts',(-13.7033084869127,-35.4648334295818,
-20.0448865414506));
#17816=CARTESIAN_POINT('Ctrl Pts',(-13.7171790381733,-35.4510238866596,
-20.045951700704));
#17817=CARTESIAN_POINT('Ctrl Pts',(-13.7241143138036,-35.4441191151985,
-20.0464842803307));
#17818=CARTESIAN_POINT('Ctrl Pts',(-13.7310804857771,-35.4371748806365,
-20.0468881344733));
#17819=CARTESIAN_POINT('Ctrl Pts',(-13.7380750284009,-35.4301936070775,
-20.0471595809266));
#17820=CARTESIAN_POINT('Ctrl Pts',(-13.7415722997128,-35.4267029702981,
-20.0472953041532));
#17821=CARTESIAN_POINT('Ctrl Pts',(-13.7450766640841,-35.4232030742188,
-20.0473979260404));
#17822=CARTESIAN_POINT('Ctrl Pts',(-13.7485878000069,-35.4196942321784,
-20.0474669897578));
#17823=CARTESIAN_POINT('Ctrl Pts',(-13.7512425760978,-35.417041190496,-20.0475192089568));
#17824=CARTESIAN_POINT('Ctrl Pts',(-13.754398814031,-35.4138864585152,-20.047555584487));
#17825=CARTESIAN_POINT('Ctrl Pts',(-13.7569273746134,-35.41135644911,-20.0475673281272));
#17826=CARTESIAN_POINT('Ctrl Pts',(-13.7577430206946,-35.4105403356773,
-20.0475711163117));
#17827=CARTESIAN_POINT('Ctrl Pts',(-13.7584934884378,-35.4097892758672,
-20.0475727773388));
#17828=CARTESIAN_POINT('Ctrl Pts',(-13.7591411982523,-35.409141187524,-20.0475730516392));
#17829=CARTESIAN_POINT('Ctrl Pts',(-13.7804931212359,-35.3877767862455,
-20.0475820940239));
#17830=CARTESIAN_POINT('Ctrl Pts',(-13.8026529826069,-35.3656086503563,
-20.0462820505238));
#17831=CARTESIAN_POINT('Ctrl Pts',(-13.8254839292651,-35.3427124028573,
-20.0434202458515));
#17832=CARTESIAN_POINT('Ctrl Pts',(-13.8481437806401,-35.3199877400064,
-20.0405798875646));
#17833=CARTESIAN_POINT('Ctrl Pts',(-13.8714648759401,-35.2965453990989,
-20.0362005538921));
#17834=CARTESIAN_POINT('Ctrl Pts',(-13.8952849871958,-35.2725025402055,
-20.0300268827267));
#17835=CARTESIAN_POINT('Ctrl Pts',(-13.9191050984514,-35.248459681312,-20.0238532115612));
#17836=CARTESIAN_POINT('Ctrl Pts',(-13.9434244184388,-35.2238158694878,
-20.0158845175589));
#17837=CARTESIAN_POINT('Ctrl Pts',(-13.9680493372299,-35.1987382984234,
-20.0058661742659));
#17838=CARTESIAN_POINT('Ctrl Pts',(-13.977457672413,-35.1891570203629,-20.002038509595));
#17839=CARTESIAN_POINT('Ctrl Pts',(-13.9871299309948,-35.1792932147603,
-19.9978150359244));
#17840=CARTESIAN_POINT('Ctrl Pts',(-13.9967972145168,-35.1694120988939,
-19.993280617275));
#17841=CARTESIAN_POINT('Ctrl Pts',(-14.0064058021206,-35.1595909772509,
-19.9887737298204));
#17842=CARTESIAN_POINT('Ctrl Pts',(-14.0160093075113,-35.1497530912975,
-19.9839596558358));
#17843=CARTESIAN_POINT('Ctrl Pts',(-14.0253653094095,-35.1401498665673,
-19.9789683807783));
#17844=CARTESIAN_POINT('Ctrl Pts',(-14.0312956955279,-35.1340627760288,
-19.9758046161023));
#17845=CARTESIAN_POINT('Ctrl Pts',(-14.0371270970296,-35.1280697608133,
-19.9725706227735));
#17846=CARTESIAN_POINT('Ctrl Pts',(-14.0428025582102,-35.122232141555,-19.9693088409132));
#17847=CARTESIAN_POINT('Ctrl Pts',(-14.0701611976502,-35.0940918168496,
-19.9535853761576));
#17848=CARTESIAN_POINT('Ctrl Pts',(-14.0963327095386,-35.0670311408392,
-19.9358471136705));
#17849=CARTESIAN_POINT('Ctrl Pts',(-14.1212830788775,-35.0411979198204,
-19.9163451557962));
#17850=CARTESIAN_POINT('Ctrl Pts',(-14.1394468349885,-35.0223914516768,
-19.9021478186064));
#17851=CARTESIAN_POINT('Ctrl Pts',(-14.1569636554044,-35.0042343822968,
-19.887016043089));
#17852=CARTESIAN_POINT('Ctrl Pts',(-14.1738240977961,-34.986766893543,-19.8710482459925));
#17853=CARTESIAN_POINT('Ctrl Pts',(-14.193834365055,-34.966036173068,-19.8520973857473));
#17854=CARTESIAN_POINT('Ctrl Pts',(-14.212919974189,-34.946277284871,-19.8319691573682));
#17855=CARTESIAN_POINT('Ctrl Pts',(-14.2310705495146,-34.9275330934599,
-19.8108271604679));
#17856=CARTESIAN_POINT('Ctrl Pts',(-14.2401458371774,-34.9181609977544,
-19.8002561620177));
#17857=CARTESIAN_POINT('Ctrl Pts',(-14.2489874564823,-34.9090421748539,
-19.7894316869711));
#17858=CARTESIAN_POINT('Ctrl Pts',(-14.2575946377114,-34.9001796687312,
-19.7783738565453));
#17859=CARTESIAN_POINT('Ctrl Pts',(-14.2618982283259,-34.8957484156699,
-19.7728449413323));
#17860=CARTESIAN_POINT('Ctrl Pts',(-14.2663517713433,-34.8911685633083,
-19.7669825101925));
#17861=CARTESIAN_POINT('Ctrl Pts',(-14.2706384453579,-34.8867626882363,
-19.7611973270037));
#17862=CARTESIAN_POINT('Ctrl Pts',(-14.2749251193725,-34.8823568131644,
-19.7554121438149));
#17863=CARTESIAN_POINT('Ctrl Pts',(-14.2790451446463,-34.8781247953313,
-19.7497046604211));
#17864=CARTESIAN_POINT('Ctrl Pts',(-14.2827124379421,-34.8743626807183,
-19.7445201065448));
#17865=CARTESIAN_POINT('Ctrl Pts',(-14.2975068311467,-34.8591857645633,
-19.723604864035));
#17866=CARTESIAN_POINT('Ctrl Pts',(-14.3123312731224,-34.8441459052951,
-19.7008120823653));
#17867=CARTESIAN_POINT('Ctrl Pts',(-14.3269411121185,-34.8294304558811,
-19.6760414162402));
#17868=CARTESIAN_POINT('Ctrl Pts',(-14.3413036352122,-34.8149641101464,
-19.65169006888));
#17869=CARTESIAN_POINT('Ctrl Pts',(-14.3554586875722,-34.800811416631,-19.6254266232903));
#17870=CARTESIAN_POINT('Ctrl Pts',(-14.3691431631417,-34.7871752343393,
-19.5971850248509));
#17871=CARTESIAN_POINT('Ctrl Pts',(-14.377964125389,-34.77838540176,-19.5789805951401));
#17872=CARTESIAN_POINT('Ctrl Pts',(-14.3865034952691,-34.7698922778293,
-19.5601396048537));
#17873=CARTESIAN_POINT('Ctrl Pts',(-14.3947786435268,-34.761666544262,-19.5404841518991));
#17874=CARTESIAN_POINT('Ctrl Pts',(-14.402873396153,-34.7536201291014,-19.5212571816421));
#17875=CARTESIAN_POINT('Ctrl Pts',(-14.4107155303935,-34.745829345794,-19.5012505138998));
#17876=CARTESIAN_POINT('Ctrl Pts',(-14.4182846912925,-34.7382967410889,
-19.4802834787482));
#17877=CARTESIAN_POINT('Ctrl Pts',(-14.4255810866987,-34.7310355845221,
-19.460072020569));
#17878=CARTESIAN_POINT('Ctrl Pts',(-14.432623973438,-34.7240141747685,-19.438967780527));
#17879=CARTESIAN_POINT('Ctrl Pts',(-14.4393582806655,-34.7172656557504,
-19.416800997403));
#17880=CARTESIAN_POINT('Ctrl Pts',(-14.4408457714661,-34.7157750258135,
-19.4119047423225));
#17881=CARTESIAN_POINT('Ctrl Pts',(-14.442318054546,-34.7142978388433,-19.4069566280643));
#17882=CARTESIAN_POINT('Ctrl Pts',(-14.4437742694652,-34.7128346783188,
-19.4019548009798));
#17883=CARTESIAN_POINT('Ctrl Pts',(-14.4516573515213,-34.704913996884,-19.3748778820325));
#17884=CARTESIAN_POINT('Ctrl Pts',(-14.4582965001819,-34.6980624380417,
-19.3489100616057));
#17885=CARTESIAN_POINT('Ctrl Pts',(-14.4639363715387,-34.6921184214563,
-19.3242164996728));
#17886=CARTESIAN_POINT('Ctrl Pts',(-14.4661232996319,-34.689813557385,-19.3146412734141));
#17887=CARTESIAN_POINT('Ctrl Pts',(-14.4681597602534,-34.6876451182921,
-19.3052571195871));
#17888=CARTESIAN_POINT('Ctrl Pts',(-14.4700591413543,-34.6856036616695,
-19.2960717821684));
#17889=CARTESIAN_POINT('Ctrl Pts',(-14.4734579899498,-34.6819505759507,
-19.2796350748798));
#17890=CARTESIAN_POINT('Ctrl Pts',(-14.4764182288969,-34.6787040153216,
-19.2638355067169));
#17891=CARTESIAN_POINT('Ctrl Pts',(-14.4790122221135,-34.675810656934,-19.2487099853794));
#17892=CARTESIAN_POINT('Ctrl Pts',(-14.4803092187218,-34.6743639777403,
-19.2411472247106));
#17893=CARTESIAN_POINT('Ctrl Pts',(-14.4815145444226,-34.6730055973423,
-19.2337529581117));
#17894=CARTESIAN_POINT('Ctrl Pts',(-14.4826367188746,-34.6717290413985,
-19.2265308116014));
#17895=CARTESIAN_POINT('Ctrl Pts',(-14.4833342253485,-34.6709355765022,
-19.2220417645213));
#17896=CARTESIAN_POINT('Ctrl Pts',(-14.4839235679003,-34.6702614216444,
-19.2181274908503));
#17897=CARTESIAN_POINT('Ctrl Pts',(-14.4845504271016,-34.6695394891977,
-19.2138416183871));
#17898=CARTESIAN_POINT('Ctrl Pts',(-14.4849320823828,-34.6690999497757,
-19.2112322192478));
#17899=CARTESIAN_POINT('Ctrl Pts',(-14.4853270789114,-34.6686432749335,
-19.2084849023242));
#17900=CARTESIAN_POINT('Ctrl Pts',(-14.4857618520254,-34.6681384289453,
-19.2053843140591));
#17901=CARTESIAN_POINT('Ctrl Pts',(-14.4877126337078,-34.6658732375746,
-19.1914722974293));
#17902=CARTESIAN_POINT('Ctrl Pts',(-14.4895157198301,-34.6637373060712,
-19.1771171773623));
#17903=CARTESIAN_POINT('Ctrl Pts',(-14.491111562952,-34.6618111725586,-19.1626247306949));
#17904=CARTESIAN_POINT('Ctrl Pts',(-14.4926914399074,-34.6599043097174,
-19.148277278741));
#17905=CARTESIAN_POINT('Ctrl Pts',(-14.4940681658665,-34.6582032367635,
-19.133795531894));
#17906=CARTESIAN_POINT('Ctrl Pts',(-14.495218285289,-34.656748536048,-19.1194852986711));
#17907=CARTESIAN_POINT('Ctrl Pts',(-14.4956431709154,-34.656211129747,-19.1141987064384));
#17908=CARTESIAN_POINT('Ctrl Pts',(-14.496037470133,-34.6557069655761,-19.1089355887219));
#17909=CARTESIAN_POINT('Ctrl Pts',(-14.4964011799049,-34.6552367471062,
-19.1037115483395));
#17910=CARTESIAN_POINT('Ctrl Pts',(-14.4971421310599,-34.6542788159608,
-19.0930691101825));
#17911=CARTESIAN_POINT('Ctrl Pts',(-14.4977897720911,-34.6534179560291,
-19.0820681263714));
#17912=CARTESIAN_POINT('Ctrl Pts',(-14.4983114928388,-34.6526999839116,
-19.0711011991041));
#17913=CARTESIAN_POINT('Ctrl Pts',(-14.4986145484379,-34.6522829303995,
-19.0647307629515));
#17914=CARTESIAN_POINT('Ctrl Pts',(-14.4988757501221,-34.6519133677684,
-19.0583719341073));
#17915=CARTESIAN_POINT('Ctrl Pts',(-14.4990939964136,-34.6515941473328,
-19.052102289881));
#17916=CARTESIAN_POINT('Ctrl Pts',(-14.4993692024711,-34.6511916140436,
-19.044196340793));
#17917=CARTESIAN_POINT('Ctrl Pts',(-14.4995892882439,-34.6508491822811,
-19.0359873571226));
#17918=CARTESIAN_POINT('Ctrl Pts',(-14.4997384781478,-34.6505922042186,
-19.028002615185));
#17919=CARTESIAN_POINT('Ctrl Pts',(-14.499750283177,-34.6505718701782,-19.0273708022445));
#17920=CARTESIAN_POINT('Ctrl Pts',(-14.4997616618496,-34.6505520505088,
-19.0267403944298));
#17921=CARTESIAN_POINT('Ctrl Pts',(-14.4997726153437,-34.6505327471463,
-19.0261116534472));
#17922=CARTESIAN_POINT('Ctrl Pts',(-14.4998099608049,-34.6504669331722,
-19.0239679884345));
#17923=CARTESIAN_POINT('Ctrl Pts',(-14.4998429628733,-34.6504060666365,
-19.0218093966219));
#17924=CARTESIAN_POINT('Ctrl Pts',(-14.4998714305716,-34.6503504002792,
-19.0196359103402));
#17925=CARTESIAN_POINT('Ctrl Pts',(-14.4998913569453,-34.6503114358138,
-19.0181145474362));
#17926=CARTESIAN_POINT('Ctrl Pts',(-14.4998972483018,-34.6502995823162,
-19.0176308556723));
#17927=CARTESIAN_POINT('Ctrl Pts',(-14.4999147420331,-34.6502622818368,
-19.0159905547103));
#17928=CARTESIAN_POINT('Ctrl Pts',(-14.4999222406195,-34.6502462932029,
-19.0152874492243));
#17929=CARTESIAN_POINT('Ctrl Pts',(-14.499931696151,-34.6502258364736,-19.0143718256226));
#17930=CARTESIAN_POINT('Ctrl Pts',(-14.499943037045,-34.6501992580938,-19.0130708039746));
#17931=CARTESIAN_POINT('Ctrl Pts',(-14.4999813878725,-34.650109379565,-19.0086712163251));
#17932=CARTESIAN_POINT('Ctrl Pts',(-14.4999919153336,-34.6500539914906,
-19.0053844415825));
#17933=CARTESIAN_POINT('Ctrl Pts',(-14.4999965710807,-34.6500280644066,
-19.0032071730045));
#17934=CARTESIAN_POINT('Ctrl Pts',(-14.5000010927208,-34.6500028841417,
-19.001092619763));
#17935=CARTESIAN_POINT('Ctrl Pts',(-14.5,-34.6500001237228,-19.0000246345907));
#17936=CARTESIAN_POINT('Ctrl Pts',(-14.5,-34.65,-19.));
#17937=CARTESIAN_POINT('Origin',(-6.65,-41.,-19.));
#17938=CARTESIAN_POINT('Ctrl Pts',(-6.65,-42.5,-18.9999999999996));
#17939=CARTESIAN_POINT('Ctrl Pts',(-6.65226000199757,-42.5,-19.0595135681296));
#17940=CARTESIAN_POINT('Ctrl Pts',(-6.65736202282211,-42.4964573811102,
-19.1183481172583));
#17941=CARTESIAN_POINT('Ctrl Pts',(-6.66530535305908,-42.4895493827004,
-19.1760919721752));
#17942=CARTESIAN_POINT('Ctrl Pts',(-6.66667075735998,-42.4883619448805,
-19.1860177470708));
#17943=CARTESIAN_POINT('Ctrl Pts',(-6.66812010820348,-42.4870749459215,
-19.1959113155602));
#17944=CARTESIAN_POINT('Ctrl Pts',(-6.66965339099016,-42.4856891362034,
-19.2057705877665));
#17945=CARTESIAN_POINT('Ctrl Pts',(-6.67326745976708,-42.4824226731111,
-19.2290096720071));
#17946=CARTESIAN_POINT('Ctrl Pts',(-6.67727817807838,-42.4786470143895,
-19.2518093522287));
#17947=CARTESIAN_POINT('Ctrl Pts',(-6.68175750076314,-42.4743454279614,
-19.2744030251193));
#17948=CARTESIAN_POINT('Ctrl Pts',(-6.68620180789899,-42.4700774676907,
-19.2968200798215));
#17949=CARTESIAN_POINT('Ctrl Pts',(-6.69110743469881,-42.4652916250251,
-19.319034767501));
#17950=CARTESIAN_POINT('Ctrl Pts',(-6.69654432805367,-42.4599219904392,
-19.3412644243957));
#17951=CARTESIAN_POINT('Ctrl Pts',(-6.70147716018822,-42.4550501814286,
-19.3614331418438));
#17952=CARTESIAN_POINT('Ctrl Pts',(-6.70684732439677,-42.4496972428746,
-19.3816143366766));
#17953=CARTESIAN_POINT('Ctrl Pts',(-6.71270664896581,-42.4437789851613,
-19.4019578562263));
#17954=CARTESIAN_POINT('Ctrl Pts',(-6.72815957505023,-42.4281706333941,
-19.4556102696049));
#17955=CARTESIAN_POINT('Ctrl Pts',(-6.74628769488154,-42.409629466202,-19.5068516933656));
#17956=CARTESIAN_POINT('Ctrl Pts',(-6.76706154044398,-42.3885021085632,
-19.5553003604037));
#17957=CARTESIAN_POINT('Ctrl Pts',(-6.77159650434243,-42.3838899724099,
-19.5658767823418));
#17958=CARTESIAN_POINT('Ctrl Pts',(-6.77625744785224,-42.3791544388057,
-19.5763200413613));
#17959=CARTESIAN_POINT('Ctrl Pts',(-6.78104387008779,-42.3742988849298,
-19.5866260128848));
#17960=CARTESIAN_POINT('Ctrl Pts',(-6.79439994646144,-42.3607499029948,
-19.6153838900628));
#17961=CARTESIAN_POINT('Ctrl Pts',(-6.80873349000797,-42.3462665987391,
-19.6430731920569));
#17962=CARTESIAN_POINT('Ctrl Pts',(-6.82402975172317,-42.330920118952,-19.6696008381745));
#17963=CARTESIAN_POINT('Ctrl Pts',(-6.83167788258077,-42.3232468790584,
-19.6828646612334));
#17964=CARTESIAN_POINT('Ctrl Pts',(-6.83956668208268,-42.3153577656287,
-19.6958380292666));
#17965=CARTESIAN_POINT('Ctrl Pts',(-6.847693575757,-42.3072615166807,-19.7085086993891));
#17966=CARTESIAN_POINT('Ctrl Pts',(-6.85175702259416,-42.3032133922067,
-19.7148440344504));
#17967=CARTESIAN_POINT('Ctrl Pts',(-6.85587999249803,-42.2991134795655,
-19.7211036930386));
#17968=CARTESIAN_POINT('Ctrl Pts',(-6.86006212898514,-42.294962861219,-19.7272861129087));
#17969=CARTESIAN_POINT('Ctrl Pts',(-6.86293175853638,-42.2921148582665,
-19.7315282639747));
#17970=CARTESIAN_POINT('Ctrl Pts',(-6.86610726662219,-42.2889722558363,
-19.736126425761));
#17971=CARTESIAN_POINT('Ctrl Pts',(-6.86901615631067,-42.2860911505991,
-19.7402712176126));
#17972=CARTESIAN_POINT('Ctrl Pts',(-6.87034661999027,-42.2847733949309,
-19.7421669564025));
#17973=CARTESIAN_POINT('Ctrl Pts',(-6.87162133697474,-42.2835109849082,
-19.7439683311309));
#17974=CARTESIAN_POINT('Ctrl Pts',(-6.87278566457079,-42.2823599620331,
-19.7456000774116));
#17975=CARTESIAN_POINT('Ctrl Pts',(-6.89056374990032,-42.2647850261135,
-19.7705151654949));
#17976=CARTESIAN_POINT('Ctrl Pts',(-6.90986404765536,-42.2459665645722,
-19.7946098108098));
#17977=CARTESIAN_POINT('Ctrl Pts',(-6.93064054578988,-42.2258491150625,
-19.8176397930381));
#17978=CARTESIAN_POINT('Ctrl Pts',(-6.95080067625634,-42.2063284815013,
-19.8399865544295));
#17979=CARTESIAN_POINT('Ctrl Pts',(-6.97235097700896,-42.1855841698343,
-19.8613306716764));
#17980=CARTESIAN_POINT('Ctrl Pts',(-6.99522941063554,-42.1635863623958,
-19.8814099110395));
#17981=CARTESIAN_POINT('Ctrl Pts',(-7.01805746563467,-42.1416369944338,
-19.9014449356397));
#17982=CARTESIAN_POINT('Ctrl Pts',(-7.04220817890412,-42.1184389191542,
-19.920220446138));
#17983=CARTESIAN_POINT('Ctrl Pts',(-7.06759492949033,-42.093993705191,-19.9374391968903));
#17984=CARTESIAN_POINT('Ctrl Pts',(-7.0913843218999,-42.0710866070363,-19.9535745276827));
#17985=CARTESIAN_POINT('Ctrl Pts',(-7.1162591457892,-42.0470841490393,-19.9683422449684));
#17986=CARTESIAN_POINT('Ctrl Pts',(-7.14212366170743,-42.0220212156647,
-19.9814718214594));
#17987=CARTESIAN_POINT('Ctrl Pts',(-7.16744137588612,-41.9974881377729,
-19.9943238255695));
#17988=CARTESIAN_POINT('Ctrl Pts',(-7.19370756043867,-41.9719385906145,
-20.0056057520601));
#17989=CARTESIAN_POINT('Ctrl Pts',(-7.22080630590297,-41.9454430912103,
-20.0150455765255));
#17990=CARTESIAN_POINT('Ctrl Pts',(-7.24714318530013,-41.9196924979478,
-20.0242200056076));
#17991=CARTESIAN_POINT('Ctrl Pts',(-7.27426657881137,-41.8930481879919,
-20.0316539195719));
#17992=CARTESIAN_POINT('Ctrl Pts',(-7.30204308495783,-41.865615010202,-20.0370874936434));
#17993=CARTESIAN_POINT('Ctrl Pts',(-7.30996254044553,-41.8577934422464,
-20.0386366786911));
#17994=CARTESIAN_POINT('Ctrl Pts',(-7.31793490966327,-41.8499080132814,
-20.0400232205299));
#17995=CARTESIAN_POINT('Ctrl Pts',(-7.32595666446443,-41.841961807025,-20.0412410399506));
#17996=CARTESIAN_POINT('Ctrl Pts',(-7.33956150200486,-41.8284850992645,
-20.0433064527914));
#17997=CARTESIAN_POINT('Ctrl Pts',(-7.35330848691337,-41.8148334295786,
-20.0448865414527));
#17998=CARTESIAN_POINT('Ctrl Pts',(-7.36717903817378,-41.8010238866572,
-20.0459517007055));
#17999=CARTESIAN_POINT('Ctrl Pts',(-7.37411431380399,-41.7941191151964,
-20.0464842803319));
#18000=CARTESIAN_POINT('Ctrl Pts',(-7.38108048577737,-41.7871748806348,
-20.0468881344744));
#18001=CARTESIAN_POINT('Ctrl Pts',(-7.38807502840106,-41.7801936070763,
-20.0471595809274));
#18002=CARTESIAN_POINT('Ctrl Pts',(-7.3915722997129,-41.7767029702971,-20.0472953041539));
#18003=CARTESIAN_POINT('Ctrl Pts',(-7.39507666408421,-41.773203074218,-20.0473979260409));
#18004=CARTESIAN_POINT('Ctrl Pts',(-7.39858780000693,-41.7696942321778,
-20.0474669897582));
#18005=CARTESIAN_POINT('Ctrl Pts',(-7.40124257609955,-41.7670411904938,
-20.0475192089572));
#18006=CARTESIAN_POINT('Ctrl Pts',(-7.40439881403369,-41.7638864585122,
-20.0475555844873));
#18007=CARTESIAN_POINT('Ctrl Pts',(-7.40692737461723,-41.761356449106,-20.0475673281273));
#18008=CARTESIAN_POINT('Ctrl Pts',(-7.40774302069666,-41.7605403356751,
-20.0475711163118));
#18009=CARTESIAN_POINT('Ctrl Pts',(-7.40849348843838,-41.7597892758664,
-20.0475727773389));
#18010=CARTESIAN_POINT('Ctrl Pts',(-7.4091411982522,-41.759141187524,-20.0475730516393));
#18011=CARTESIAN_POINT('Ctrl Pts',(-7.43038644694172,-41.7378835228822,
-20.0475820488475));
#18012=CARTESIAN_POINT('Ctrl Pts',(-7.45243155834306,-41.7158301684825,
-20.0462949982859));
#18013=CARTESIAN_POINT('Ctrl Pts',(-7.47514178883455,-41.6930555178392,
-20.0434630216311));
#18014=CARTESIAN_POINT('Ctrl Pts',(-7.49785201932604,-41.6702808671958,
-20.0406310449764));
#18015=CARTESIAN_POINT('Ctrl Pts',(-7.52122758417547,-41.646784426698,-20.0362536182468));
#18016=CARTESIAN_POINT('Ctrl Pts',(-7.54510514075294,-41.6226840666228,
-20.030073463483));
#18017=CARTESIAN_POINT('Ctrl Pts',(-7.5689826973304,-41.5985837065475,-20.0238933087192));
#18018=CARTESIAN_POINT('Ctrl Pts',(-7.59336244091483,-41.5738789862741,
-20.0159097323494));
#18019=CARTESIAN_POINT('Ctrl Pts',(-7.61804933726504,-41.5487382983867,
-20.005866174252));
#18020=CARTESIAN_POINT('Ctrl Pts',(-7.62745767243902,-41.5391570203356,
-20.0020385095841));
#18021=CARTESIAN_POINT('Ctrl Pts',(-7.6371299310114,-41.5292932147427,-19.9978150359171));
#18022=CARTESIAN_POINT('Ctrl Pts',(-7.64679721452351,-41.5194120988865,
-19.9932806172721));
#18023=CARTESIAN_POINT('Ctrl Pts',(-7.65640580211876,-41.5095909772525,
-19.9887737298213));
#18024=CARTESIAN_POINT('Ctrl Pts',(-7.6660093075004,-41.4997530913086,-19.9839596558412));
#18025=CARTESIAN_POINT('Ctrl Pts',(-7.67536530938891,-41.4901498665887,
-19.9789683807891));
#18026=CARTESIAN_POINT('Ctrl Pts',(-7.68129569551421,-41.4840627760434,
-19.9758046161096));
#18027=CARTESIAN_POINT('Ctrl Pts',(-7.68712709702198,-41.4780697608219,
-19.9725706227775));
#18028=CARTESIAN_POINT('Ctrl Pts',(-7.69280255820763,-41.4722321415587,
-19.9693088409143));
#18029=CARTESIAN_POINT('Ctrl Pts',(-7.72004186109628,-41.4442145630646,
-19.9536539608574));
#18030=CARTESIAN_POINT('Ctrl Pts',(-7.74610437826649,-41.4172671980039,
-19.9360018267513));
#18031=CARTESIAN_POINT('Ctrl Pts',(-7.77095651373042,-41.3915360379521,
-19.916600253824));
#18032=CARTESIAN_POINT('Ctrl Pts',(-7.79638238142,-41.3652108526606,-19.8967507794423));
#18033=CARTESIAN_POINT('Ctrl Pts',(-7.82054133380115,-41.3401586341855,
-19.8750707073972));
#18034=CARTESIAN_POINT('Ctrl Pts',(-7.84340909674202,-41.3164822526811,
-19.8518296258943));
#18035=CARTESIAN_POINT('Ctrl Pts',(-7.85637899306561,-41.3030537326189,
-19.8386479946907));
#18036=CARTESIAN_POINT('Ctrl Pts',(-7.86893375001436,-41.2900668280115,
-19.8249642427768));
#18037=CARTESIAN_POINT('Ctrl Pts',(-7.88107054947811,-41.2775330935049,
-19.8108271605079));
#18038=CARTESIAN_POINT('Ctrl Pts',(-7.89014583714544,-41.2681609977944,
-19.8002561620539));
#18039=CARTESIAN_POINT('Ctrl Pts',(-7.89898745645573,-41.259042174888,-19.7894316870022));
#18040=CARTESIAN_POINT('Ctrl Pts',(-7.90759463769082,-41.2501796687586,
-19.7783738565697));
#18041=CARTESIAN_POINT('Ctrl Pts',(-7.91189822830837,-41.2457484156939,
-19.7728449413534));
#18042=CARTESIAN_POINT('Ctrl Pts',(-7.91635177133052,-41.241168563327,-19.7669825102079));
#18043=CARTESIAN_POINT('Ctrl Pts',(-7.92063844534917,-41.2367626882505,
-19.7611973270139));
#18044=CARTESIAN_POINT('Ctrl Pts',(-7.92492511936782,-41.2323568131741,
-19.7554121438198));
#18045=CARTESIAN_POINT('Ctrl Pts',(-7.92904514464509,-41.2281247953371,
-19.7497046604214));
#18046=CARTESIAN_POINT('Ctrl Pts',(-7.93271243794148,-41.224362680723,-19.7445201065445));
#18047=CARTESIAN_POINT('Ctrl Pts',(-7.94750683115358,-41.2091857645587,
-19.7236048640247));
#18048=CARTESIAN_POINT('Ctrl Pts',(-7.96233127313597,-41.1941459052826,
-19.7008120823441));
#18049=CARTESIAN_POINT('Ctrl Pts',(-7.97694111213783,-41.1794304558619,
-19.6760414162073));
#18050=CARTESIAN_POINT('Ctrl Pts',(-7.99130363522735,-41.1649641101307,
-19.6516900688525));
#18051=CARTESIAN_POINT('Ctrl Pts',(-8.00545868758248,-41.1508114166195,
-19.6254266232702));
#18052=CARTESIAN_POINT('Ctrl Pts',(-8.01914316314706,-41.1371752343325,
-19.5971850248403));
#18053=CARTESIAN_POINT('Ctrl Pts',(-8.02796412505137,-41.1283854020948,
-19.5789805958367));
#18054=CARTESIAN_POINT('Ctrl Pts',(-8.03650349459571,-41.1198922784968,
-19.5601396063383));
#18055=CARTESIAN_POINT('Ctrl Pts',(-8.04477864253932,-41.1116665452412,
-19.5404841542451));
#18056=CARTESIAN_POINT('Ctrl Pts',(-8.05287339486533,-41.1036201303786,
-19.521257184814));
#18057=CARTESIAN_POINT('Ctrl Pts',(-8.06071552882594,-41.0958293473494,
-19.5012505179667));
#18058=CARTESIAN_POINT('Ctrl Pts',(-8.06828468947963,-41.0882967428912,
-19.4802834837703));
#18059=CARTESIAN_POINT('Ctrl Pts',(-8.07558108464161,-41.0810355865701,
-19.4600720265333));
#18060=CARTESIAN_POINT('Ctrl Pts',(-8.08262397116933,-41.0740141770325,
-19.4389677874913));
#18061=CARTESIAN_POINT('Ctrl Pts',(-8.08935827823115,-41.0672656581897,
-19.416801005416));
#18062=CARTESIAN_POINT('Ctrl Pts',(-8.09084576985912,-41.0657750274258,
-19.4119047477233));
#18063=CARTESIAN_POINT('Ctrl Pts',(-8.092318053751,-41.0642978396422,-19.4069566307951));
#18064=CARTESIAN_POINT('Ctrl Pts',(-8.09377426946536,-41.0628346783188,
-19.4019548009793));
#18065=CARTESIAN_POINT('Ctrl Pts',(-8.10165735146519,-41.0549139969409,
-19.3748778822251));
#18066=CARTESIAN_POINT('Ctrl Pts',(-8.10829650007887,-41.048062438149,-19.3489100620048));
#18067=CARTESIAN_POINT('Ctrl Pts',(-8.11393637139768,-41.0421184216066,
-19.3242165002901));
#18068=CARTESIAN_POINT('Ctrl Pts',(-8.11612329956549,-41.0398135574578,
-19.3146412737247));
#18069=CARTESIAN_POINT('Ctrl Pts',(-8.11815976025071,-41.0376451182974,
-19.3052571196084));
#18070=CARTESIAN_POINT('Ctrl Pts',(-8.12005914140593,-41.0356036616162,
-19.2960717819185));
#18071=CARTESIAN_POINT('Ctrl Pts',(-8.12345798999853,-41.0319505758999,
-19.2796350746289));
#18072=CARTESIAN_POINT('Ctrl Pts',(-8.12641822893859,-41.0287040152778,
-19.263835506486));
#18073=CARTESIAN_POINT('Ctrl Pts',(-8.12901222214599,-41.0258106568998,
-19.2487099851899));
#18074=CARTESIAN_POINT('Ctrl Pts',(-8.13030921874969,-41.0243639777107,
-19.2411472245419));
#18075=CARTESIAN_POINT('Ctrl Pts',(-8.13151454444533,-41.0230055973182,
-19.2337529579691));
#18076=CARTESIAN_POINT('Ctrl Pts',(-8.13263671889179,-41.0217290413801,
-19.2265308114904));
#18077=CARTESIAN_POINT('Ctrl Pts',(-8.13333422540494,-41.0209355764389,
-19.2220417641558));
#18078=CARTESIAN_POINT('Ctrl Pts',(-8.13392356800037,-41.0202614215306,
-19.2181274901863));
#18079=CARTESIAN_POINT('Ctrl Pts',(-8.13455042724244,-41.0195394890359,
-19.213841617424));
#18080=CARTESIAN_POINT('Ctrl Pts',(-8.13493208248694,-41.0190999496557,
-19.2112322185235));
#18081=CARTESIAN_POINT('Ctrl Pts',(-8.13532707897324,-41.0186432748618,
-19.2084849018829));
#18082=CARTESIAN_POINT('Ctrl Pts',(-8.13576185202539,-41.0181384289453,
-19.205384314059));
#18083=CARTESIAN_POINT('Ctrl Pts',(-8.13771262528723,-41.0158732473514,
-19.191472357481));
#18084=CARTESIAN_POINT('Ctrl Pts',(-8.1395157048406,-41.0137373238154,-19.1771172970035));
#18085=CARTESIAN_POINT('Ctrl Pts',(-8.14111154314203,-41.0118111964496,
-19.1626249105981));
#18086=CARTESIAN_POINT('Ctrl Pts',(-8.1426914155545,-41.009904339417,-19.1482775162208));
#18087=CARTESIAN_POINT('Ctrl Pts',(-8.14406813862452,-41.0082032705474,
-19.1337958275692));
#18088=CARTESIAN_POINT('Ctrl Pts',(-8.14521825670048,-41.0067485722023,
-19.1194856543808));
#18089=CARTESIAN_POINT('Ctrl Pts',(-8.14564315329892,-41.0062111522699,
-19.1141989416181));
#18090=CARTESIAN_POINT('Ctrl Pts',(-8.14603746204511,-41.0057069760317,
-19.1089357048896));
#18091=CARTESIAN_POINT('Ctrl Pts',(-8.1464011799049,-41.0052367471062,-19.1037115483395));
#18092=CARTESIAN_POINT('Ctrl Pts',(-8.14714211371262,-41.0042788383895,
-19.0930693593443));
#18093=CARTESIAN_POINT('Ctrl Pts',(-8.14778974326321,-41.0034179943571,
-19.0820686180879));
#18094=CARTESIAN_POINT('Ctrl Pts',(-8.14831145781078,-41.0027000321074,
-19.0711019354135));
#18095=CARTESIAN_POINT('Ctrl Pts',(-8.14861452860038,-41.0022829584664,
-19.0647312463215));
#18096=CARTESIAN_POINT('Ctrl Pts',(-8.14887574202692,-41.0019133796073,
-19.058372166662));
#18097=CARTESIAN_POINT('Ctrl Pts',(-8.14909399641365,-41.0015941473328,
-19.052102289881));
#18098=CARTESIAN_POINT('Ctrl Pts',(-8.14936917840194,-41.0011916492509,
-19.0441970322375));
#18099=CARTESIAN_POINT('Ctrl Pts',(-8.14958925209284,-41.0008492385839,
-19.0359887114371));
#18100=CARTESIAN_POINT('Ctrl Pts',(-8.14973844015323,-41.0005922696627,
-19.0280046486033));
#18101=CARTESIAN_POINT('Ctrl Pts',(-8.14975025877486,-41.0005719126821,
-19.0273721541701));
#18102=CARTESIAN_POINT('Ctrl Pts',(-8.14976165011097,-41.0005520711957,
-19.0267410682369));
#18103=CARTESIAN_POINT('Ctrl Pts',(-8.14977261534365,-41.0005327471464,
-19.0261116534473));
#18104=CARTESIAN_POINT('Ctrl Pts',(-8.14980996055586,-41.0004669336114,
-19.023968002731));
#18105=CARTESIAN_POINT('Ctrl Pts',(-8.1498429625613,-41.0004060672224,-19.0218094180695));
#18106=CARTESIAN_POINT('Ctrl Pts',(-8.14987143029062,-41.0003504008284,
-19.0196359317889));
#18107=CARTESIAN_POINT('Ctrl Pts',(-8.149891356706,-41.0003114362984,-19.0181145673715));
#18108=CARTESIAN_POINT('Ctrl Pts',(-8.14989724819467,-41.0002995825442,
-19.017630865736));
#18109=CARTESIAN_POINT('Ctrl Pts',(-8.14991474203512,-41.0002622818322,
-19.0159905545236));
#18110=CARTESIAN_POINT('Ctrl Pts',(-8.1499222406434,-41.0002462931515,-19.0152874469765));
#18111=CARTESIAN_POINT('Ctrl Pts',(-8.14993169617691,-41.0002258364128,
-19.014371822654));
#18112=CARTESIAN_POINT('Ctrl Pts',(-8.14994303704496,-41.0001992580938,
-19.0130708039747));
#18113=CARTESIAN_POINT('Ctrl Pts',(-8.14998138787466,-41.0001093795607,
-19.0086712160803));
#18114=CARTESIAN_POINT('Ctrl Pts',(-8.14999191533451,-41.0000539914869,
-19.0053844413071));
#18115=CARTESIAN_POINT('Ctrl Pts',(-8.14999657108114,-41.0000280644039,
-19.0032071727755));
#18116=CARTESIAN_POINT('Ctrl Pts',(-8.15000109272075,-41.0000028841407,
-19.0010926196445));
#18117=CARTESIAN_POINT('Ctrl Pts',(-8.15,-41.0000001237227,-19.0000246345903));
#18118=CARTESIAN_POINT('Ctrl Pts',(-8.15,-41.,-19.));
#18119=CARTESIAN_POINT('Origin',(6.65000000000001,-41.,-19.));
#18120=CARTESIAN_POINT('Ctrl Pts',(8.15,-41.,-19.));
#18121=CARTESIAN_POINT('Ctrl Pts',(8.15,-41.0002683704757,-19.0070720744224));
#18122=CARTESIAN_POINT('Ctrl Pts',(8.15089521197314,-41.0008162323464,-19.0450824564593));
#18123=CARTESIAN_POINT('Ctrl Pts',(8.14310178514989,-41.0110134479911,-19.1473283611714));
#18124=CARTESIAN_POINT('Ctrl Pts',(8.13880142380088,-41.0161476273552,-19.188930185515));
#18125=CARTESIAN_POINT('Ctrl Pts',(8.12693222592505,-41.0289667632545,-19.2616359813663));
#18126=CARTESIAN_POINT('Ctrl Pts',(8.12206224129179,-41.0341016700959,-19.2875788667459));
#18127=CARTESIAN_POINT('Ctrl Pts',(8.1129416839662,-41.0434746813198,-19.3288153343187));
#18128=CARTESIAN_POINT('Ctrl Pts',(8.10792666252564,-41.0485793738028,-19.3500126256123));
#18129=CARTESIAN_POINT('Ctrl Pts',(8.10117431736145,-41.0553534003873,-19.3756863418201));
#18130=CARTESIAN_POINT('Ctrl Pts',(8.09807548032772,-41.0584413889392,-19.3868828152105));
#18131=CARTESIAN_POINT('Ctrl Pts',(8.09596271791297,-41.0605421677138,-19.3943891095187));
#18132=CARTESIAN_POINT('Ctrl Pts',(8.09440408811516,-41.0620877097325,-19.3998091262296));
#18133=CARTESIAN_POINT('Ctrl Pts',(8.07377569063469,-41.0825127044705,-19.470717216128));
#18134=CARTESIAN_POINT('Ctrl Pts',(8.04936906368569,-41.1063530633271,-19.5340649360603));
#18135=CARTESIAN_POINT('Ctrl Pts',(8.00832701954771,-41.146828527008,-19.6201464490146));
#18136=CARTESIAN_POINT('Ctrl Pts',(7.99390564020552,-41.1611049532053,-19.6473572700006));
#18137=CARTESIAN_POINT('Ctrl Pts',(7.96391537629543,-41.1909975275679,-19.6987524161986));
#18138=CARTESIAN_POINT('Ctrl Pts',(7.94763577235608,-41.2073325510938,-19.7239445600917));
#18139=CARTESIAN_POINT('Ctrl Pts',(7.90180834138563,-41.2536918915203,-19.7889111120554));
#18140=CARTESIAN_POINT('Ctrl Pts',(7.86689741505336,-41.2896437989342,-19.8306766770476));
#18141=CARTESIAN_POINT('Ctrl Pts',(7.80717671830243,-41.3517717037839,-19.8879120782711));
#18142=CARTESIAN_POINT('Ctrl Pts',(7.78604578677822,-41.3738393322969,-19.9060806952984));
#18143=CARTESIAN_POINT('Ctrl Pts',(7.74122618271941,-41.4206695624837,-19.9400003403023));
#18144=CARTESIAN_POINT('Ctrl Pts',(7.71886496684154,-41.4440503251323,-19.9549959652906));
#18145=CARTESIAN_POINT('Ctrl Pts',(7.63984928743279,-41.5263333775036,-19.9999263838627));
#18146=CARTESIAN_POINT('Ctrl Pts',(7.58848295448559,-41.5789080829667,-20.0192563634084));
#18147=CARTESIAN_POINT('Ctrl Pts',(7.51673107086387,-41.6514471381893,-20.0371046073696));
#18148=CARTESIAN_POINT('Ctrl Pts',(7.49368269483908,-41.674597899477,-20.0411970669247));
#18149=CARTESIAN_POINT('Ctrl Pts',(7.46071601075377,-41.7076076831635,-20.0451193489578));
#18150=CARTESIAN_POINT('Ctrl Pts',(7.44463305263381,-41.7236851791591,-20.0465257906142));
#18151=CARTESIAN_POINT('Ctrl Pts',(7.42662569081657,-41.7416724003666,-20.0473128143695));
#18152=CARTESIAN_POINT('Ctrl Pts',(7.41907557426793,-41.7492147607402,-20.0474791032032));
#18153=CARTESIAN_POINT('Ctrl Pts',(7.41407992108659,-41.7542058652218,-20.0475532708895));
#18154=CARTESIAN_POINT('Ctrl Pts',(7.41256983645835,-41.7557145519462,-20.0475716004366));
#18155=CARTESIAN_POINT('Ctrl Pts',(7.29942442170989,-41.86879388002,-20.0476194900838));
#18156=CARTESIAN_POINT('Ctrl Pts',(7.19581712569751,-41.9707644713628,-20.0142261657756));
#18157=CARTESIAN_POINT('Ctrl Pts',(7.05985359017351,-42.1031060930873,-19.9326926928216));
#18158=CARTESIAN_POINT('Ctrl Pts',(7.01768638274607,-42.1439053577669,-19.9002696352458));
#18159=CARTESIAN_POINT('Ctrl Pts',(6.95981692261362,-42.1998618651349,-19.8458099780624));
#18160=CARTESIAN_POINT('Ctrl Pts',(6.94142040681827,-42.2176450616935,-19.8266825482702));
#18161=CARTESIAN_POINT('Ctrl Pts',(6.91521906794671,-42.2430175435688,-19.7967518928284));
#18162=CARTESIAN_POINT('Ctrl Pts',(6.90671735831938,-42.2512581854557,-19.7865681729846));
#18163=CARTESIAN_POINT('Ctrl Pts',(6.89018513444049,-42.2673080364089,-19.765820985304));
#18164=CARTESIAN_POINT('Ctrl Pts',(6.88297613066536,-42.2743164823635,-19.7563895776994));
#18165=CARTESIAN_POINT('Ctrl Pts',(6.83990888094453,-42.3162962602546,-19.6970422219251));
#18166=CARTESIAN_POINT('Ctrl Pts',(6.80913262857571,-42.3469593113872,-19.6442998690234));
#18167=CARTESIAN_POINT('Ctrl Pts',(6.76870183396352,-42.3875766182603,-19.5583253785916));
#18168=CARTESIAN_POINT('Ctrl Pts',(6.75617870942774,-42.4002185564266,-19.5285226500173));
#18169=CARTESIAN_POINT('Ctrl Pts',(6.73305905770577,-42.4235267889677,-19.4667920197505));
#18170=CARTESIAN_POINT('Ctrl Pts',(6.72297996471863,-42.4336781543738,-19.436632917398));
#18171=CARTESIAN_POINT('Ctrl Pts',(6.67225353272374,-42.4841587298309,-19.2632423353073));
#18172=CARTESIAN_POINT('Ctrl Pts',(6.65128524878669,-42.5,-19.1269410506644));
#18173=CARTESIAN_POINT('Ctrl Pts',(6.65,-42.5000000000004,-19.));
#18174=CARTESIAN_POINT('Origin',(13.,-34.65,-19.));
#18175=CARTESIAN_POINT('Ctrl Pts',(14.5000000000002,-34.65,-19.));
#18176=CARTESIAN_POINT('Ctrl Pts',(14.5,-34.6502683704737,-19.0070720743719));
#18177=CARTESIAN_POINT('Ctrl Pts',(14.5008952119754,-34.6508162323428,-19.0450824563835));
#18178=CARTESIAN_POINT('Ctrl Pts',(14.4931017851574,-34.6610134479854,-19.1473283610961));
#18179=CARTESIAN_POINT('Ctrl Pts',(14.4888014238101,-34.666147627349,-19.1889301854463));
#18180=CARTESIAN_POINT('Ctrl Pts',(14.4769322259341,-34.6789667632491,-19.2616359813167));
#18181=CARTESIAN_POINT('Ctrl Pts',(14.4720622413002,-34.684101670091,-19.2875788667042));
#18182=CARTESIAN_POINT('Ctrl Pts',(14.4629416839726,-34.6934746813162,-19.328815334291));
#18183=CARTESIAN_POINT('Ctrl Pts',(14.4579266625307,-34.6985793738,-19.3500126255922));
#18184=CARTESIAN_POINT('Ctrl Pts',(14.4511743173642,-34.7053534003858,-19.3756863418097));
#18185=CARTESIAN_POINT('Ctrl Pts',(14.4480754803294,-34.7084413889382,-19.3868828152043));
#18186=CARTESIAN_POINT('Ctrl Pts',(14.4459627179139,-34.7105421677132,-19.3943891095155));
#18187=CARTESIAN_POINT('Ctrl Pts',(14.4444040881144,-34.7120877097334,-19.3998091262323));
#18188=CARTESIAN_POINT('Ctrl Pts',(14.4237756906626,-34.7325127044393,-19.4707172160325));
#18189=CARTESIAN_POINT('Ctrl Pts',(14.3993690637418,-34.7563530632669,-19.5340649359253));
#18190=CARTESIAN_POINT('Ctrl Pts',(14.3583270196135,-34.7968285269389,-19.6201464488869));
#18191=CARTESIAN_POINT('Ctrl Pts',(14.3439056402692,-34.8111049531388,-19.6473572698862));
#18192=CARTESIAN_POINT('Ctrl Pts',(14.3139153763399,-34.8409975275222,-19.6987524161288));
#18193=CARTESIAN_POINT('Ctrl Pts',(14.2976357723551,-34.8573325510948,-19.7239445600931));
#18194=CARTESIAN_POINT('Ctrl Pts',(14.2518083413899,-34.9036918915172,-19.7889111120491));
#18195=CARTESIAN_POINT('Ctrl Pts',(14.2168974150601,-34.9396437989292,-19.8306766770395));
#18196=CARTESIAN_POINT('Ctrl Pts',(14.1571767183094,-35.0017717037788,-19.887912078264));
#18197=CARTESIAN_POINT('Ctrl Pts',(14.1360457867847,-35.0238393322921,-19.9060806952923));
#18198=CARTESIAN_POINT('Ctrl Pts',(14.0912261827236,-35.0706695624807,-19.9400003402989));
#18199=CARTESIAN_POINT('Ctrl Pts',(14.0688649668324,-35.0940503251426,-19.9549959652954));
#18200=CARTESIAN_POINT('Ctrl Pts',(13.9898492874502,-35.1763333774833,-19.9999263838538));
#18201=CARTESIAN_POINT('Ctrl Pts',(13.9384829545141,-35.2289080829351,-20.0192563634001));
#18202=CARTESIAN_POINT('Ctrl Pts',(13.8667310708931,-35.3014471381576,-20.0371046073651));
#18203=CARTESIAN_POINT('Ctrl Pts',(13.8436826948659,-35.324597899448,-20.0411970669219));
#18204=CARTESIAN_POINT('Ctrl Pts',(13.8107160107728,-35.3576076831428,-20.0451193489571));
#18205=CARTESIAN_POINT('Ctrl Pts',(13.7946330526479,-35.3736851791435,-20.0465257906145));
#18206=CARTESIAN_POINT('Ctrl Pts',(13.776625690823,-35.3916724003586,-20.0473128143704));
#18207=CARTESIAN_POINT('Ctrl Pts',(13.7690755742706,-35.399214760736,-20.0474791032043));
#18208=CARTESIAN_POINT('Ctrl Pts',(13.7640799210867,-35.40420586522,-20.0475532708907));
#18209=CARTESIAN_POINT('Ctrl Pts',(13.7625698364557,-35.4057145519471,-20.0475716004378));
#18210=CARTESIAN_POINT('Ctrl Pts',(13.6494244217085,-35.5187938800181,-20.0476194900858));
#18211=CARTESIAN_POINT('Ctrl Pts',(13.5458171256972,-35.6207644713594,-20.0142261657789));
#18212=CARTESIAN_POINT('Ctrl Pts',(13.4098535901744,-35.7531060930839,-19.9326926928252));
#18213=CARTESIAN_POINT('Ctrl Pts',(13.3676863827473,-35.7939053577639,-19.9002696352492));
#18214=CARTESIAN_POINT('Ctrl Pts',(13.3098169226151,-35.8498618651327,-19.8458099780649));
#18215=CARTESIAN_POINT('Ctrl Pts',(13.2914204068199,-35.8676450616917,-19.8266825482724));
#18216=CARTESIAN_POINT('Ctrl Pts',(13.2652190679484,-35.8930175435675,-19.7967518928298));
#18217=CARTESIAN_POINT('Ctrl Pts',(13.2567173583211,-35.9012581854546,-19.7865681729857));
#18218=CARTESIAN_POINT('Ctrl Pts',(13.2401851344423,-35.9173080364082,-19.7658209853045));
#18219=CARTESIAN_POINT('Ctrl Pts',(13.232976130669,-35.9243164823613,-19.7563895777022));
#18220=CARTESIAN_POINT('Ctrl Pts',(13.1899088809391,-35.9662962602624,-19.6970422219134));
#18221=CARTESIAN_POINT('Ctrl Pts',(13.1591326285664,-35.9969593113973,-19.6442998690046));
#18222=CARTESIAN_POINT('Ctrl Pts',(13.1187018339535,-36.037576618269,-19.5583253785721));
#18223=CARTESIAN_POINT('Ctrl Pts',(13.1061787094184,-36.050218556434,-19.5285226499992));
#18224=CARTESIAN_POINT('Ctrl Pts',(13.0830590576994,-36.0735267889718,-19.4667920197387));
#18225=CARTESIAN_POINT('Ctrl Pts',(13.0729799647175,-36.0836781543729,-19.4366329174011));
#18226=CARTESIAN_POINT('Ctrl Pts',(13.0222535327245,-36.1341587298343,-19.2632423352947));
#18227=CARTESIAN_POINT('Ctrl Pts',(13.0012852487877,-36.15,-19.1269410506513));
#18228=CARTESIAN_POINT('Ctrl Pts',(13.,-36.1500000000004,-18.9999999999985));
#18229=CARTESIAN_POINT('Origin',(13.,5.15,-19.));
#18230=CARTESIAN_POINT('Ctrl Pts',(13.,6.65000000000001,-19.));
#18231=CARTESIAN_POINT('Ctrl Pts',(13.0022571542305,6.65000000000001,-19.0595221284898));
#18232=CARTESIAN_POINT('Ctrl Pts',(13.0073599851969,6.64645638324243,-19.118370455344));
#18233=CARTESIAN_POINT('Ctrl Pts',(13.0153077826458,6.63954451909008,-19.1761328970953));
#18234=CARTESIAN_POINT('Ctrl Pts',(13.01667053524,6.6383593906485,-19.1860370142866));
#18235=CARTESIAN_POINT('Ctrl Pts',(13.0181169221604,6.63707511433721,-19.1959092263041));
#18236=CARTESIAN_POINT('Ctrl Pts',(13.0196469288946,6.63569242536674,-19.2057474553742));
#18237=CARTESIAN_POINT('Ctrl Pts',(13.0232674819402,6.632420479792,-19.2290282876918));
#18238=CARTESIAN_POINT('Ctrl Pts',(13.0272868844424,6.62863709363144,-19.2518709215669));
#18239=CARTESIAN_POINT('Ctrl Pts',(13.0317769417697,6.62432546027521,-19.274508038418));
#18240=CARTESIAN_POINT('Ctrl Pts',(13.0362317965552,6.62004763059737,-19.2969676777902));
#18241=CARTESIAN_POINT('Ctrl Pts',(13.0411499681799,6.61524965955653,-19.3192254433173));
#18242=CARTESIAN_POINT('Ctrl Pts',(13.0466012500809,6.60986557248324,-19.3414979264492));
#18243=CARTESIAN_POINT('Ctrl Pts',(13.0515189167187,6.6050085231037,-19.3615902000146));
#18244=CARTESIAN_POINT('Ctrl Pts',(13.0568704390258,6.59967389575934,-19.381694590447));
#18245=CARTESIAN_POINT('Ctrl Pts',(13.0627066489669,6.59377898516122,-19.4019578562265));
#18246=CARTESIAN_POINT('Ctrl Pts',(13.0781595750536,6.57817063339199,-19.4556102696119));
#18247=CARTESIAN_POINT('Ctrl Pts',(13.0962876948866,6.55962946619751,-19.5068516933774));
#18248=CARTESIAN_POINT('Ctrl Pts',(13.1170615404503,6.53850210855677,-19.5553003604184));
#18249=CARTESIAN_POINT('Ctrl Pts',(13.1215965043478,6.53388997240436,-19.5658767823541));
#18250=CARTESIAN_POINT('Ctrl Pts',(13.1262574478565,6.52915443880112,-19.5763200413713));
#18251=CARTESIAN_POINT('Ctrl Pts',(13.1310438700908,6.52429888492631,-19.5866260128923));
#18252=CARTESIAN_POINT('Ctrl Pts',(13.1443999464643,6.51074990299114,-19.6153838900703));
#18253=CARTESIAN_POINT('Ctrl Pts',(13.1587334900103,6.49626659873545,-19.6430731920639));
#18254=CARTESIAN_POINT('Ctrl Pts',(13.1740297517247,6.48092011894879,-19.6696008381805));
#18255=CARTESIAN_POINT('Ctrl Pts',(13.181677882582,6.47324687905545,-19.6828646612388));
#18256=CARTESIAN_POINT('Ctrl Pts',(13.1895666820834,6.46535776562609,-19.6958380292713));
#18257=CARTESIAN_POINT('Ctrl Pts',(13.1976935757572,6.45726151667853,-19.7085086993931));
#18258=CARTESIAN_POINT('Ctrl Pts',(13.2017570225941,6.45321339220475,-19.714844034454));
#18259=CARTESIAN_POINT('Ctrl Pts',(13.2058799924977,6.44911347956379,-19.7211036930418));
#18260=CARTESIAN_POINT('Ctrl Pts',(13.2100621289846,6.44496286121754,-19.7272861129114));
#18261=CARTESIAN_POINT('Ctrl Pts',(13.2129317585359,6.44211485826487,-19.7315282639777));
#18262=CARTESIAN_POINT('Ctrl Pts',(13.2161072666219,6.43897225583455,-19.736126425764));
#18263=CARTESIAN_POINT('Ctrl Pts',(13.2190161563104,6.43609115059731,-19.7402712176158));
#18264=CARTESIAN_POINT('Ctrl Pts',(13.2203466199895,6.43477339492959,-19.742166956405));
#18265=CARTESIAN_POINT('Ctrl Pts',(13.2216213369736,6.43351098490738,-19.7439683311328));
#18266=CARTESIAN_POINT('Ctrl Pts',(13.2227856645693,6.4323599620326,-19.7456000774129));
#18267=CARTESIAN_POINT('Ctrl Pts',(13.2405637498981,6.41478502611381,-19.7705151654951));
#18268=CARTESIAN_POINT('Ctrl Pts',(13.2598640476524,6.39596656457336,-19.7946098108089));
#18269=CARTESIAN_POINT('Ctrl Pts',(13.2806405457862,6.37584911506449,-19.8176397930363));
#18270=CARTESIAN_POINT('Ctrl Pts',(13.300800676252,6.35632848150411,-19.8399865544269));
#18271=CARTESIAN_POINT('Ctrl Pts',(13.3223509770039,6.33558416983796,-19.8613306716731));
#18272=CARTESIAN_POINT('Ctrl Pts',(13.3452294106298,6.31358636240038,-19.8814099110357));
#18273=CARTESIAN_POINT('Ctrl Pts',(13.368057465629,6.29163699443858,-19.901444935636));
#18274=CARTESIAN_POINT('Ctrl Pts',(13.3922081788985,6.2684389191592,-19.9202204461343));
#18275=CARTESIAN_POINT('Ctrl Pts',(13.4175949294849,6.2439937051961,-19.9374391968868));
#18276=CARTESIAN_POINT('Ctrl Pts',(13.4413843218934,6.22108660704275,-19.9535745276784));
#18277=CARTESIAN_POINT('Ctrl Pts',(13.4662591457815,6.19708414904712,-19.9683422449636));
#18278=CARTESIAN_POINT('Ctrl Pts',(13.4921236616985,6.17202121567392,-19.9814718214543));
#18279=CARTESIAN_POINT('Ctrl Pts',(13.5174413758768,6.14748813778273,-19.9943238255645));
#18280=CARTESIAN_POINT('Ctrl Pts',(13.5437075604289,6.12193859062504,-20.0056057520552));
#18281=CARTESIAN_POINT('Ctrl Pts',(13.5708063058928,6.09544309122141,-20.0150455765209));
#18282=CARTESIAN_POINT('Ctrl Pts',(13.5971431852842,6.06969249796466,-20.0242200056014));
#18283=CARTESIAN_POINT('Ctrl Pts',(13.6242665787895,6.04304818801491,-20.0316539195649));
#18284=CARTESIAN_POINT('Ctrl Pts',(13.6520430849297,6.01561501023135,-20.0370874936366));
#18285=CARTESIAN_POINT('Ctrl Pts',(13.6599625404261,6.00779344226723,-20.0386366786864));
#18286=CARTESIAN_POINT('Ctrl Pts',(13.6679349096527,5.9999080132935,-20.0400232205269));
#18287=CARTESIAN_POINT('Ctrl Pts',(13.6759566644627,5.99196180702828,-20.041241039949));
#18288=CARTESIAN_POINT('Ctrl Pts',(13.6895615020033,5.97848509926772,-20.0433064527899));
#18289=CARTESIAN_POINT('Ctrl Pts',(13.703308486912,5.96483342958172,-20.0448865414512));
#18290=CARTESIAN_POINT('Ctrl Pts',(13.7171790381725,5.95102388666013,-20.0459517007041));
#18291=CARTESIAN_POINT('Ctrl Pts',(13.7241143138028,5.94411911519934,-20.0464842803305));
#18292=CARTESIAN_POINT('Ctrl Pts',(13.7310804857763,5.93717488063765,-20.046888134473));
#18293=CARTESIAN_POINT('Ctrl Pts',(13.7380750284,5.93019360707907,-20.0471595809261));
#18294=CARTESIAN_POINT('Ctrl Pts',(13.7415722997119,5.92670297029977,-20.0472953041526));
#18295=CARTESIAN_POINT('Ctrl Pts',(13.7450766640833,5.92320307422066,-20.0473979260396));
#18296=CARTESIAN_POINT('Ctrl Pts',(13.748587800006,5.91969423218044,-20.0474669897569));
#18297=CARTESIAN_POINT('Ctrl Pts',(13.7512425760986,5.91704119049648,-20.0475192089559));
#18298=CARTESIAN_POINT('Ctrl Pts',(13.7543988140328,5.91388645851485,-20.0475555844859));
#18299=CARTESIAN_POINT('Ctrl Pts',(13.7569273746163,5.91135644910865,-20.047567328126));
#18300=CARTESIAN_POINT('Ctrl Pts',(13.7577430206958,5.91054033567769,-20.0475711163105));
#18301=CARTESIAN_POINT('Ctrl Pts',(13.7584934884376,5.90978927586902,-20.0475727773376));
#18302=CARTESIAN_POINT('Ctrl Pts',(13.7591411982514,5.90914118752659,-20.047573051638));
#18303=CARTESIAN_POINT('Ctrl Pts',(13.7804931212824,5.88777678620174,-20.047582094022));
#18304=CARTESIAN_POINT('Ctrl Pts',(13.8026529826977,5.86560865026827,-20.0462820505162));
#18305=CARTESIAN_POINT('Ctrl Pts',(13.8254839293969,5.84271240272766,-20.0434202458333));
#18306=CARTESIAN_POINT('Ctrl Pts',(13.8481437807667,5.81998773988161,-20.0405798875415));
#18307=CARTESIAN_POINT('Ctrl Pts',(13.8714648760556,5.79654539898445,-20.0362005538657));
#18308=CARTESIAN_POINT('Ctrl Pts',(13.8952849872949,5.77250254010668,-20.0300268827002));
#18309=CARTESIAN_POINT('Ctrl Pts',(13.9191050985343,5.74845968122891,-20.0238532115346));
#18310=CARTESIAN_POINT('Ctrl Pts',(13.9434244185003,5.72381586942578,-20.0158845175354));
#18311=CARTESIAN_POINT('Ctrl Pts',(13.9680493372659,5.69873829838729,-20.0058661742509));
#18312=CARTESIAN_POINT('Ctrl Pts',(13.9774576724419,5.68915702033412,-20.0020385095822));
#18313=CARTESIAN_POINT('Ctrl Pts',(13.9871299310162,5.67929321473919,-19.9978150359143));
#18314=CARTESIAN_POINT('Ctrl Pts',(13.9967972145302,5.66941209888099,-19.9932806172683));
#18315=CARTESIAN_POINT('Ctrl Pts',(14.0064058021273,5.65959097724507,-19.9887737298165));
#18316=CARTESIAN_POINT('Ctrl Pts',(14.0160093075107,5.64975309129928,-19.9839596558353));
#18317=CARTESIAN_POINT('Ctrl Pts',(14.025365309401,5.64014986657743,-19.9789683807821));
#18318=CARTESIAN_POINT('Ctrl Pts',(14.0312956955227,5.63406277603582,-19.9758046161044));
#18319=CARTESIAN_POINT('Ctrl Pts',(14.037127097027,5.62806976081782,-19.972570622774));
#18320=CARTESIAN_POINT('Ctrl Pts',(14.0428025582096,5.62223214155778,-19.9693088409126));
#18321=CARTESIAN_POINT('Ctrl Pts',(14.0700418610936,5.59421456306827,-19.9536539608584));
#18322=CARTESIAN_POINT('Ctrl Pts',(14.096104378259,5.5672671980123,-19.936001826756));
#18323=CARTESIAN_POINT('Ctrl Pts',(14.1209565137182,5.54153603796518,-19.9166002538334));
#18324=CARTESIAN_POINT('Ctrl Pts',(14.1463823814028,5.51521085267855,-19.8967507794566));
#18325=CARTESIAN_POINT('Ctrl Pts',(14.170541333779,5.49015863420826,-19.8750707074175));
#18326=CARTESIAN_POINT('Ctrl Pts',(14.1934090967151,5.46648225270853,-19.8518296259219));
#18327=CARTESIAN_POINT('Ctrl Pts',(14.2063789930497,5.45305373263471,-19.8386479947084));
#18328=CARTESIAN_POINT('Ctrl Pts',(14.2189337500087,5.44006682801658,-19.8249642427839));
#18329=CARTESIAN_POINT('Ctrl Pts',(14.2310705494818,5.42753309350011,-19.8108271605039));
#18330=CARTESIAN_POINT('Ctrl Pts',(14.2401458371487,5.41816099778997,-19.8002561620504));
#18331=CARTESIAN_POINT('Ctrl Pts',(14.2489874564584,5.40904217488394,-19.7894316869992));
#18332=CARTESIAN_POINT('Ctrl Pts',(14.257594637693,5.40017966875506,-19.7783738565673));
#18333=CARTESIAN_POINT('Ctrl Pts',(14.2618982283102,5.39574841569061,-19.7728449413514));
#18334=CARTESIAN_POINT('Ctrl Pts',(14.266351771335,5.39116856332107,-19.7669825102024));
#18335=CARTESIAN_POINT('Ctrl Pts',(14.2706384453547,5.38676268824343,-19.7611973270068));
#18336=CARTESIAN_POINT('Ctrl Pts',(14.2749251193744,5.3823568131658,-19.7554121438113));
#18337=CARTESIAN_POINT('Ctrl Pts',(14.2790451446513,5.37812479532921,-19.7497046604132));
#18338=CARTESIAN_POINT('Ctrl Pts',(14.2827124379418,5.37436268072119,-19.7445201065446));
#18339=CARTESIAN_POINT('Ctrl Pts',(14.2975068310896,5.35918576462267,-19.7236048641156));
#18340=CARTESIAN_POINT('Ctrl Pts',(14.3123312730158,5.34414590540356,-19.7008120825301));
#18341=CARTESIAN_POINT('Ctrl Pts',(14.3269411119702,5.32943045603072,-19.6760414164915));
#18342=CARTESIAN_POINT('Ctrl Pts',(14.3413036350922,5.31496411026688,-19.651690069099));
#18343=CARTESIAN_POINT('Ctrl Pts',(14.355458687486,5.30081141671765,-19.6254266234608));
#18344=CARTESIAN_POINT('Ctrl Pts',(14.3691431630914,5.28717523439047,-19.5971850249547));
#18345=CARTESIAN_POINT('Ctrl Pts',(14.3779641248736,5.27838540227468,-19.5789805962081));
#18346=CARTESIAN_POINT('Ctrl Pts',(14.3865034943007,5.26989227879306,-19.5601396069914));
#18347=CARTESIAN_POINT('Ctrl Pts',(14.3947786421362,5.26166654564463,-19.5404841552019));
#18348=CARTESIAN_POINT('Ctrl Pts',(14.4028733943578,5.25362013088561,-19.521257186065));
#18349=CARTESIAN_POINT('Ctrl Pts',(14.4107155282228,5.24582934795134,-19.5012505195327));
#18350=CARTESIAN_POINT('Ctrl Pts',(14.418284688794,5.23829674357582,-19.4802834856691));
#18351=CARTESIAN_POINT('Ctrl Pts',(14.4255810838726,5.23103558733821,-19.4600720287635));
#18352=CARTESIAN_POINT('Ctrl Pts',(14.4326239703295,5.22401417787251,-19.4389677900705));
#18353=CARTESIAN_POINT('Ctrl Pts',(14.4393582773371,5.2172656590867,-19.4168010083586));
#18354=CARTESIAN_POINT('Ctrl Pts',(14.4408457692689,5.21577502801899,-19.4119047497069));
#18355=CARTESIAN_POINT('Ctrl Pts',(14.4423180534589,5.21429783993652,-19.4069566317984));
#18356=CARTESIAN_POINT('Ctrl Pts',(14.4437742694652,5.21283467831966,-19.4019548009798));
#18357=CARTESIAN_POINT('Ctrl Pts',(14.4516573514295,5.20491399697665,-19.3748778823479));
#18358=CARTESIAN_POINT('Ctrl Pts',(14.4582965000137,5.198062438216,-19.3489100622576));
#18359=CARTESIAN_POINT('Ctrl Pts',(14.4639363713086,5.19211842170032,-19.32421650068));
#18360=CARTESIAN_POINT('Ctrl Pts',(14.4661232995233,5.18981355750282,-19.3146412739223));
#18361=CARTESIAN_POINT('Ctrl Pts',(14.4681597602484,5.18764511830001,-19.3052571196246));
#18362=CARTESIAN_POINT('Ctrl Pts',(14.4700591414377,5.185603661582,-19.2960717817647));
#18363=CARTESIAN_POINT('Ctrl Pts',(14.4734579900285,5.1819505758674,-19.2796350744744));
#18364=CARTESIAN_POINT('Ctrl Pts',(14.4764182289643,5.1787040152497,-19.2638355063437));
#18365=CARTESIAN_POINT('Ctrl Pts',(14.479012222166,5.17581065687768,-19.2487099850732));
#18366=CARTESIAN_POINT('Ctrl Pts',(14.4803092187669,5.17436397769167,-19.241147224438));
#18367=CARTESIAN_POINT('Ctrl Pts',(14.4815145444593,5.17300559730254,-19.2337529578813));
#18368=CARTESIAN_POINT('Ctrl Pts',(14.4826367189024,5.17172904136818,-19.226530811422));
#18369=CARTESIAN_POINT('Ctrl Pts',(14.4833342253862,5.17093557646023,-19.2220417642747));
#18370=CARTESIAN_POINT('Ctrl Pts',(14.4839235679489,5.17026142158958,-19.2181274905262));
#18371=CARTESIAN_POINT('Ctrl Pts',(14.4845504271603,5.16953948913056,-19.2138416179853));
#18372=CARTESIAN_POINT('Ctrl Pts',(14.4849320824255,5.16909994972671,-19.2112322189507));
#18373=CARTESIAN_POINT('Ctrl Pts',(14.4853270789361,5.16864327490485,-19.2084849021477));
#18374=CARTESIAN_POINT('Ctrl Pts',(14.4857618520254,5.16813842894516,-19.2053843140591));
#18375=CARTESIAN_POINT('Ctrl Pts',(14.4877126281297,5.16587324405032,-19.19147233721));
#18376=CARTESIAN_POINT('Ctrl Pts',(14.4895157098943,5.16373731783201,-19.1771172566613));
#18377=CARTESIAN_POINT('Ctrl Pts',(14.4911115498147,5.16181118840159,-19.1626248500009));
#18378=CARTESIAN_POINT('Ctrl Pts',(14.4926914237591,5.15990432941029,-19.1482774362137));
#18379=CARTESIAN_POINT('Ctrl Pts',(14.4940681477991,5.15820325916898,-19.1337957279846));
#18380=CARTESIAN_POINT('Ctrl Pts',(14.495218266324,5.15674856003158,-19.119485534642));
#18381=CARTESIAN_POINT('Ctrl Pts',(14.4956431592295,5.1562111446872,-19.1141988624459));
#18382=CARTESIAN_POINT('Ctrl Pts',(14.4960374647681,5.15570697251119,-19.1089356657791));
#18383=CARTESIAN_POINT('Ctrl Pts',(14.4964011799049,5.15523674710575,-19.1037115483395));
#18384=CARTESIAN_POINT('Ctrl Pts',(14.4971421224544,5.1542788270869,-19.093069233785));
#18385=CARTESIAN_POINT('Ctrl Pts',(14.4977897578427,5.15341797497385,-19.0820683695518));
#18386=CARTESIAN_POINT('Ctrl Pts',(14.4983114755707,5.15270000767031,-19.0711015620904));
#18387=CARTESIAN_POINT('Ctrl Pts',(14.4986145386453,5.15228294425303,-19.0647310015177));
#18388=CARTESIAN_POINT('Ctrl Pts',(14.4988757461215,5.1519133736185,-19.0583720490357));
#18389=CARTESIAN_POINT('Ctrl Pts',(14.4990939964136,5.15159414733242,-19.052102289881));
#18390=CARTESIAN_POINT('Ctrl Pts',(14.4993691946477,5.1511916254878,-19.0441965655395));
#18391=CARTESIAN_POINT('Ctrl Pts',(14.4995892765542,5.15084920049255,-19.0359877955948));
#18392=CARTESIAN_POINT('Ctrl Pts',(14.4997384658976,5.15059222531898,-19.0280032708125));
#18393=CARTESIAN_POINT('Ctrl Pts',(14.499750275309,5.15057188388268,-19.0273712381535));
#18394=CARTESIAN_POINT('Ctrl Pts',(14.4997616580645,5.15055205717901,-19.0267406116957));
#18395=CARTESIAN_POINT('Ctrl Pts',(14.4997726153437,5.15053274714614,-19.0261116534473));
#18396=CARTESIAN_POINT('Ctrl Pts',(14.4998099607338,5.15046693329733,-19.0239679925148));
#18397=CARTESIAN_POINT('Ctrl Pts',(14.4998429627843,5.15040606680349,-19.0218094027432));
#18398=CARTESIAN_POINT('Ctrl Pts',(14.4998714304914,5.15035040043575,-19.0196359164617));
#18399=CARTESIAN_POINT('Ctrl Pts',(14.4998913568769,5.15031143595214,-19.0181145531323));
#18400=CARTESIAN_POINT('Ctrl Pts',(14.499897248271,5.15029958238154,-19.017630858564));
#18401=CARTESIAN_POINT('Ctrl Pts',(14.4999147420333,5.1502622818361,-19.0159905546918));
#18402=CARTESIAN_POINT('Ctrl Pts',(14.499922240626,5.15024629318873,-19.0152874486141));
#18403=CARTESIAN_POINT('Ctrl Pts',(14.4999316961582,5.15022583645654,-19.0143718247977));
#18404=CARTESIAN_POINT('Ctrl Pts',(14.499943037045,5.15019925809364,-19.0130708039746));
#18405=CARTESIAN_POINT('Ctrl Pts',(14.4999813878725,5.15010937956514,-19.0086712163258));
#18406=CARTESIAN_POINT('Ctrl Pts',(14.4999919153334,5.15005399149088,-19.0053844416258));
#18407=CARTESIAN_POINT('Ctrl Pts',(14.4999965710805,5.15002806440687,-19.0032071730684));
#18408=CARTESIAN_POINT('Ctrl Pts',(14.5000010927209,5.15000288414101,-19.0010926197659));
#18409=CARTESIAN_POINT('Ctrl Pts',(14.5,5.15000012372276,-19.0000246345919));
#18410=CARTESIAN_POINT('Ctrl Pts',(14.5,5.15,-19.));
#18411=CARTESIAN_POINT('Origin',(0.,0.,-19.5));
#18412=CARTESIAN_POINT('Origin',(15.87105808376,-20.475,12.5));
#18413=CARTESIAN_POINT('',(14.4421161675142,-17.9999999999976,12.5));
#18414=CARTESIAN_POINT('Origin',(14.44211616751,-18.,12.5));
#18415=CARTESIAN_POINT('Origin',(15.87105808376,1.525,12.5));
#18416=CARTESIAN_POINT('',(14.4421161675142,4.00000000000243,12.5));
#18417=CARTESIAN_POINT('Origin',(14.44211616751,4.,12.5));
#18418=CARTESIAN_POINT('Origin',(0.,0.,-5.));
#18419=CARTESIAN_POINT('',(13.75,0.,-5.));
#18420=CARTESIAN_POINT('',(18.88,-23.05,-5.));
#18421=CARTESIAN_POINT('',(13.98,-23.05,-5.));
#18422=CARTESIAN_POINT('',(0.,-23.05,-5.));
#18423=CARTESIAN_POINT('',(18.88,-37.95,-5.));
#18424=CARTESIAN_POINT('',(18.88,0.,-5.));
#18425=CARTESIAN_POINT('',(13.98,-37.95,-5.));
#18426=CARTESIAN_POINT('',(0.,-37.95,-5.));
#18427=CARTESIAN_POINT('',(13.98,0.,-5.));
#18428=CARTESIAN_POINT('Origin',(13.75,-22.475,12.5));
#18429=CARTESIAN_POINT('Origin',(13.475,-43.87105808376,12.5));
#18430=CARTESIAN_POINT('',(13.475,-43.87105808376,12.5));
#18431=CARTESIAN_POINT('Origin',(11.,-42.44211616751,12.5));
#18432=CARTESIAN_POINT('',(11.0000000000008,-42.4421161675114,12.5));
#18433=CARTESIAN_POINT('',(11.,-42.44211616751,12.5));
#18434=CARTESIAN_POINT('',(11.,-42.44211616751,12.5));
#18435=CARTESIAN_POINT('Origin',(8.525,-43.87105808376,12.5));
#18436=CARTESIAN_POINT('',(8.525,-43.87105808376,12.5));
#18437=CARTESIAN_POINT('',(8.525,-43.87105808376,12.5));
#18438=CARTESIAN_POINT('Origin',(-11.,-42.44211616751,12.5));
#18439=CARTESIAN_POINT('',(-11.,-42.44211616751,12.5));
#18440=CARTESIAN_POINT('',(-11.,-42.44211616751,12.5));
#18441=CARTESIAN_POINT('Origin',(0.,0.,12.5));
#18442=CARTESIAN_POINT('Origin',(0.,0.,12.5));
#18443=CARTESIAN_POINT('Origin',(0.,0.,12.5));
#18444=CARTESIAN_POINT('Origin',(0.,0.,-12.5));
#18445=CARTESIAN_POINT('Origin',(0.,0.,-12.5));
#18446=CARTESIAN_POINT('Origin',(0.,0.,12.5));
#18447=CARTESIAN_POINT('Origin',(-13.98,-23.05,-5.));
#18448=CARTESIAN_POINT('',(-18.88,-23.05,-4.1));
#18449=CARTESIAN_POINT('',(-13.98,-23.05,-4.1));
#18450=CARTESIAN_POINT('',(-13.98,-23.05,-4.1));
#18451=CARTESIAN_POINT('',(-13.98,-23.05,-5.));
#18452=CARTESIAN_POINT('',(-18.88,-23.05,-5.));
#18453=CARTESIAN_POINT('Origin',(-13.98,-37.95,-5.));
#18454=CARTESIAN_POINT('',(-13.98,-37.95,-4.1));
#18455=CARTESIAN_POINT('',(-13.98,-37.95,-4.1));
#18456=CARTESIAN_POINT('',(-13.98,-37.95,-5.));
#18457=CARTESIAN_POINT('Origin',(-18.88,-37.95,-5.));
#18458=CARTESIAN_POINT('',(-18.88,-37.95,-4.1));
#18459=CARTESIAN_POINT('',(-18.88,-37.95,-4.1));
#18460=CARTESIAN_POINT('',(-18.88,-37.95,-5.));
#18461=CARTESIAN_POINT('Origin',(-18.88,-23.05,-5.));
#18462=CARTESIAN_POINT('',(-18.88,-23.05,-4.1));
#18463=CARTESIAN_POINT('Ctrl Pts',(-12.9943339616048,6.64999987669794,-18.9993941238939));
#18464=CARTESIAN_POINT('Ctrl Pts',(-13.2370215098806,6.64999993944614,-19.001183928572));
#18465=CARTESIAN_POINT('Ctrl Pts',(-13.4998389840212,6.64999999595731,-18.742870425708));
#18466=CARTESIAN_POINT('Ctrl Pts',(-13.4997146189277,6.64999995914459,-18.4999999987164));
#18467=CARTESIAN_POINT('Ctrl Pts',(-12.9952528649784,6.65005651677245,-19.1408685056908));
#18468=CARTESIAN_POINT('Ctrl Pts',(-13.2563860307187,6.65002775365178,-19.0952152758849));
#18469=CARTESIAN_POINT('Ctrl Pts',(-13.5368119433216,6.65000184997225,-18.7900242993434));
#18470=CARTESIAN_POINT('Ctrl Pts',(-13.5652595935244,6.65001872630134,-18.4999999984663));
#18471=CARTESIAN_POINT('Ctrl Pts',(-13.0396126023806,6.61116933174272,-19.4140223461765));
#18472=CARTESIAN_POINT('Ctrl Pts',(-13.3232070225677,6.63093544404987,-19.2738284330859));
#18473=CARTESIAN_POINT('Ctrl Pts',(-13.6226027377202,6.64873553214766,-18.8824627820465));
#18474=CARTESIAN_POINT('Ctrl Pts',(-13.6962559207404,6.63713438038325,-18.4999999979752));
#18475=CARTESIAN_POINT('Ctrl Pts',(-13.2092320493187,6.44517535101228,-19.7671081794715));
#18476=CARTESIAN_POINT('Ctrl Pts',(-13.4926490904923,6.5329355447166,-19.5234352013649));
#18477=CARTESIAN_POINT('Ctrl Pts',(-13.7989275084018,6.61612657000081,-18.9987393235434));
#18478=CARTESIAN_POINT('Ctrl Pts',(-13.8851496535813,6.57983328116779,-18.499999997364));
#18479=CARTESIAN_POINT('Ctrl Pts',(-13.4604801612314,6.1970778370455,-20.0000694996498));
#18480=CARTESIAN_POINT('Ctrl Pts',(-13.7204167792394,6.35869299291861,-19.700859717038));
#18481=CARTESIAN_POINT('Ctrl Pts',(-14.009795050356,6.52385442234337,-19.0757337060942));
#18482=CARTESIAN_POINT('Ctrl Pts',(-14.0591509646277,6.48682859378864,-18.4999999969598));
#18483=CARTESIAN_POINT('Ctrl Pts',(-13.7542035734046,5.90426917911432,-20.0822650788903));
#18484=CARTESIAN_POINT('Ctrl Pts',(-13.9754027621768,6.12558454016965,-19.7657545358291));
#18485=CARTESIAN_POINT('Ctrl Pts',(-14.214781365486,6.36471268348123,-19.1045289473903));
#18486=CARTESIAN_POINT('Ctrl Pts',(-14.2116652821764,6.36166528217619,-18.4999999968019));
#18487=CARTESIAN_POINT('Ctrl Pts',(-14.0470674075829,5.61021883748008,-20.0001437555208));
#18488=CARTESIAN_POINT('Ctrl Pts',(-14.209895391559,5.87040128717705,-19.6998305081928));
#18489=CARTESIAN_POINT('Ctrl Pts',(-14.3737201797862,6.15993553582587,-19.0761517589312));
#18490=CARTESIAN_POINT('Ctrl Pts',(-14.336828593787,6.20915096462532,-18.499999996955));
#18491=CARTESIAN_POINT('Ctrl Pts',(-14.2951361405339,5.36009661840369,-19.7669964902509));
#18492=CARTESIAN_POINT('Ctrl Pts',(-14.3844114694822,5.64346751311684,-19.5204897565764));
#18493=CARTESIAN_POINT('Ctrl Pts',(-14.4661360608765,5.94912088712555,-18.9989428562545));
#18494=CARTESIAN_POINT('Ctrl Pts',(-14.4298332811648,6.0351496535811,-18.4999999973626));
#18495=CARTESIAN_POINT('Ctrl Pts',(-14.4611328976568,5.18703565679378,-19.4146293224293));
#18496=CARTESIAN_POINT('Ctrl Pts',(-14.482540122838,5.47116307253208,-19.270971688124));
#18497=CARTESIAN_POINT('Ctrl Pts',(-14.4987564117522,5.77187033265161,-18.8811859318062));
#18498=CARTESIAN_POINT('Ctrl Pts',(-14.4871343803804,5.84625592074344,-18.4999999979862));
#18499=CARTESIAN_POINT('Ctrl Pts',(-14.5000565697471,5.14917290265596,-19.1402100483587));
#18500=CARTESIAN_POINT('Ctrl Pts',(-14.5000254205556,5.40884039973222,-19.088420003154));
#18501=CARTESIAN_POINT('Ctrl Pts',(-14.5000018196169,5.6881172092188,-18.7897579239478));
#18502=CARTESIAN_POINT('Ctrl Pts',(-14.5000187262999,5.71525959351538,-18.4999999984668));
#18503=CARTESIAN_POINT('Ctrl Pts',(-14.4999998765826,5.14432072445288,-18.9995579554861));
#18504=CARTESIAN_POINT('Ctrl Pts',(-14.499999944535,5.38684649954523,-18.9943613932106));
#18505=CARTESIAN_POINT('Ctrl Pts',(-14.4999999960227,5.64983329085767,-18.7428715921064));
#18506=CARTESIAN_POINT('Ctrl Pts',(-14.4999999591429,5.64971461892676,-18.4999999987146));
#18507=CARTESIAN_POINT('Ctrl Pts',(-14.5000000000013,-34.6443380969227,
-19.0000100692442));
#18508=CARTESIAN_POINT('Ctrl Pts',(-14.5000000000008,-34.8871059113903,
-19.0015933091084));
#18509=CARTESIAN_POINT('Ctrl Pts',(-14.5000000000027,-35.1500000009281,
-18.7430757267126));
#18510=CARTESIAN_POINT('Ctrl Pts',(-14.5000000000019,-35.15,-18.4999999987137));
#18511=CARTESIAN_POINT('Ctrl Pts',(-14.5000000000028,-34.645317328355,-19.1412652085388));
#18512=CARTESIAN_POINT('Ctrl Pts',(-14.5000000000014,-34.9064831044291,
-19.0954746833564));
#18513=CARTESIAN_POINT('Ctrl Pts',(-14.5000000000026,-35.1869365607809,
-18.7901585471376));
#18514=CARTESIAN_POINT('Ctrl Pts',(-14.5000000000014,-35.215449847102,-18.4999999984638));
#18515=CARTESIAN_POINT('Ctrl Pts',(-14.461088950263,-34.6896947394679,-19.4141933256417));
#18516=CARTESIAN_POINT('Ctrl Pts',(-14.4808879882492,-34.9732890737612,
-19.2739493035027));
#18517=CARTESIAN_POINT('Ctrl Pts',(-14.4987197414757,-35.272688121818,-18.8825190881865));
#18518=CARTESIAN_POINT('Ctrl Pts',(-14.4871066327079,-35.3463473912737,
-18.4999999979725));
#18519=CARTESIAN_POINT('Ctrl Pts',(-14.2951753510104,-34.8592320493177,
-19.7671081794723));
#18520=CARTESIAN_POINT('Ctrl Pts',(-14.3829355447186,-35.1426490904922,
-19.5234352013656));
#18521=CARTESIAN_POINT('Ctrl Pts',(-14.466126570005,-35.448927508403,-18.9987393235418));
#18522=CARTESIAN_POINT('Ctrl Pts',(-14.4298332811675,-35.5351496535818,
-18.4999999973609));
#18523=CARTESIAN_POINT('Ctrl Pts',(-14.0470778370451,-35.1104801612305,
-20.0000694996508));
#18524=CARTESIAN_POINT('Ctrl Pts',(-14.208692992919,-35.3704167792393,-19.7008597170388));
#18525=CARTESIAN_POINT('Ctrl Pts',(-14.373854422343,-35.6597950503571,-19.0757337060923));
#18526=CARTESIAN_POINT('Ctrl Pts',(-14.3368285937893,-35.709150964628,-18.4999999969561));
#18527=CARTESIAN_POINT('Ctrl Pts',(-13.7542691791144,-35.4042035734038,
-20.0822650788914));
#18528=CARTESIAN_POINT('Ctrl Pts',(-13.9755845401677,-35.6254027621767,
-19.7657545358299));
#18529=CARTESIAN_POINT('Ctrl Pts',(-14.2147126834794,-35.864781365487,-19.1045289473882));
#18530=CARTESIAN_POINT('Ctrl Pts',(-14.2116652821725,-35.8616652821764,
-18.4999999967981));
#18531=CARTESIAN_POINT('Ctrl Pts',(-13.4602188374819,-35.6970674075824,
-20.0001437555219));
#18532=CARTESIAN_POINT('Ctrl Pts',(-13.7204012871743,-35.859895391559,-19.6998305081936));
#18533=CARTESIAN_POINT('Ctrl Pts',(-14.0099355358227,-36.023720179787,-19.0761517589292));
#18534=CARTESIAN_POINT('Ctrl Pts',(-14.0591509646221,-35.9868285937868,
-18.4999999969514));
#18535=CARTESIAN_POINT('Ctrl Pts',(-13.2100966184005,-35.9451361405336,
-19.7669964902518));
#18536=CARTESIAN_POINT('Ctrl Pts',(-13.4934675131165,-36.0344114694822,
-19.5204897565771));
#18537=CARTESIAN_POINT('Ctrl Pts',(-13.7991208871267,-36.1161360608768,
-18.9989428562529));
#18538=CARTESIAN_POINT('Ctrl Pts',(-13.8851496535816,-36.0798332811645,
-18.4999999973594));
#18539=CARTESIAN_POINT('Ctrl Pts',(-13.0371194604123,-36.1110525148315,
-19.4147999538865));
#18540=CARTESIAN_POINT('Ctrl Pts',(-13.3212465098146,-36.1324926046905,
-19.2710925155892));
#18541=CARTESIAN_POINT('Ctrl Pts',(-13.6219561650579,-36.1487406155644,
-18.8812429548123));
#18542=CARTESIAN_POINT('Ctrl Pts',(-13.6963473912789,-36.1371066327043,
-18.4999999979835));
#18543=CARTESIAN_POINT('Ctrl Pts',(-12.9992279345901,-36.1500000000002,
-19.1406085881773));
#18544=CARTESIAN_POINT('Ctrl Pts',(-13.2589309435621,-36.1500000000008,
-19.0886851287514));
#18545=CARTESIAN_POINT('Ctrl Pts',(-13.5382388686105,-36.1499999999992,
-18.7898907052044));
#18546=CARTESIAN_POINT('Ctrl Pts',(-13.5654498470941,-36.1499999999989,
-18.4999999984642));
#18547=CARTESIAN_POINT('Ctrl Pts',(-12.9943419397749,-36.1500000000006,
-19.0001703298077));
#18548=CARTESIAN_POINT('Ctrl Pts',(-13.2369423184852,-36.1500000000009,
-18.9947709047232));
#18549=CARTESIAN_POINT('Ctrl Pts',(-13.5000000009278,-36.1499999999995,
-18.7430757267406));
#18550=CARTESIAN_POINT('Ctrl Pts',(-13.4999999999998,-36.1499999999986,
-18.499999998712));
#18551=CARTESIAN_POINT('Ctrl Pts',(-8.14999999999987,-40.9943380969236,
-19.0000100692442));
#18552=CARTESIAN_POINT('Ctrl Pts',(-8.1500000000003,-41.237105911391,-19.0015933091078));
#18553=CARTESIAN_POINT('Ctrl Pts',(-8.15000000000033,-41.5000000009281,
-18.7430757267123));
#18554=CARTESIAN_POINT('Ctrl Pts',(-8.15000000000025,-41.5,-18.4999999987137));
#18555=CARTESIAN_POINT('Ctrl Pts',(-8.15000000000028,-40.9953173283559,
-19.1412652085387));
#18556=CARTESIAN_POINT('Ctrl Pts',(-8.15000000000049,-41.2564831044297,
-19.0954746833557));
#18557=CARTESIAN_POINT('Ctrl Pts',(-8.15000000000039,-41.536936560781,-18.7901585471373));
#18558=CARTESIAN_POINT('Ctrl Pts',(-8.15000000000039,-41.565449847102,-18.4999999984638));
#18559=CARTESIAN_POINT('Ctrl Pts',(-8.11108895026239,-41.0396947394688,
-19.4141933256412));
#18560=CARTESIAN_POINT('Ctrl Pts',(-8.13088798825094,-41.3232890737619,
-19.2739493035018));
#18561=CARTESIAN_POINT('Ctrl Pts',(-8.14871974147486,-41.6226881218181,
-18.8825190881861));
#18562=CARTESIAN_POINT('Ctrl Pts',(-8.13710663270727,-41.6963473912737,
-18.4999999979725));
#18563=CARTESIAN_POINT('Ctrl Pts',(-7.94517535101228,-41.2092320493187,
-19.7671081794715));
#18564=CARTESIAN_POINT('Ctrl Pts',(-8.03293554471679,-41.4926490904929,
-19.5234352013644));
#18565=CARTESIAN_POINT('Ctrl Pts',(-8.11612657000116,-41.7989275084031,
-18.9987393235412));
#18566=CARTESIAN_POINT('Ctrl Pts',(-8.07983328116756,-41.8851496535818,
-18.4999999973609));
#18567=CARTESIAN_POINT('Ctrl Pts',(-7.69707783704551,-41.4604801612314,
-20.0000694996498));
#18568=CARTESIAN_POINT('Ctrl Pts',(-7.85869299291896,-41.72041677924,-19.7008597170374));
#18569=CARTESIAN_POINT('Ctrl Pts',(-8.02385442234407,-42.0097950503572,
-19.0757337060916));
#18570=CARTESIAN_POINT('Ctrl Pts',(-7.98682859378841,-42.059150964628,-18.4999999969561));
#18571=CARTESIAN_POINT('Ctrl Pts',(-7.40426917911432,-41.7542035734046,
-20.0822650788903));
#18572=CARTESIAN_POINT('Ctrl Pts',(-7.62558454017011,-41.9754027621772,
-19.7657545358284));
#18573=CARTESIAN_POINT('Ctrl Pts',(-7.86471268348223,-42.214781365487,-19.1045289473875));
#18574=CARTESIAN_POINT('Ctrl Pts',(-7.86166528217617,-42.2116652821764,
-18.4999999967981));
#18575=CARTESIAN_POINT('Ctrl Pts',(-7.11021883748008,-42.0470674075829,
-20.0001437555208));
#18576=CARTESIAN_POINT('Ctrl Pts',(-7.3704012871776,-42.2098953915593,-19.6998305081922));
#18577=CARTESIAN_POINT('Ctrl Pts',(-7.65993553582709,-42.3737201797869,
-19.0761517589285));
#18578=CARTESIAN_POINT('Ctrl Pts',(-7.70915096462563,-42.3368285937868,
-18.4999999969514));
#18579=CARTESIAN_POINT('Ctrl Pts',(-6.86009661840369,-42.2951361405338,
-19.7669964902509));
#18580=CARTESIAN_POINT('Ctrl Pts',(-7.14346751311743,-42.3844114694824,
-19.5204897565759));
#18581=CARTESIAN_POINT('Ctrl Pts',(-7.44912088712684,-42.4661360608768,
-18.9989428562523));
#18582=CARTESIAN_POINT('Ctrl Pts',(-7.53514965358164,-42.4298332811645,
-18.4999999973594));
#18583=CARTESIAN_POINT('Ctrl Pts',(-6.68711946041285,-42.4610525148318,
-19.4147999538856));
#18584=CARTESIAN_POINT('Ctrl Pts',(-6.97124650981146,-42.4824926046906,
-19.271092515588));
#18585=CARTESIAN_POINT('Ctrl Pts',(-7.2719561650544,-42.4987406155645,-18.8812429548117));
#18586=CARTESIAN_POINT('Ctrl Pts',(-7.34634739127708,-42.4871066327043,
-18.4999999979835));
#18587=CARTESIAN_POINT('Ctrl Pts',(-6.64922793459199,-42.5000000000004,
-19.1406085881762));
#18588=CARTESIAN_POINT('Ctrl Pts',(-6.90893094356097,-42.5000000000009,
-19.0886851287501));
#18589=CARTESIAN_POINT('Ctrl Pts',(-7.1882388686094,-42.4999999999992,-18.7898907052038));
#18590=CARTESIAN_POINT('Ctrl Pts',(-7.21544984709361,-42.4999999999989,
-18.4999999984642));
#18591=CARTESIAN_POINT('Ctrl Pts',(-6.64434193977743,-42.5000000000005,
-19.0001703298062));
#18592=CARTESIAN_POINT('Ctrl Pts',(-6.88694231848536,-42.5000000000009,
-18.9947709047217));
#18593=CARTESIAN_POINT('Ctrl Pts',(-7.15000000092837,-42.4999999999995,
-18.7430757267398));
#18594=CARTESIAN_POINT('Ctrl Pts',(-7.15,-42.4999999999986,-18.499999998712));
#18595=CARTESIAN_POINT('Ctrl Pts',(6.64433396160519,-42.499999876699,-18.9993941238985));
#18596=CARTESIAN_POINT('Ctrl Pts',(6.88702150988135,-42.4999999394466,-19.001183928576));
#18597=CARTESIAN_POINT('Ctrl Pts',(7.14983898402066,-42.4999999959597,-18.74287042571));
#18598=CARTESIAN_POINT('Ctrl Pts',(7.14971461892777,-42.4999999591463,-18.4999999987164));
#18599=CARTESIAN_POINT('Ctrl Pts',(6.6452528649791,-42.5000565167741,-19.140868505694));
#18600=CARTESIAN_POINT('Ctrl Pts',(6.90638603072031,-42.5000277536524,-19.095215275888));
#18601=CARTESIAN_POINT('Ctrl Pts',(7.1868119433205,-42.5000018499744,-18.7900242993449));
#18602=CARTESIAN_POINT('Ctrl Pts',(7.2152595935232,-42.5000187263022,-18.4999999984663));
#18603=CARTESIAN_POINT('Ctrl Pts',(6.68961260237979,-42.4611693317427,-19.4140223461786));
#18604=CARTESIAN_POINT('Ctrl Pts',(6.97320702256912,-42.4809354440478,-19.2738284330882));
#18605=CARTESIAN_POINT('Ctrl Pts',(7.27260273771983,-42.4987355321484,-18.8824627820476));
#18606=CARTESIAN_POINT('Ctrl Pts',(7.34625592074007,-42.4871343803837,-18.4999999979752));
#18607=CARTESIAN_POINT('Ctrl Pts',(6.85923204931696,-42.2951753510103,-19.7671081794728));
#18608=CARTESIAN_POINT('Ctrl Pts',(7.14264909049096,-42.3829355447183,-19.5234352013668));
#18609=CARTESIAN_POINT('Ctrl Pts',(7.44892750840371,-42.4661265700047,-18.9987393235443));
#18610=CARTESIAN_POINT('Ctrl Pts',(7.53514965358202,-42.4298332811677,-18.499999997364));
#18611=CARTESIAN_POINT('Ctrl Pts',(7.11048016122898,-42.0470778370448,-20.0000694996515));
#18612=CARTESIAN_POINT('Ctrl Pts',(7.37041677923766,-42.2086929929184,-19.7008597170403));
#18613=CARTESIAN_POINT('Ctrl Pts',(7.65979505035629,-42.3738544223423,-19.0757337060953));
#18614=CARTESIAN_POINT('Ctrl Pts',(7.70915096462646,-42.3368285937896,-18.4999999969597));
#18615=CARTESIAN_POINT('Ctrl Pts',(7.4042035734027,-41.754269179114,-20.0822650788921));
#18616=CARTESIAN_POINT('Ctrl Pts',(7.62540276217399,-41.9755845401669,-19.7657545358315));
#18617=CARTESIAN_POINT('Ctrl Pts',(7.86478136548691,-42.2147126834784,-19.1045289473914));
#18618=CARTESIAN_POINT('Ctrl Pts',(7.86166528217616,-42.2116652821725,-18.4999999968019));
#18619=CARTESIAN_POINT('Ctrl Pts',(7.69706740757966,-41.4602188374814,-20.0001437555225));
#18620=CARTESIAN_POINT('Ctrl Pts',(7.85989539155775,-41.7204012871734,-19.6998305081951));
#18621=CARTESIAN_POINT('Ctrl Pts',(8.02372017978781,-42.0099355358214,-19.0761517589322));
#18622=CARTESIAN_POINT('Ctrl Pts',(7.98682859378959,-42.0591509646218,-18.499999996955));
#18623=CARTESIAN_POINT('Ctrl Pts',(7.94513614053531,-41.2100966184,-19.7669964902523));
#18624=CARTESIAN_POINT('Ctrl Pts',(8.0344114694836,-41.4934675131155,-19.5204897565783));
#18625=CARTESIAN_POINT('Ctrl Pts',(8.11613606087722,-41.7991208871254,-18.9989428562554));
#18626=CARTESIAN_POINT('Ctrl Pts',(8.07983328116767,-41.8851496535811,-18.4999999973625));
#18627=CARTESIAN_POINT('Ctrl Pts',(8.11113289765597,-41.037035656793,-19.4146293224311));
#18628=CARTESIAN_POINT('Ctrl Pts',(8.13254012283828,-41.3211630725351,-19.2709716881261));
#18629=CARTESIAN_POINT('Ctrl Pts',(8.14875641175435,-41.6218703326553,-18.8811859318073));
#18630=CARTESIAN_POINT('Ctrl Pts',(8.13713438038314,-41.6962559207456,-18.4999999979862));
#18631=CARTESIAN_POINT('Ctrl Pts',(8.15005656974628,-40.9991729026537,-19.1402100483613));
#18632=CARTESIAN_POINT('Ctrl Pts',(8.15002542055481,-41.2588403997333,-19.0884200031566));
#18633=CARTESIAN_POINT('Ctrl Pts',(8.15000181961798,-41.5381172092203,-18.7897579239491));
#18634=CARTESIAN_POINT('Ctrl Pts',(8.15001872630097,-41.5652595935165,-18.4999999984667));
#18635=CARTESIAN_POINT('Ctrl Pts',(8.14999987658211,-40.9943207244499,-18.9995579554898));
#18636=CARTESIAN_POINT('Ctrl Pts',(8.14999994453439,-41.2368464995451,-18.994361393214));
#18637=CARTESIAN_POINT('Ctrl Pts',(8.14999999602334,-41.4998332908577,-18.742871592108));
#18638=CARTESIAN_POINT('Ctrl Pts',(8.14999995914438,-41.4997146189276,-18.4999999987146));
#18639=CARTESIAN_POINT('Ctrl Pts',(12.9943339616049,-36.149999876699,-18.9993941238957));
#18640=CARTESIAN_POINT('Ctrl Pts',(13.2370215098809,-36.1499999394466,-19.001183928573));
#18641=CARTESIAN_POINT('Ctrl Pts',(13.4998389840216,-36.1499999959597,-18.7428704257086));
#18642=CARTESIAN_POINT('Ctrl Pts',(13.4997146189285,-36.1499999591463,-18.4999999987164));
#18643=CARTESIAN_POINT('Ctrl Pts',(12.9952528649788,-36.1500565167744,-19.1408685056919));
#18644=CARTESIAN_POINT('Ctrl Pts',(13.2563860307191,-36.1500277536526,-19.0952152758855));
#18645=CARTESIAN_POINT('Ctrl Pts',(13.536811943322,-36.1500018499744,-18.7900242993437));
#18646=CARTESIAN_POINT('Ctrl Pts',(13.5652595935249,-36.1500187263023,-18.4999999984663));
#18647=CARTESIAN_POINT('Ctrl Pts',(13.039612602381,-36.1111693317432,-19.4140223461769));
#18648=CARTESIAN_POINT('Ctrl Pts',(13.3232070225681,-36.1309354440481,-19.2738284330861));
#18649=CARTESIAN_POINT('Ctrl Pts',(13.6226027377205,-36.1487355321485,-18.8824627820465));
#18650=CARTESIAN_POINT('Ctrl Pts',(13.6962559207406,-36.1371343803838,-18.4999999979752));
#18651=CARTESIAN_POINT('Ctrl Pts',(13.2092320493188,-35.9451753510108,-19.7671081794713));
#18652=CARTESIAN_POINT('Ctrl Pts',(13.4926490904924,-36.0329355447186,-19.5234352013647));
#18653=CARTESIAN_POINT('Ctrl Pts',(13.7989275084019,-36.1161265700046,-18.9987393235433));
#18654=CARTESIAN_POINT('Ctrl Pts',(13.8851496535813,-36.0798332811677,-18.499999997364));
#18655=CARTESIAN_POINT('Ctrl Pts',(13.4604801612315,-35.6970778370458,-20.0000694996497));
#18656=CARTESIAN_POINT('Ctrl Pts',(13.7204167792395,-35.8586929929191,-19.7008597170378));
#18657=CARTESIAN_POINT('Ctrl Pts',(14.009795050356,-36.0238544223422,-19.0757337060941));
#18658=CARTESIAN_POINT('Ctrl Pts',(14.0591509646277,-35.9868285937896,-18.4999999969598));
#18659=CARTESIAN_POINT('Ctrl Pts',(13.7542035734047,-35.4042691791153,-20.0822650788901));
#18660=CARTESIAN_POINT('Ctrl Pts',(13.9754027621768,-35.6255845401679,-19.7657545358289));
#18661=CARTESIAN_POINT('Ctrl Pts',(14.214781365486,-35.8647126834784,-19.1045289473902));
#18662=CARTESIAN_POINT('Ctrl Pts',(14.2116652821764,-35.8616652821725,-18.4999999968019));
#18663=CARTESIAN_POINT('Ctrl Pts',(14.047067407583,-35.1102188374757,-20.0001437555207));
#18664=CARTESIAN_POINT('Ctrl Pts',(14.209895391559,-35.3704012871737,-19.6998305081926));
#18665=CARTESIAN_POINT('Ctrl Pts',(14.3737201797862,-35.6599355358214,-19.0761517589311));
#18666=CARTESIAN_POINT('Ctrl Pts',(14.336828593787,-35.7091509646218,-18.499999996955));
#18667=CARTESIAN_POINT('Ctrl Pts',(14.2951361405339,-34.8600966184017,-19.7669964902508));
#18668=CARTESIAN_POINT('Ctrl Pts',(14.3844114694822,-35.1434675131167,-19.5204897565762));
#18669=CARTESIAN_POINT('Ctrl Pts',(14.4661360608765,-35.4491208871255,-18.9989428562544));
#18670=CARTESIAN_POINT('Ctrl Pts',(14.4298332811648,-35.5351496535811,-18.4999999973626));
#18671=CARTESIAN_POINT('Ctrl Pts',(14.4611328976566,-34.6870356567945,-19.4146293224298));
#18672=CARTESIAN_POINT('Ctrl Pts',(14.4825401228378,-34.9711630725361,-19.2709716881243));
#18673=CARTESIAN_POINT('Ctrl Pts',(14.4987564117522,-35.2718703326553,-18.8811859318064));
#18674=CARTESIAN_POINT('Ctrl Pts',(14.4871343803803,-35.3462559207454,-18.4999999979862));
#18675=CARTESIAN_POINT('Ctrl Pts',(14.5000565697469,-34.6491729026552,-19.1402100483601));
#18676=CARTESIAN_POINT('Ctrl Pts',(14.5000254205555,-34.9088403997342,-19.0884200031548));
#18677=CARTESIAN_POINT('Ctrl Pts',(14.5000018196169,-35.1881172092201,-18.7897579239482));
#18678=CARTESIAN_POINT('Ctrl Pts',(14.5000187262999,-35.2152595935161,-18.4999999984667));
#18679=CARTESIAN_POINT('Ctrl Pts',(14.4999998765827,-34.6443207244513,-18.9995579554883));
#18680=CARTESIAN_POINT('Ctrl Pts',(14.499999944535,-34.8868464995459,-18.9943613932121));
#18681=CARTESIAN_POINT('Ctrl Pts',(14.4999999960227,-35.1498332908573,-18.7428715921071));
#18682=CARTESIAN_POINT('Ctrl Pts',(14.499999959143,-35.149714618927,-18.4999999987146));
#18683=CARTESIAN_POINT('Ctrl Pts',(14.5000000000013,5.14433809692412,-19.0000100692486));
#18684=CARTESIAN_POINT('Ctrl Pts',(14.5000000000008,5.38710591139172,-19.0015933091117));
#18685=CARTESIAN_POINT('Ctrl Pts',(14.5000000000027,5.65000000092752,-18.7430757267142));
#18686=CARTESIAN_POINT('Ctrl Pts',(14.5000000000019,5.65,-18.4999999987137));
#18687=CARTESIAN_POINT('Ctrl Pts',(14.5000000000024,5.14531732835656,-19.1412652085418));
#18688=CARTESIAN_POINT('Ctrl Pts',(14.5000000000012,5.40648310443134,-19.0954746833587));
#18689=CARTESIAN_POINT('Ctrl Pts',(14.5000000000026,5.6869365607798,-18.7901585471388));
#18690=CARTESIAN_POINT('Ctrl Pts',(14.5000000000012,5.71544984710073,-18.4999999984638));
#18691=CARTESIAN_POINT('Ctrl Pts',(14.4610889502624,5.18969473946802,-19.4141933256432));
#18692=CARTESIAN_POINT('Ctrl Pts',(14.4808879882489,5.47328907376343,-19.2739493035041));
#18693=CARTESIAN_POINT('Ctrl Pts',(14.4987197414756,5.77268812181769,-18.8825190881872));
#18694=CARTESIAN_POINT('Ctrl Pts',(14.4871066327078,5.84634739127338,-18.4999999979725));
#18695=CARTESIAN_POINT('Ctrl Pts',(14.2951753510102,5.3592320493172,-19.7671081794728));
#18696=CARTESIAN_POINT('Ctrl Pts',(14.3829355447185,5.64264909049228,-19.5234352013663));
#18697=CARTESIAN_POINT('Ctrl Pts',(14.4661265700051,5.94892750840517,-18.9987393235421));
#18698=CARTESIAN_POINT('Ctrl Pts',(14.4298332811675,6.03514965358259,-18.4999999973609));
#18699=CARTESIAN_POINT('Ctrl Pts',(14.0470778370448,5.61048016122898,-20.0000694996515));
#18700=CARTESIAN_POINT('Ctrl Pts',(14.2086929929188,5.8704167792382,-19.7008597170397));
#18701=CARTESIAN_POINT('Ctrl Pts',(14.373854422343,6.15979505035749,-19.0757337060927));
#18702=CARTESIAN_POINT('Ctrl Pts',(14.3368285937893,6.20915096462677,-18.4999999969561));
#18703=CARTESIAN_POINT('Ctrl Pts',(13.754269179114,5.90420357340269,-20.0822650788921));
#18704=CARTESIAN_POINT('Ctrl Pts',(13.9755845401674,6.12540276217445,-19.7657545358308));
#18705=CARTESIAN_POINT('Ctrl Pts',(14.2147126834794,6.36478136548791,-19.1045289473886));
#18706=CARTESIAN_POINT('Ctrl Pts',(14.2116652821725,6.36166528217614,-18.4999999967981));
#18707=CARTESIAN_POINT('Ctrl Pts',(13.4602188374814,6.19706740757966,-20.0001437555225));
#18708=CARTESIAN_POINT('Ctrl Pts',(13.7204012871739,6.35989539155808,-19.6998305081945));
#18709=CARTESIAN_POINT('Ctrl Pts',(14.0099355358226,6.52372017978849,-19.0761517589296));
#18710=CARTESIAN_POINT('Ctrl Pts',(14.0591509646221,6.48682859378936,-18.4999999969514));
#18711=CARTESIAN_POINT('Ctrl Pts',(13.2100966183999,6.44513614053531,-19.7669964902523));
#18712=CARTESIAN_POINT('Ctrl Pts',(13.493467513116,6.53441146948378,-19.5204897565778));
#18713=CARTESIAN_POINT('Ctrl Pts',(13.7991208871266,6.61613606087756,-18.9989428562532));
#18714=CARTESIAN_POINT('Ctrl Pts',(13.8851496535816,6.57983328116744,-18.4999999973594));
#18715=CARTESIAN_POINT('Ctrl Pts',(13.0371194604117,6.61105251483121,-19.4147999538868));
#18716=CARTESIAN_POINT('Ctrl Pts',(13.3212465098142,6.63249260469108,-19.2710925155897));
#18717=CARTESIAN_POINT('Ctrl Pts',(13.6219561650578,6.64874061556663,-18.8812429548125));
#18718=CARTESIAN_POINT('Ctrl Pts',(13.6963473912789,6.63710663270717,-18.4999999979835));
#18719=CARTESIAN_POINT('Ctrl Pts',(12.9992279345896,6.64999999999977,-19.1406085881775));
#18720=CARTESIAN_POINT('Ctrl Pts',(13.2589309435617,6.65000000000017,-19.0886851287518));
#18721=CARTESIAN_POINT('Ctrl Pts',(13.5382388686105,6.65000000000027,-18.7898907052046));
#18722=CARTESIAN_POINT('Ctrl Pts',(13.5654498470941,6.65000000000003,-18.4999999984642));
#18723=CARTESIAN_POINT('Ctrl Pts',(12.9943419397744,6.64999999999998,-19.0001703298077));
#18724=CARTESIAN_POINT('Ctrl Pts',(13.2369423184849,6.65000000000029,-18.9947709047236));
#18725=CARTESIAN_POINT('Ctrl Pts',(13.5000000009278,6.65000000000017,-18.7430757267408));
#18726=CARTESIAN_POINT('Ctrl Pts',(13.4999999999998,6.65000000000004,-18.499999998712));
#18727=CARTESIAN_POINT('Origin',(13.98,-23.05,-5.));
#18728=CARTESIAN_POINT('',(13.98,-37.95,-4.1));
#18729=CARTESIAN_POINT('',(13.98,-23.05,-4.1));
#18730=CARTESIAN_POINT('',(13.98,-23.05,-4.1));
#18731=CARTESIAN_POINT('',(13.98,-23.05,-5.));
#18732=CARTESIAN_POINT('',(13.98,-37.95,-5.));
#18733=CARTESIAN_POINT('Origin',(18.88,-23.05,-5.));
#18734=CARTESIAN_POINT('',(18.88,-23.05,-4.1));
#18735=CARTESIAN_POINT('',(18.88,-23.05,-4.1));
#18736=CARTESIAN_POINT('',(18.88,-23.05,-5.));
#18737=CARTESIAN_POINT('Origin',(18.88,-37.95,-5.));
#18738=CARTESIAN_POINT('',(18.88,-37.95,-4.1));
#18739=CARTESIAN_POINT('',(18.88,-37.95,-4.1));
#18740=CARTESIAN_POINT('',(18.88,-37.95,-5.));
#18741=CARTESIAN_POINT('Origin',(13.98,-37.95,-5.));
#18742=CARTESIAN_POINT('',(13.98,-37.95,-4.1));
#18743=CARTESIAN_POINT('Origin',(0.,0.,28.));
#18744=CARTESIAN_POINT('Origin',(0.,0.,-4.1));
#18745=CARTESIAN_POINT('Origin',(0.,0.,-19.8));
#18746=CARTESIAN_POINT('Origin',(0.,0.,-4.1));
#18747=CARTESIAN_POINT('Origin',(0.,0.,-21.));
#18748=CARTESIAN_POINT('Origin',(0.,0.,-23.5));
#18749=CARTESIAN_POINT('Origin',(0.,0.,-24.3));
#18750=CARTESIAN_POINT('Origin',(0.,0.,-26.1));
#20147=UNCERTAINTY_MEASURE_WITH_UNIT(LENGTH_MEASURE(0.01),#20177,
'DISTANCE_ACCURACY_VALUE',
'Maximum model space distance between geometric entities at asserted c
onnectivities');
#20160=UNCERTAINTY_MEASURE_WITH_UNIT(LENGTH_MEASURE(0.01),#20177,
'DISTANCE_ACCURACY_VALUE',
'Maximum model space distance between geometric entities at asserted c
onnectivities');
#20163=(
GEOMETRIC_REPRESENTATION_CONTEXT(3)
GLOBAL_UNCERTAINTY_ASSIGNED_CONTEXT((#20147))
GLOBAL_UNIT_ASSIGNED_CONTEXT((#20177,#20179,#20180))
REPRESENTATION_CONTEXT('','3D')
);
#20176=(
GEOMETRIC_REPRESENTATION_CONTEXT(3)
GLOBAL_UNCERTAINTY_ASSIGNED_CONTEXT((#20160))
GLOBAL_UNIT_ASSIGNED_CONTEXT((#20177,#20179,#20180))
REPRESENTATION_CONTEXT('','3D')
);
#20177=(
LENGTH_UNIT()
NAMED_UNIT(*)
SI_UNIT(.MILLI.,.METRE.)
);
#20179=(
NAMED_UNIT(*)
PLANE_ANGLE_UNIT()
SI_UNIT($,.RADIAN.)
);
#20180=(
NAMED_UNIT(*)
SI_UNIT($,.STERADIAN.)
SOLID_ANGLE_UNIT()
);
#20183=SHAPE_DEFINITION_REPRESENTATION(#20198,#20257);
#20198=PRODUCT_DEFINITION_SHAPE('',$,#20273);
#20257=SHAPE_REPRESENTATION('',(#11215),#20163);
#20270=PRODUCT_DEFINITION_CONTEXT('part definition',#20317,'design');
#20273=PRODUCT_DEFINITION('Servo Motor','Servo Motor',#20288,#20270);
#20288=PRODUCT_DEFINITION_FORMATION('',$,#20321);
#20317=APPLICATION_CONTEXT(
'Core Data for Automotive Mechanical Design Process');
#20318=PRODUCT_CONTEXT('part definition',#20317,'mechanical');
#20321=PRODUCT('Servo Motor','Servo Motor',$,(#20318));
#20336=PRESENTATION_STYLE_ASSIGNMENT((#20341));
#20341=SURFACE_STYLE_USAGE(.BOTH.,#20346);
#20346=SURFACE_SIDE_STYLE('',(#20351));
#20351=SURFACE_STYLE_FILL_AREA(#20356);
#20356=FILL_AREA_STYLE('Opaque(97,158,199)',(#20361));
#20361=FILL_AREA_STYLE_COLOUR('Opaque(97,158,199)',#20366);
#20366=COLOUR_RGB('Opaque(97,158,199)',0.380392156862745,0.619607843137255,
0.780392156862745);
ENDSEC;
END-ISO-10303-21;
